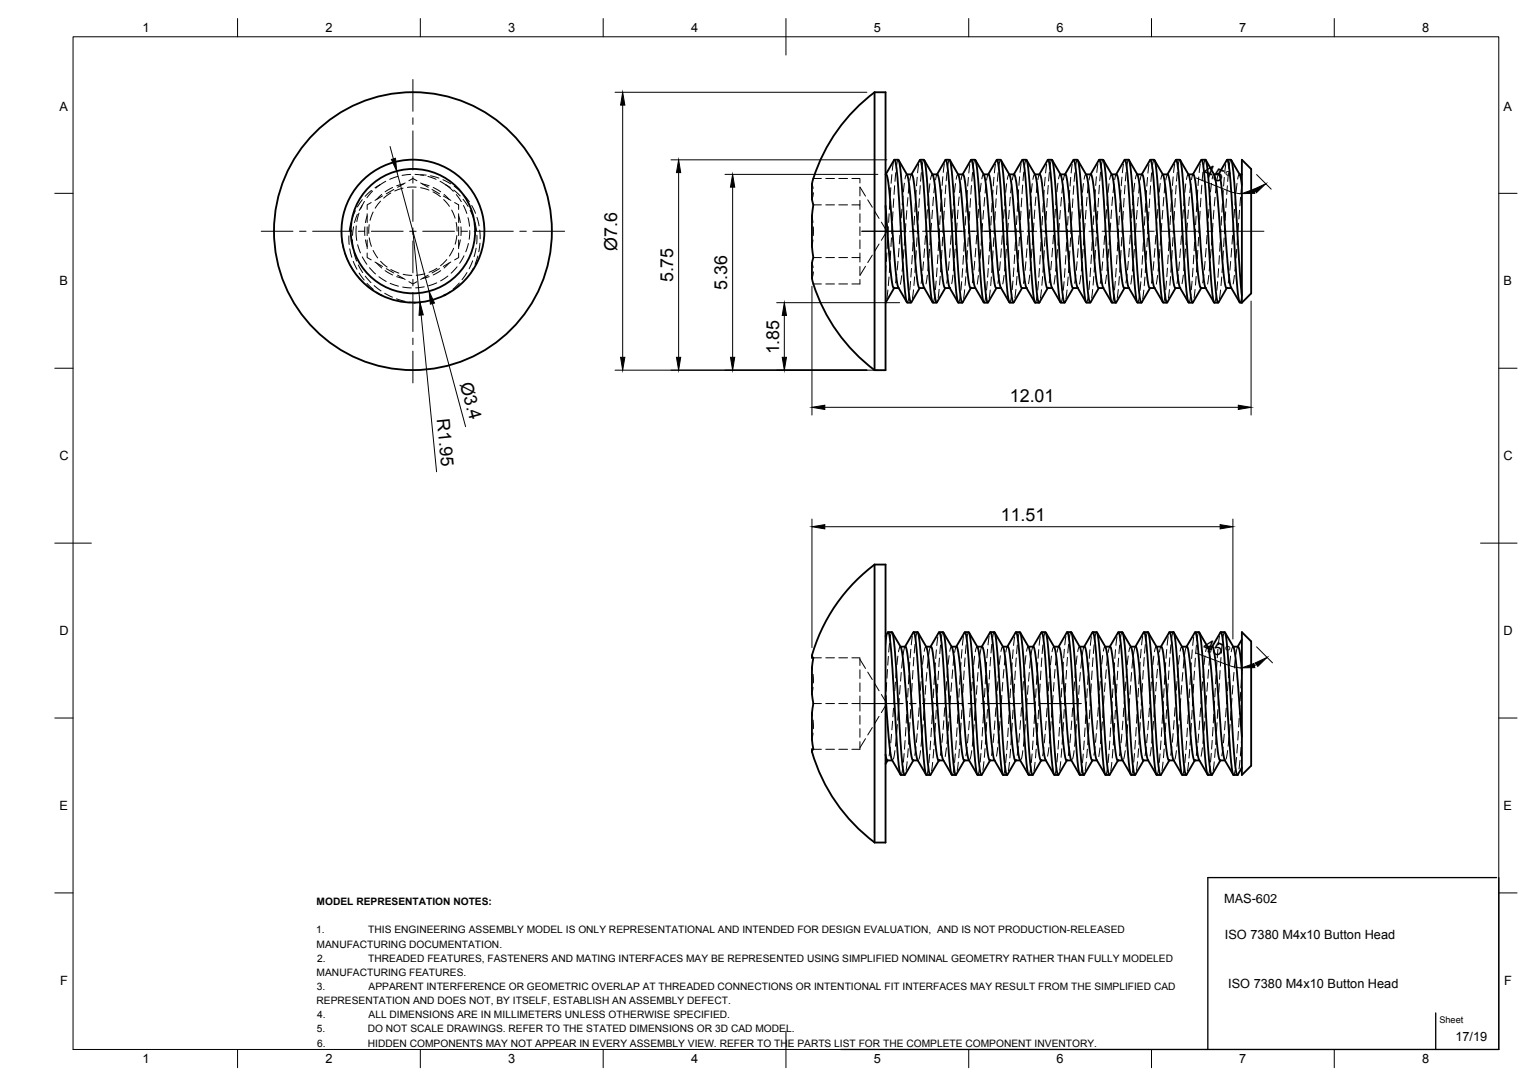
ISO-10303-21;
HEADER;
/* Generated by software containing ST-Developer
 * from STEP Tools, Inc. (www.steptools.com) 
 */

FILE_DESCRIPTION(
/* description */ (''),
/* implementation_level */ '2;1');

FILE_NAME(
/* name */ 'ISO 7380 M4x10 Button Head.step',
/* time_stamp */ '2026-10-15T14:42:47-07:00',
/* author */ (''),
/* organization */ (''),
/* preprocessor_version */ 'ST-DEVELOPER v20.2',
/* originating_system */ 'Autodesk Translation Framework v15.15.0.0',
/* authorisation */ '');

FILE_SCHEMA (('AUTOMOTIVE_DESIGN { 1 0 10303 214 3 1 1 }'));
ENDSEC;

DATA;
#10=MECHANICAL_DESIGN_GEOMETRIC_PRESENTATION_REPRESENTATION('',(#249),#85789);
#147=(
BOUNDED_CURVE()
B_SPLINE_CURVE(2,(#85443,#85444,#85445),.UNSPECIFIED.,.F.,.F.)
B_SPLINE_CURVE_WITH_KNOTS((3,3),(0.00911071066679689,0.0953350369275265),
 .UNSPECIFIED.)
CURVE()
GEOMETRIC_REPRESENTATION_ITEM()
RATIONAL_B_SPLINE_CURVE((1.01317087172823,1.0695397444443,1.01317087172823))
REPRESENTATION_ITEM('')
);
#148=(
BOUNDED_CURVE()
B_SPLINE_CURVE(2,(#85450,#85451,#85452),.UNSPECIFIED.,.F.,.F.)
B_SPLINE_CURVE_WITH_KNOTS((3,3),(0.00911071066679641,0.0953350369275264),
 .UNSPECIFIED.)
CURVE()
GEOMETRIC_REPRESENTATION_ITEM()
RATIONAL_B_SPLINE_CURVE((1.01317087172823,1.06953974444431,1.01317087172823))
REPRESENTATION_ITEM('')
);
#149=(
BOUNDED_CURVE()
B_SPLINE_CURVE(2,(#85457,#85458,#85459),.UNSPECIFIED.,.F.,.F.)
B_SPLINE_CURVE_WITH_KNOTS((3,3),(0.00911071066679675,0.0953350369275265),
 .UNSPECIFIED.)
CURVE()
GEOMETRIC_REPRESENTATION_ITEM()
RATIONAL_B_SPLINE_CURVE((1.01317087172823,1.0695397444443,1.01317087172823))
REPRESENTATION_ITEM('')
);
#150=(
BOUNDED_CURVE()
B_SPLINE_CURVE(2,(#85464,#85465,#85466),.UNSPECIFIED.,.F.,.F.)
B_SPLINE_CURVE_WITH_KNOTS((3,3),(0.00911071066679614,0.0953350369275257),
 .UNSPECIFIED.)
CURVE()
GEOMETRIC_REPRESENTATION_ITEM()
RATIONAL_B_SPLINE_CURVE((1.01317087172823,1.0695397444443,1.01317087172823))
REPRESENTATION_ITEM('')
);
#151=(
BOUNDED_CURVE()
B_SPLINE_CURVE(2,(#85471,#85472,#85473),.UNSPECIFIED.,.F.,.F.)
B_SPLINE_CURVE_WITH_KNOTS((3,3),(0.0091107106667967,0.0953350369275265),
 .UNSPECIFIED.)
CURVE()
GEOMETRIC_REPRESENTATION_ITEM()
RATIONAL_B_SPLINE_CURVE((1.01317087172823,1.0695397444443,1.01317087172823))
REPRESENTATION_ITEM('')
);
#152=(
BOUNDED_CURVE()
B_SPLINE_CURVE(2,(#85480,#85481,#85482),.UNSPECIFIED.,.F.,.F.)
B_SPLINE_CURVE_WITH_KNOTS((3,3),(0.00911071066679617,0.0953350369275259),
 .UNSPECIFIED.)
CURVE()
GEOMETRIC_REPRESENTATION_ITEM()
RATIONAL_B_SPLINE_CURVE((1.01317087172823,1.0695397444443,1.01317087172823))
REPRESENTATION_ITEM('')
);
#190=CONICAL_SURFACE('',#10812,0.185470053837925,1.0471975511966);
#191=CONICAL_SURFACE('',#10814,0.185470053837925,1.0471975511966);
#192=CONICAL_SURFACE('',#10816,0.185470053837925,1.0471975511966);
#193=CONICAL_SURFACE('',#10818,0.185470053837925,1.0471975511966);
#194=CONICAL_SURFACE('',#10820,0.185470053837925,1.0471975511966);
#195=CONICAL_SURFACE('',#10823,0.185470053837925,1.0471975511966);
#196=CONICAL_SURFACE('',#10840,0.06125,1.02376802452586);
#197=CONICAL_SURFACE('',#10851,0.185,0.785398163397448);
#213=SHAPE_REPRESENTATION_RELATIONSHIP('SRR','None',#85878,#231);
#231=ADVANCED_BREP_SHAPE_REPRESENTATION('',(#267),#85786);
#249=STYLED_ITEM('',(#85977),#267);
#267=MANIFOLD_SOLID_BREP('Body1',#9896);
#279=SPHERICAL_SURFACE('',#10825,0.475);
#384=B_SPLINE_SURFACE_WITH_KNOTS('',3,3,((#84473,#84474,#84475,#84476,#84477,
#84478,#84479,#84480,#84481,#84482,#84483,#84484,#84485,#84486,#84487,#84488,
#84489,#84490,#84491,#84492,#84493,#84494,#84495,#84496,#84497,#84498,#84499,
#84500,#84501,#84502,#84503,#84504,#84505,#84506,#84507,#84508,#84509,#84510,
#84511,#84512,#84513,#84514,#84515,#84516,#84517,#84518,#84519,#84520,#84521,
#84522,#84523,#84524,#84525,#84526,#84527,#84528,#84529,#84530,#84531,#84532,
#84533,#84534,#84535,#84536,#84537,#84538,#84539,#84540,#84541,#84542,#84543,
#84544,#84545,#84546,#84547,#84548,#84549,#84550,#84551,#84552,#84553,#84554,
#84555,#84556,#84557,#84558,#84559,#84560,#84561,#84562,#84563,#84564,#84565),
(#84566,#84567,#84568,#84569,#84570,#84571,#84572,#84573,#84574,#84575,
#84576,#84577,#84578,#84579,#84580,#84581,#84582,#84583,#84584,#84585,#84586,
#84587,#84588,#84589,#84590,#84591,#84592,#84593,#84594,#84595,#84596,#84597,
#84598,#84599,#84600,#84601,#84602,#84603,#84604,#84605,#84606,#84607,#84608,
#84609,#84610,#84611,#84612,#84613,#84614,#84615,#84616,#84617,#84618,#84619,
#84620,#84621,#84622,#84623,#84624,#84625,#84626,#84627,#84628,#84629,#84630,
#84631,#84632,#84633,#84634,#84635,#84636,#84637,#84638,#84639,#84640,#84641,
#84642,#84643,#84644,#84645,#84646,#84647,#84648,#84649,#84650,#84651,#84652,
#84653,#84654,#84655,#84656,#84657,#84658),(#84659,#84660,#84661,#84662,
#84663,#84664,#84665,#84666,#84667,#84668,#84669,#84670,#84671,#84672,#84673,
#84674,#84675,#84676,#84677,#84678,#84679,#84680,#84681,#84682,#84683,#84684,
#84685,#84686,#84687,#84688,#84689,#84690,#84691,#84692,#84693,#84694,#84695,
#84696,#84697,#84698,#84699,#84700,#84701,#84702,#84703,#84704,#84705,#84706,
#84707,#84708,#84709,#84710,#84711,#84712,#84713,#84714,#84715,#84716,#84717,
#84718,#84719,#84720,#84721,#84722,#84723,#84724,#84725,#84726,#84727,#84728,
#84729,#84730,#84731,#84732,#84733,#84734,#84735,#84736,#84737,#84738,#84739,
#84740,#84741,#84742,#84743,#84744,#84745,#84746,#84747,#84748,#84749,#84750,
#84751),(#84752,#84753,#84754,#84755,#84756,#84757,#84758,#84759,#84760,
#84761,#84762,#84763,#84764,#84765,#84766,#84767,#84768,#84769,#84770,#84771,
#84772,#84773,#84774,#84775,#84776,#84777,#84778,#84779,#84780,#84781,#84782,
#84783,#84784,#84785,#84786,#84787,#84788,#84789,#84790,#84791,#84792,#84793,
#84794,#84795,#84796,#84797,#84798,#84799,#84800,#84801,#84802,#84803,#84804,
#84805,#84806,#84807,#84808,#84809,#84810,#84811,#84812,#84813,#84814,#84815,
#84816,#84817,#84818,#84819,#84820,#84821,#84822,#84823,#84824,#84825,#84826,
#84827,#84828,#84829,#84830,#84831,#84832,#84833,#84834,#84835,#84836,#84837,
#84838,#84839,#84840,#84841,#84842,#84843,#84844)),.UNSPECIFIED.,.F.,.F.,
 .F.,(4,4),(4,1,1,1,1,1,1,1,1,1,1,1,1,1,1,1,1,1,1,1,1,1,1,1,1,1,1,1,1,1,
1,1,1,1,1,1,1,1,1,1,1,1,1,1,1,1,1,1,1,1,1,1,1,1,1,1,1,1,1,1,1,1,1,1,1,1,
1,1,1,1,1,1,1,1,1,1,1,1,1,1,1,1,1,1,1,1,1,1,1,1,4),(-0.000253204253161567,
0.04630431131317),(8.3105869227397,9.30553171793124,10.3004765131228,11.2954213083143,
12.2903661035059,13.2853108986974,14.2802556938889,15.2752004890805,16.270145284272,
17.2650900794635,18.2600348746551,19.2549796698466,20.2499244650382,21.2448692602297,
22.2398140554212,23.2347588506128,24.2297036458043,25.2246484409959,26.2195932361874,
27.2145380313789,28.2094828265705,29.204427621762,30.1993724169535,31.1943172121451,
32.1892620073366,33.1842068025282,34.1791515977197,35.1740963929112,36.1690411881028,
37.1639859832943,38.1589307784859,39.1538755736774,40.1488203688689,41.1437651640605,
42.138709959252,43.1336547544436,44.1285995496351,45.1235443448266,46.1184891400182,
47.1134339352097,48.1083787304012,49.1033235255928,50.0982683207843,51.0932131159759,
52.0881579111674,53.0831027063589,54.0780475015505,55.072992296742,56.0679370919336,
57.0628818871251,58.0578266823166,59.0527714775082,60.0477162726997,61.0426610678912,
62.0376058630828,63.0325506582743,64.0274954534659,65.0224402486574,66.0173850438489,
67.0123298390405,68.007274634232,69.0022194294236,69.9971642246151,70.9921090198066,
71.9870538149982,72.9819986101897,73.9769434053812,74.9718882005728,75.9668329957643,
76.9617777909559,77.9567225861474,78.951667381339,79.9466121765305,80.941556971722,
81.9365017669136,82.9314465621051,83.9263913572966,84.9213361524882,85.9162809476797,
86.9112257428713,87.9061705380628,88.9011153332543,89.8960601284459,90.8910049236374,
91.885949718829,92.8808945140205,93.875839309212,94.8707841044036,95.8657288995951,
96.8606736947866,97.8556184899782),.UNSPECIFIED.);
#385=B_SPLINE_SURFACE_WITH_KNOTS('',3,3,((#85012,#85013,#85014,#85015,#85016,
#85017,#85018,#85019,#85020,#85021,#85022,#85023,#85024,#85025,#85026,#85027,
#85028,#85029,#85030,#85031,#85032,#85033,#85034,#85035,#85036,#85037,#85038,
#85039,#85040,#85041,#85042,#85043,#85044,#85045,#85046,#85047,#85048,#85049,
#85050,#85051,#85052,#85053,#85054,#85055,#85056,#85057,#85058,#85059,#85060,
#85061,#85062,#85063,#85064,#85065,#85066,#85067,#85068,#85069,#85070,#85071,
#85072,#85073,#85074,#85075,#85076,#85077,#85078,#85079,#85080,#85081,#85082,
#85083,#85084,#85085,#85086,#85087,#85088,#85089,#85090,#85091,#85092,#85093,
#85094,#85095,#85096,#85097,#85098,#85099,#85100,#85101,#85102,#85103,#85104),
(#85105,#85106,#85107,#85108,#85109,#85110,#85111,#85112,#85113,#85114,
#85115,#85116,#85117,#85118,#85119,#85120,#85121,#85122,#85123,#85124,#85125,
#85126,#85127,#85128,#85129,#85130,#85131,#85132,#85133,#85134,#85135,#85136,
#85137,#85138,#85139,#85140,#85141,#85142,#85143,#85144,#85145,#85146,#85147,
#85148,#85149,#85150,#85151,#85152,#85153,#85154,#85155,#85156,#85157,#85158,
#85159,#85160,#85161,#85162,#85163,#85164,#85165,#85166,#85167,#85168,#85169,
#85170,#85171,#85172,#85173,#85174,#85175,#85176,#85177,#85178,#85179,#85180,
#85181,#85182,#85183,#85184,#85185,#85186,#85187,#85188,#85189,#85190,#85191,
#85192,#85193,#85194,#85195,#85196,#85197),(#85198,#85199,#85200,#85201,
#85202,#85203,#85204,#85205,#85206,#85207,#85208,#85209,#85210,#85211,#85212,
#85213,#85214,#85215,#85216,#85217,#85218,#85219,#85220,#85221,#85222,#85223,
#85224,#85225,#85226,#85227,#85228,#85229,#85230,#85231,#85232,#85233,#85234,
#85235,#85236,#85237,#85238,#85239,#85240,#85241,#85242,#85243,#85244,#85245,
#85246,#85247,#85248,#85249,#85250,#85251,#85252,#85253,#85254,#85255,#85256,
#85257,#85258,#85259,#85260,#85261,#85262,#85263,#85264,#85265,#85266,#85267,
#85268,#85269,#85270,#85271,#85272,#85273,#85274,#85275,#85276,#85277,#85278,
#85279,#85280,#85281,#85282,#85283,#85284,#85285,#85286,#85287,#85288,#85289,
#85290),(#85291,#85292,#85293,#85294,#85295,#85296,#85297,#85298,#85299,
#85300,#85301,#85302,#85303,#85304,#85305,#85306,#85307,#85308,#85309,#85310,
#85311,#85312,#85313,#85314,#85315,#85316,#85317,#85318,#85319,#85320,#85321,
#85322,#85323,#85324,#85325,#85326,#85327,#85328,#85329,#85330,#85331,#85332,
#85333,#85334,#85335,#85336,#85337,#85338,#85339,#85340,#85341,#85342,#85343,
#85344,#85345,#85346,#85347,#85348,#85349,#85350,#85351,#85352,#85353,#85354,
#85355,#85356,#85357,#85358,#85359,#85360,#85361,#85362,#85363,#85364,#85365,
#85366,#85367,#85368,#85369,#85370,#85371,#85372,#85373,#85374,#85375,#85376,
#85377,#85378,#85379,#85380,#85381,#85382,#85383)),.UNSPECIFIED.,.F.,.F.,
 .F.,(4,4),(4,1,1,1,1,1,1,1,1,1,1,1,1,1,1,1,1,1,1,1,1,1,1,1,1,1,1,1,1,1,
1,1,1,1,1,1,1,1,1,1,1,1,1,1,1,1,1,1,1,1,1,1,1,1,1,1,1,1,1,1,1,1,1,1,1,1,
1,1,1,1,1,1,1,1,1,1,1,1,1,1,1,1,1,1,1,1,1,1,1,1,4),(-0.000274284936597264,
0.0463311323873803),(11.6151052031776,12.6103663143021,13.6053111094936,
14.6002559046852,15.5952006998767,16.5901454950682,17.5850902902598,18.5800350854513,
19.5749798806429,20.5699246758344,21.5648694710259,22.5598142662175,23.554759061409,
24.5497038566006,25.5446486517921,26.5395934469836,27.5345382421752,28.5294830373667,
29.5244278325583,30.5193726277498,31.5143174229413,32.5092622181329,33.5042070133244,
34.4991518085159,35.4940966037075,36.489041398899,37.4839861940906,38.4789309892821,
39.4738757844736,40.4688205796652,41.4637653748567,42.4587101700483,43.4536549652398,
44.4485997604313,45.4435445556229,46.4384893508144,47.433434146006,48.4283789411975,
49.423323736389,50.4182685315806,51.4132133267721,52.4081581219637,53.4031029171552,
54.3980477123467,55.3929925075383,56.3879373027298,57.3828820979213,58.3778268931129,
59.3727716883044,60.367716483496,61.3626612786875,62.357606073879,63.3525508690706,
64.3474956642621,65.3424404594537,66.3373852546452,67.3323300498367,68.3272748450283,
69.3222196402198,70.3171644354113,71.3121092306029,72.3070540257944,73.301998820986,
74.2969436161775,75.291888411369,76.2868332065606,77.2817780017521,78.2767227969437,
79.2716675921352,80.2666123873267,81.2615571825183,82.2565019777098,83.2514467729014,
84.2463915680929,85.2413363632844,86.236281158476,87.2312259536675,88.226170748859,
89.2211155440506,90.2160603392421,91.2110051344337,92.2059499296252,93.2008947248167,
94.1958395200083,95.1907843151998,96.1857291103914,97.1806739055829,98.1756187007744,
99.170563495966,100.165508291158,101.160453086349),.UNSPECIFIED.);
#473=FACE_BOUND('',#3455,.T.);
#474=FACE_BOUND('',#3459,.T.);
#908=B_SPLINE_CURVE_WITH_KNOTS('',3,(#77896,#77897,#77898,#77899,#77900,
#77901,#77902,#77903,#77904,#77905,#77906,#77907,#77908,#77909,#77910,#77911,
#77912,#77913,#77914,#77915,#77916,#77917,#77918,#77919,#77920,#77921,#77922,
#77923,#77924,#77925,#77926,#77927,#77928,#77929,#77930,#77931,#77932,#77933,
#77934,#77935,#77936,#77937,#77938,#77939,#77940,#77941,#77942,#77943,#77944),
 .UNSPECIFIED.,.F.,.F.,(4,3,3,3,3,3,3,3,3,3,3,3,3,3,3,3,4),(10.3761261730577,
10.5727849197489,10.7692055827359,10.9654664845638,11.1621727918026,11.2954213083143,
11.494377948575,11.6933749873077,11.8919022657422,12.0911341846241,12.2903661035059,
12.4887047013559,12.6878562506913,12.8857302559588,13.0855205773281,13.2853108986974,
13.4195932955372),.UNSPECIFIED.);
#909=B_SPLINE_CURVE_WITH_KNOTS('',3,(#77947,#77948,#77949,#77950,#77951,
#77952,#77953,#77954,#77955,#77956,#77957,#77958,#77959,#77960,#77961,#77962,
#77963,#77964,#77965,#77966,#77967,#77968,#77969,#77970,#77971,#77972,#77973,
#77974),.UNSPECIFIED.,.F.,.F.,(4,3,3,3,3,3,3,3,3,4),(11.6154215191106,11.818758087608,
12.02219938105,12.2256382911152,12.4297226410097,12.6103663143021,12.8124062223988,
13.0085336172549,13.213529781972,13.418525946689),.UNSPECIFIED.);
#910=B_SPLINE_CURVE_WITH_KNOTS('',3,(#77980,#77981,#77982,#77983,#77984,
#77985,#77986,#77987,#77988,#77989,#77990,#77991,#77992,#77993,#77994,#77995,
#77996,#77997,#77998,#77999,#78000,#78001,#78002,#78003,#78004,#78005,#78006,
#78007,#78008,#78009,#78010,#78011,#78012,#78013,#78014,#78015,#78016,#78017,
#78018,#78019,#78020,#78021,#78022,#78023,#78024,#78025,#78026,#78027,#78028,
#78029,#78030,#78031,#78032,#78033,#78034,#78035,#78036,#78037,#78038,#78039,
#78040,#78041,#78042,#78043),.UNSPECIFIED.,.F.,.F.,(4,3,3,3,3,3,3,3,3,3,
3,3,3,3,3,3,3,3,3,3,3,4),(15.7079632679489,15.9107481580219,16.1142494687792,
16.270145284272,16.4687682481423,16.6678487059726,16.8660184761811,17.0655542778223,
17.2650900794635,17.463705654094,17.6627879592342,17.8609505715831,18.0604927231191,
18.2600348746551,18.4586404264755,18.6577252373183,18.8558771547285,19.0554284122876,
19.2549796698466,19.4536004000213,19.6518004795038,19.7024262307223),
 .UNSPECIFIED.);
#911=B_SPLINE_CURVE_WITH_KNOTS('',3,(#78044,#78045,#78046,#78047,#78048,
#78049,#78050,#78051,#78052,#78053,#78054,#78055,#78056,#78057,#78058,#78059,
#78060,#78061,#78062,#78063,#78064,#78065,#78066,#78067,#78068,#78069,#78070,
#78071,#78072,#78073,#78074,#78075,#78076,#78077,#78078,#78079,#78080),
 .UNSPECIFIED.,.F.,.F.,(4,3,3,3,3,3,3,3,3,3,3,3,4),(13.4195932955372,13.6179476079485,
13.816207268142,14.0144158621728,14.2130841295482,14.2802556938889,14.4789073498003,
14.6779806346204,14.8761820439794,15.0756912665299,15.2752004890805,15.4915818782546,
15.7079632674287),.UNSPECIFIED.);
#912=B_SPLINE_CURVE_WITH_KNOTS('',3,(#78082,#78083,#78084,#78085,#78086,
#78087,#78088,#78089,#78090,#78091,#78092,#78093,#78094,#78095,#78096,#78097,
#78098,#78099,#78100,#78101,#78102,#78103,#78104,#78105,#78106,#78107,#78108,
#78109,#78110,#78111,#78112,#78113,#78114,#78115,#78116,#78117,#78118),
 .UNSPECIFIED.,.F.,.F.,(4,3,3,3,3,3,3,3,3,3,3,3,4),(13.418525946689,13.6053111094936,
13.8042318364677,14.003237853522,14.2017004757908,14.400978190238,14.6002559046852,
14.7992124415244,14.9982095061125,15.1967366702124,15.3959686850445,15.5952006998767,
15.7079632679489),.UNSPECIFIED.);
#913=B_SPLINE_CURVE_WITH_KNOTS('',3,(#78119,#78120,#78121,#78122,#78123,
#78124,#78125,#78126,#78127,#78128,#78129,#78130,#78131,#78132,#78133,#78134,
#78135,#78136,#78137,#78138,#78139,#78140,#78141,#78142,#78143,#78144,#78145,
#78146,#78147,#78148,#78149,#78150,#78151,#78152,#78153,#78154,#78155,#78156,
#78157,#78158,#78159,#78160,#78161,#78162,#78163,#78164,#78165,#78166,#78167,
#78168,#78169,#78170,#78171,#78172,#78173,#78174,#78175,#78176,#78177,#78178,
#78179,#78180,#78181,#78182,#78183,#78184,#78185,#78186,#78187,#78188,#78189,
#78190,#78191,#78192,#78193,#78194,#78195,#78196,#78197,#78198,#78199,#78200,
#78201,#78202,#78203,#78204,#78205,#78206,#78207,#78208,#78209,#78210,#78211,
#78212,#78213,#78214,#78215,#78216,#78217,#78218,#78219,#78220,#78221,#78222,
#78223,#78224,#78225,#78226,#78227,#78228,#78229,#78230,#78231,#78232,#78233,
#78234,#78235,#78236,#78237,#78238,#78239,#78240,#78241,#78242),
 .UNSPECIFIED.,.F.,.F.,(4,2,2,2,2,2,2,2,2,2,2,2,2,2,2,2,2,2,2,2,2,2,2,2,
2,2,2,2,2,2,2,2,2,2,2,2,2,2,2,2,2,2,2,2,2,2,2,2,2,2,2,2,2,2,2,2,2,2,2,2,
2,4),(-1.96103056545371,-1.92615510476781,-1.90994104798314,-1.9046916544681,
-1.90116335747262,-1.89772121026667,-1.89353123364095,-1.8830555785659,
-1.84636429336028,-1.83469395897624,-1.82971190344123,-1.82587053879483,
-1.82382632031197,-1.82191411745611,-1.81939311968034,-1.81356733650211,
-1.77965416666506,-1.76360355394232,-1.75280328971649,-1.74820347743362,
-1.74476514754024,-1.74105759432205,-1.73505605688044,-1.70682592759978,
-1.6841639181994,-1.67334525175968,-1.67015445276645,-1.66812211217972,
-1.66633132628009,-1.66333921335296,-1.65504429895045,-1.62400305204443,
-1.60514022362692,-1.59676356512943,-1.59258448468083,-1.58919905483207,
-1.5852684928244,-1.57835914547407,-1.54422662487699,-1.52704989903113,
-1.51777093811399,-1.51474603772319,-1.51275491824691,-1.51094365904601,
-1.50782252160796,-1.49846413471266,-1.47181634411575,-1.44773006870327,
-1.44064466762602,-1.43672150260578,-1.43334093274202,-1.42916612578598,
-1.42263789249716,-1.39594967959925,-1.37360499022705,-1.3663301636072,
-1.3611348244643,-1.35870036542346,-1.35679264787092,-1.35442699301585,
-1.34960688579188,-1.33784917433159),.UNSPECIFIED.);
#914=B_SPLINE_CURVE_WITH_KNOTS('',3,(#78248,#78249,#78250,#78251,#78252,
#78253,#78254,#78255,#78256,#78257,#78258,#78259,#78260,#78261,#78262,#78263,
#78264,#78265,#78266,#78267,#78268,#78269,#78270,#78271,#78272,#78273,#78274,
#78275,#78276,#78277,#78278,#78279,#78280,#78281,#78282,#78283,#78284,#78285,
#78286,#78287,#78288,#78289,#78290,#78291,#78292,#78293,#78294,#78295,#78296,
#78297,#78298,#78299,#78300,#78301,#78302,#78303,#78304,#78305,#78306,#78307,
#78308),.UNSPECIFIED.,.F.,.F.,(4,3,3,3,3,3,3,3,3,3,3,3,3,3,3,3,3,3,3,3,
4),(21.991148575456,22.2398140554212,22.4384256549512,22.6375089538666,
22.8356672026196,23.0352130266162,23.2347588506128,23.4333701243398,23.6324535047059,
23.8306114233726,24.0301575345884,24.2297036458043,24.4283147914976,24.6273982038722,
24.8255559829737,25.0251022119848,25.2246484409959,25.4232904579861,25.6215093722145,
25.8197872076773,25.9848803801132),.UNSPECIFIED.);
#915=B_SPLINE_CURVE_WITH_KNOTS('',3,(#78309,#78310,#78311,#78312,#78313,
#78314,#78315,#78316,#78317,#78318,#78319,#78320,#78321,#78322,#78323,#78324,
#78325,#78326,#78327,#78328,#78329,#78330,#78331,#78332,#78333,#78334,#78335,
#78336,#78337,#78338,#78339,#78340,#78341,#78342,#78343,#78344,#78345),
 .UNSPECIFIED.,.F.,.F.,(4,3,3,3,3,3,3,3,3,3,3,3,4),(19.7024262307223,19.9005709735403,
20.0991973388965,20.2499244650382,20.4485361071857,20.6476193954467,20.845777725713,
21.0453234929714,21.2448692602297,21.4412420479956,21.6371996234507,21.8332504102883,
21.9911485751285),.UNSPECIFIED.);
#916=B_SPLINE_CURVE_WITH_KNOTS('',3,(#78346,#78347,#78348,#78349,#78350,
#78351,#78352,#78353,#78354,#78355,#78356,#78357,#78358,#78359,#78360,#78361,
#78362,#78363,#78364,#78365,#78366,#78367,#78368,#78369,#78370,#78371,#78372,
#78373,#78374,#78375,#78376,#78377,#78378,#78379,#78380,#78381,#78382,#78383,
#78384,#78385,#78386,#78387,#78388,#78389,#78390,#78391,#78392,#78393,#78394,
#78395,#78396,#78397,#78398,#78399,#78400,#78401,#78402,#78403,#78404,#78405,
#78406,#78407,#78408,#78409,#78410,#78411,#78412,#78413,#78414,#78415,#78416,
#78417,#78418,#78419,#78420,#78421,#78422,#78423,#78424,#78425,#78426,#78427,
#78428,#78429,#78430,#78431,#78432,#78433,#78434,#78435,#78436,#78437,#78438,
#78439,#78440,#78441,#78442,#78443,#78444,#78445,#78446,#78447,#78448,#78449,
#78450,#78451,#78452,#78453,#78454,#78455,#78456,#78457,#78458,#78459,#78460,
#78461,#78462,#78463,#78464,#78465,#78466,#78467,#78468,#78469,#78470,#78471,
#78472,#78473,#78474,#78475,#78476,#78477,#78478,#78479,#78480,#78481,#78482,
#78483,#78484,#78485,#78486,#78487,#78488,#78489,#78490,#78491,#78492,#78493,
#78494,#78495,#78496,#78497,#78498,#78499,#78500,#78501,#78502,#78503,#78504,
#78505,#78506,#78507,#78508,#78509,#78510,#78511,#78512,#78513,#78514,#78515,
#78516,#78517,#78518,#78519,#78520,#78521,#78522,#78523,#78524,#78525,#78526,
#78527,#78528,#78529,#78530,#78531,#78532,#78533,#78534,#78535),
 .UNSPECIFIED.,.F.,.F.,(4,2,2,2,2,2,2,2,2,2,2,2,2,2,2,2,2,2,2,2,2,2,2,2,
2,2,2,2,2,2,2,2,2,2,2,2,2,2,2,2,2,2,2,2,2,2,2,2,2,2,2,2,2,2,2,2,2,2,2,2,
2,2,2,2,2,2,2,2,2,2,2,2,2,2,2,2,2,2,2,2,2,2,2,2,2,2,2,2,2,2,2,2,2,2,4),
(-1.33784917433159,-1.32756271885982,-1.30746809628493,-1.28939857659663,
-1.28395387447302,-1.28036685748039,-1.27691930054231,-1.2727846053549,
-1.26276650569296,-1.22575346202038,-1.21407469874287,-1.20681188390887,
-1.20403977707747,-1.20209398347381,-1.19993728032837,-1.19614402680512,
-1.1729430995681,-1.15449759215625,-1.14117856246438,-1.13168731495249,
-1.12730885836149,-1.12390720854947,-1.12011025153647,-1.11365057866505,
-1.07528746513936,-1.0553370235293,-1.05052825197158,-1.04816492281006,
-1.04644637863359,-1.04410710587933,-1.03942200525473,-1.01275043165541,
-0.980829421102169,-0.974447844548088,-0.970667458066885,-0.9672627866578,
-0.962855203362212,-0.953192246538504,-0.939528089692697,-0.921336843879064,
-0.898406338458633,-0.894624793607861,-0.89247094204319,-0.890525409423738,
-0.887750286363114,-0.880459212620312,-0.868713363789876,-0.831175749903035,
-0.822319674972369,-0.817511683875312,-0.814081167966399,-0.810469415682009,
-0.804899683798356,-0.78523918108987,-0.766557014422738,-0.744919619905274,
-0.740103169427347,-0.737738155416985,-0.735829107829343,-0.733390517868837,
-0.728181935370119,-0.720884753609942,-0.69840605593486,-0.671982171455758,
-0.665440679358723,-0.661259612770394,-0.657875180711825,-0.653948729818894,
-0.646860388854981,-0.622776219453138,-0.596138296662889,-0.586737876282968,
-0.58360986965392,-0.581796092624829,-0.579804634036784,-0.576781103437763,
-0.567518514649867,-0.5503895920759,-0.516283668413562,-0.509384121107263,
-0.505456557571469,-0.502072217283729,-0.497892614783625,-0.489508899082389,
-0.470574667497139,-0.439334079795521,-0.431182458349704,-0.428211654249095,
-0.426426865138206,-0.424400132297633,-0.421208225679968,-0.410292686384152,
-0.387244928865465,-0.359349102730245,-0.35767490124526),.UNSPECIFIED.);
#917=B_SPLINE_CURVE_WITH_KNOTS('',3,(#78541,#78542,#78543,#78544,#78545,
#78546,#78547,#78548,#78549,#78550,#78551,#78552,#78553,#78554,#78555,#78556,
#78557,#78558,#78559,#78560,#78561,#78562,#78563,#78564,#78565,#78566,#78567,
#78568,#78569,#78570,#78571,#78572,#78573,#78574,#78575,#78576,#78577,#78578,
#78579,#78580,#78581,#78582,#78583,#78584,#78585,#78586,#78587,#78588,#78589,
#78590,#78591,#78592,#78593,#78594,#78595,#78596,#78597,#78598,#78599,#78600,
#78601,#78602,#78603,#78604),.UNSPECIFIED.,.F.,.F.,(4,3,3,3,3,3,3,3,3,3,
3,3,3,3,3,3,3,3,3,3,3,4),(28.2743338827622,28.471046494824,28.667522646786,
28.8638355561955,29.0606093893357,29.204427621762,29.4030388737554,29.602122259555,
29.8002801509351,29.9998262839443,30.1993724169535,30.3979836682494,30.5970670542233,
30.7952249447415,30.9947710784433,31.1943172121451,31.3929284665306,31.5920118517321,
31.7901697455092,31.9897158764229,32.1892620073366,32.2690227615599),
 .UNSPECIFIED.);
#918=B_SPLINE_CURVE_WITH_KNOTS('',3,(#78605,#78606,#78607,#78608,#78609,
#78610,#78611,#78612,#78613,#78614,#78615,#78616,#78617,#78618,#78619,#78620,
#78621,#78622,#78623,#78624,#78625,#78626,#78627,#78628,#78629,#78630,#78631,
#78632,#78633,#78634,#78635,#78636,#78637,#78638,#78639,#78640,#78641,#78642,
#78643,#78644),.UNSPECIFIED.,.F.,.F.,(4,3,3,3,3,3,3,3,3,3,3,3,3,4),(25.9848803801132,
26.1834953229633,26.2195932361874,26.4182044870052,26.6172878730986,26.8154457638341,
27.0149918976065,27.2145380313789,27.4131492703702,27.6122326594203,27.8103905369092,
28.0099366817399,28.2094828265705,28.2743338823081),.UNSPECIFIED.);
#919=B_SPLINE_CURVE_WITH_KNOTS('',3,(#78646,#78647,#78648,#78649,#78650,
#78651,#78652,#78653,#78654,#78655,#78656,#78657,#78658,#78659,#78660,#78661,
#78662,#78663,#78664,#78665,#78666,#78667,#78668,#78669,#78670,#78671,#78672,
#78673,#78674,#78675,#78676,#78677,#78678,#78679,#78680,#78681,#78682,#78683,
#78684,#78685,#78686,#78687,#78688,#78689,#78690,#78691,#78692,#78693,#78694,
#78695,#78696,#78697,#78698,#78699,#78700,#78701,#78702,#78703,#78704,#78705,
#78706,#78707,#78708,#78709,#78710,#78711,#78712,#78713,#78714,#78715,#78716,
#78717,#78718,#78719,#78720,#78721,#78722,#78723),.UNSPECIFIED.,.F.,.F.,
(4,2,2,2,2,2,2,2,2,2,2,2,2,2,2,2,2,2,2,2,2,2,2,2,2,2,2,2,2,2,2,2,2,2,2,
2,2,2,4),(-0.35767490124526,-0.353305421574032,-0.349595255689124,-0.346170349734198,
-0.341613025527349,-0.331039317409103,-0.315467840449632,-0.284630569162204,
-0.276082485707659,-0.273059191968105,-0.271264872944148,-0.26925104854512,
-0.266119814035009,-0.255837730626168,-0.235260851599245,-0.206256226033263,
-0.199755621329898,-0.195586231881908,-0.192202201704497,-0.188266060712361,
-0.181130922108284,-0.156680755239567,-0.129309790545012,-0.12084135672295,
-0.117828378943232,-0.116035930774091,-0.114019618232537,-0.111292342370151,
-0.10519671203938,-0.102721920333533,-0.0876272756893066,-0.058692799791427,
-0.0465427107185492,-0.0416200658294285,-0.0381695350916806,-0.0345894279611084,
-0.0309667648357375,-0.0258029228333309,-0.000454559668527777),
 .UNSPECIFIED.);
#920=B_SPLINE_CURVE_WITH_KNOTS('',3,(#78724,#78725,#78726,#78727,#78728,
#78729,#78730,#78731,#78732,#78733,#78734,#78735,#78736,#78737,#78738,#78739,
#78740,#78741,#78742,#78743,#78744,#78745,#78746,#78747,#78748,#78749,#78750,
#78751,#78752,#78753,#78754,#78755,#78756,#78757,#78758,#78759,#78760,#78761,
#78762,#78763,#78764,#78765,#78766,#78767,#78768,#78769,#78770,#78771,#78772,
#78773,#78774,#78775,#78776,#78777,#78778,#78779,#78780,#78781,#78782,#78783,
#78784,#78785,#78786,#78787,#78788,#78789,#78790,#78791,#78792,#78793,#78794,
#78795,#78796,#78797,#78798,#78799,#78800,#78801,#78802,#78803,#78804,#78805,
#78806,#78807,#78808,#78809,#78810,#78811,#78812,#78813,#78814,#78815,#78816,
#78817,#78818,#78819,#78820,#78821,#78822,#78823,#78824,#78825,#78826,#78827,
#78828,#78829,#78830,#78831,#78832,#78833,#78834,#78835,#78836,#78837,#78838,
#78839,#78840,#78841,#78842,#78843,#78844,#78845,#78846,#78847,#78848,#78849,
#78850,#78851,#78852,#78853,#78854,#78855,#78856,#78857),.UNSPECIFIED.,
 .F.,.F.,(4,2,2,2,2,2,2,2,2,2,2,2,2,2,2,2,2,2,2,2,2,2,2,2,2,2,2,2,2,2,2,
2,2,2,2,2,2,2,2,2,2,2,2,2,2,2,2,2,2,2,2,2,2,2,2,2,2,2,2,2,2,2,2,2,2,2,4),
(-1.96074742950682,-1.92903103891679,-1.92565394037489,-1.92276149113017,
-1.92079576416029,-1.91868782038145,-1.91511919124233,-1.9004272637792,
-1.87491209959576,-1.85410453753753,-1.84813467188929,-1.8479163875349,
-1.84770085619269,-1.84748534465099,-1.84726696921916,-1.8470425292415,
-1.84680828683192,-1.84655965391311,-1.8462907190531,-1.84285619153888,
-1.83917562130058,-1.83327062379081,-1.80958144579062,-1.78819556450568,
-1.77185176006219,-1.76828771149167,-1.76618076264445,-1.76423727298914,
-1.76136039858266,-1.75390897523033,-1.72574504428177,-1.70091214406183,
-1.69373013799826,-1.68978518091811,-1.68640266589147,-1.68224669189248,
-1.67579014886227,-1.64469048785606,-1.62559436177049,-1.61890027333474,
-1.61401473550339,-1.61163686591323,-1.60991777261583,-1.60759235705981,
-1.60311921587875,-1.56755879210728,-1.54516146622278,-1.53829655404521,
-1.53441625718776,-1.53102828603607,-1.52678609995889,-1.52003079834842,
-1.4794373383665,-1.46156592197152,-1.45793400775734,-1.45581228428364,
-1.45387566523685,-1.45103839222197,-1.44383935846247,-1.41163093054835,
-1.39220114476349,-1.38398165704351,-1.37983323323713,-1.3764507990235,
-1.37249905929152,-1.36548575233231,-1.33781741101813),.UNSPECIFIED.);
#921=B_SPLINE_CURVE_WITH_KNOTS('',3,(#78863,#78864,#78865,#78866,#78867,
#78868,#78869,#78870,#78871,#78872,#78873,#78874,#78875,#78876,#78877,#78878,
#78879,#78880,#78881,#78882,#78883,#78884,#78885,#78886,#78887,#78888,#78889,
#78890,#78891,#78892,#78893,#78894,#78895,#78896,#78897,#78898,#78899,#78900,
#78901,#78902,#78903,#78904,#78905,#78906,#78907,#78908,#78909,#78910,#78911,
#78912,#78913,#78914,#78915,#78916,#78917,#78918,#78919,#78920,#78921,#78922,
#78923),.UNSPECIFIED.,.F.,.F.,(4,3,3,3,3,3,3,3,3,3,3,3,3,3,3,3,3,3,3,3,
4),(34.5575191894876,34.7574162785789,34.9657563357451,35.1740963929112,
35.3727076459311,35.571791031474,35.7699489238318,35.9694950559673,36.1690411881028,
36.3676524411512,36.566735826687,36.7648937190718,36.9644398511831,37.1639859832943,
37.3625972363943,37.5616806219172,37.7598385143569,37.9593846464214,38.1589307784859,
38.3575822166857,38.5521360709588),.UNSPECIFIED.);
#922=B_SPLINE_CURVE_WITH_KNOTS('',3,(#78924,#78925,#78926,#78927,#78928,
#78929,#78930,#78931,#78932,#78933,#78934,#78935,#78936,#78937,#78938,#78939,
#78940,#78941,#78942,#78943,#78944,#78945,#78946,#78947,#78948,#78949,#78950,
#78951,#78952,#78953,#78954,#78955,#78956,#78957,#78958,#78959,#78960),
 .UNSPECIFIED.,.F.,.F.,(4,3,3,3,3,3,3,3,3,3,3,3,4),(32.2690227615599,32.4674315365707,
32.6656817064457,32.8638217074933,33.0624351927568,33.1842068025282,33.3828180553875,
33.5819014409705,33.7800593331526,33.9796054654362,34.1791515977197,34.4020312303527,
34.5575191891138),.UNSPECIFIED.);
#923=B_SPLINE_CURVE_WITH_KNOTS('',3,(#78961,#78962,#78963,#78964,#78965,
#78966,#78967,#78968,#78969,#78970,#78971,#78972,#78973,#78974,#78975,#78976,
#78977,#78978,#78979,#78980,#78981,#78982,#78983,#78984,#78985,#78986,#78987,
#78988,#78989,#78990,#78991,#78992,#78993,#78994,#78995,#78996,#78997,#78998,
#78999,#79000,#79001,#79002,#79003,#79004,#79005,#79006,#79007,#79008,#79009,
#79010,#79011,#79012,#79013,#79014,#79015,#79016,#79017,#79018,#79019,#79020,
#79021,#79022,#79023,#79024,#79025,#79026,#79027,#79028,#79029,#79030,#79031,
#79032,#79033,#79034,#79035,#79036,#79037,#79038,#79039,#79040,#79041,#79042,
#79043,#79044,#79045,#79046,#79047,#79048,#79049,#79050,#79051,#79052,#79053,
#79054,#79055,#79056,#79057,#79058,#79059,#79060,#79061,#79062,#79063,#79064,
#79065,#79066,#79067,#79068,#79069,#79070,#79071,#79072,#79073,#79074,#79075,
#79076,#79077,#79078,#79079,#79080,#79081,#79082,#79083,#79084,#79085,#79086,
#79087,#79088,#79089,#79090,#79091,#79092,#79093,#79094,#79095,#79096,#79097,
#79098,#79099,#79100,#79101,#79102,#79103,#79104,#79105,#79106,#79107,#79108,
#79109,#79110,#79111,#79112,#79113,#79114,#79115,#79116,#79117,#79118,#79119,
#79120,#79121,#79122,#79123,#79124,#79125,#79126,#79127,#79128,#79129,#79130,
#79131,#79132,#79133,#79134,#79135,#79136,#79137,#79138,#79139,#79140,#79141,
#79142,#79143,#79144,#79145,#79146,#79147,#79148,#79149,#79150,#79151,#79152,
#79153,#79154),.UNSPECIFIED.,.F.,.F.,(4,2,2,2,2,2,2,2,2,2,2,2,2,2,2,2,2,
2,2,2,2,2,2,2,2,2,2,2,2,2,2,2,2,2,2,2,2,2,2,2,2,2,2,2,2,2,2,2,2,2,2,2,2,
2,2,2,2,2,2,2,2,2,2,2,2,2,2,2,2,2,2,2,2,2,2,2,2,2,2,2,2,2,2,2,2,2,2,2,2,
2,2,2,2,2,2,2,4),(-1.33781741101813,-1.32557054748569,-1.30642325762965,
-1.30274443726903,-1.3006124784046,-1.29868008249966,-1.29586834752457,
-1.28882936678198,-1.25644145308868,-1.24063435784198,-1.22995239379204,
-1.22537824600346,-1.22195104437654,-1.21824825123111,-1.21223927049898,
-1.18597264853726,-1.16660703127076,-1.15094181272081,-1.1474117560645,
-1.14531188838297,-1.14336405551559,-1.14093291874721,-1.13473541317179,
-1.10549895970416,-1.08015610547455,-1.07291039461136,-1.06895207515003,
-1.06556957871674,-1.0614280936387,-1.05502288041877,-1.01515152809839,
-0.997476336090281,-0.992916540144445,-0.990601665430235,-0.988689696233156,
-0.986232812579258,-0.980778604028425,-0.953630680690489,-0.924854703890282,
-0.918350583704046,-0.914180129903392,-0.910795981752568,-0.906860541147936,
-0.899729092546172,-0.875308682999262,-0.847998749724382,-0.839453654853804,
-0.836430689067862,-0.834636393737101,-0.832622393064683,-0.82949058378624,
-0.819203594884595,-0.798609412213889,-0.769625876465328,-0.763124628596293,
-0.75895495005321,-0.755570762541077,-0.751634525082281,-0.744499459965995,
-0.720051244764577,-0.692685845095345,-0.684209210936487,-0.681195075399877,
-0.679402357538995,-0.677386193267486,-0.674244322217734,-0.663856014568973,
-0.642886016807153,-0.61441246624213,-0.60790414398511,-0.603732352207339,
-0.600347967854745,-0.596413206435946,-0.589285745128215,-0.564898521241319,
-0.537656523833296,-0.529023735626237,-0.52598939754516,-0.524192955143136,
-0.522181455130139,-0.519061844668738,-0.508897862206567,-0.488752430631048,
-0.459147264159303,-0.452656356672005,-0.448489564172418,-0.445105368015876,
-0.441166475658373,-0.434018934636533,-0.409473381633096,-0.381912546958663,
-0.37367728374367,-0.370694922915517,-0.368907871851527,-0.366883711054085,
-0.363704659428616,-0.357528053359181),.UNSPECIFIED.);
#924=B_SPLINE_CURVE_WITH_KNOTS('',3,(#79160,#79161,#79162,#79163,#79164,
#79165,#79166,#79167,#79168,#79169,#79170,#79171,#79172,#79173,#79174,#79175,
#79176,#79177,#79178,#79179,#79180,#79181,#79182,#79183,#79184,#79185,#79186,
#79187,#79188,#79189,#79190,#79191,#79192,#79193,#79194,#79195,#79196,#79197,
#79198,#79199,#79200,#79201,#79202,#79203,#79204,#79205,#79206,#79207,#79208,
#79209,#79210,#79211,#79212,#79213,#79214,#79215,#79216,#79217,#79218,#79219,
#79220,#79221,#79222,#79223),.UNSPECIFIED.,.F.,.F.,(4,3,3,3,3,3,3,3,3,3,
3,3,3,3,3,3,3,3,3,3,3,4),(40.8407044972538,41.0794323899344,41.1437651640605,
41.3423764171309,41.5414598026612,41.7396176950701,41.939163827161,42.138709959252,
42.3373212123239,42.5364045978538,42.7345624902641,42.9341086223539,43.1336547544436,
43.3322660075162,43.5313493930459,43.729507285457,43.929053417546,44.1285995496351,
44.3272255543724,44.5254262229014,44.7236012490529,44.8344902319945),
 .UNSPECIFIED.);
#925=B_SPLINE_CURVE_WITH_KNOTS('',3,(#79224,#79225,#79226,#79227,#79228,
#79229,#79230,#79231,#79232,#79233,#79234,#79235,#79236,#79237,#79238,#79239,
#79240,#79241,#79242,#79243,#79244,#79245,#79246,#79247,#79248,#79249,#79250,
#79251,#79252,#79253,#79254,#79255,#79256,#79257,#79258,#79259,#79260),
 .UNSPECIFIED.,.F.,.F.,(4,3,3,3,3,3,3,3,3,3,3,3,4),(38.5521360709588,38.7502960103253,
38.9520857920013,39.1538755736774,39.3524868267472,39.5515702122776,39.7497281046856,
39.9492742367772,40.1488203688689,40.3464146547053,40.5435759929651,40.740698017163,
40.8407044966673),.UNSPECIFIED.);
#926=B_SPLINE_CURVE_WITH_KNOTS('',3,(#79262,#79263,#79264,#79265,#79266,
#79267,#79268,#79269,#79270,#79271,#79272,#79273,#79274,#79275,#79276,#79277,
#79278,#79279,#79280,#79281,#79282,#79283,#79284,#79285,#79286,#79287,#79288,
#79289,#79290,#79291,#79292,#79293,#79294,#79295,#79296,#79297,#79298,#79299,
#79300,#79301,#79302,#79303,#79304,#79305,#79306,#79307,#79308,#79309,#79310,
#79311,#79312,#79313,#79314,#79315,#79316,#79317,#79318,#79319,#79320,#79321,
#79322,#79323,#79324,#79325,#79326,#79327,#79328,#79329,#79330,#79331,#79332,
#79333,#79334,#79335,#79336,#79337,#79338,#79339,#79340,#79341,#79342,#79343,
#79344,#79345,#79346,#79347,#79348,#79349,#79350,#79351),.UNSPECIFIED.,
 .F.,.F.,(4,2,2,2,2,2,2,2,2,2,2,2,2,2,2,2,2,2,2,2,2,2,2,2,2,2,2,2,2,2,2,
2,2,2,2,2,2,2,2,2,2,2,2,2,4),(-0.357528053359181,-0.352930405912873,-0.330462642455156,
-0.304009230386146,-0.297468152475844,-0.293286744040802,-0.289901657857665,
-0.28597402498536,-0.278882326711891,-0.254777871301631,-0.228102710486401,
-0.218743244390323,-0.215619612249958,-0.213806399782365,-0.211813531796777,
-0.208784517756886,-0.199476651462255,-0.182208505324855,-0.14831736500732,
-0.141398888399427,-0.137466728906528,-0.134291370221815,-0.133828565823825,
-0.133649087723284,-0.133563820798045,-0.133266687893385,-0.132993635286933,
-0.13273680585135,-0.132490289554489,-0.13224935607113,-0.132009976436451,
-0.131768500529493,-0.131521419772047,-0.131265174605576,-0.125091814624551,
-0.117449814466257,-0.100593419334615,-0.0755948938769075,-0.063960119168855,
-0.0606101279504411,-0.0585490235715298,-0.0565519714899307,-0.0535023239476616,
-0.044006928678212,-0.000454731073245817),.UNSPECIFIED.);
#927=B_SPLINE_CURVE_WITH_KNOTS('',3,(#79352,#79353,#79354,#79355,#79356,
#79357,#79358,#79359,#79360,#79361,#79362,#79363,#79364,#79365,#79366,#79367,
#79368,#79369,#79370,#79371,#79372,#79373,#79374,#79375,#79376,#79377,#79378,
#79379,#79380,#79381,#79382,#79383,#79384,#79385,#79386,#79387,#79388,#79389,
#79390,#79391,#79392,#79393,#79394,#79395,#79396,#79397,#79398,#79399,#79400,
#79401,#79402,#79403,#79404,#79405,#79406,#79407,#79408,#79409,#79410,#79411,
#79412,#79413,#79414,#79415,#79416,#79417,#79418,#79419,#79420,#79421,#79422,
#79423,#79424,#79425,#79426,#79427,#79428,#79429,#79430,#79431,#79432,#79433,
#79434,#79435,#79436,#79437,#79438,#79439,#79440,#79441,#79442,#79443,#79444,
#79445,#79446,#79447,#79448,#79449,#79450,#79451,#79452,#79453,#79454,#79455,
#79456,#79457,#79458,#79459,#79460,#79461,#79462,#79463,#79464,#79465,#79466,
#79467,#79468,#79469,#79470,#79471,#79472,#79473,#79474,#79475,#79476,#79477),
 .UNSPECIFIED.,.F.,.F.,(4,2,2,2,2,2,2,2,2,2,2,2,2,2,2,2,2,2,2,2,2,2,2,2,
2,2,2,2,2,2,2,2,2,2,2,2,2,2,2,2,2,2,2,2,2,2,2,2,2,2,2,2,2,2,2,2,2,2,2,2,
2,2,4),(-1.96083796406488,-1.95304681045243,-1.94724249161864,-1.94387972686813,
-1.94064315409192,-1.9369955779625,-1.9312507196165,-1.91060233647322,-1.8795195359313,
-1.86874028479968,-1.86556113495289,-1.86353727366749,-1.8617507481269,
-1.85876976042871,-1.85054114363201,-1.82300332314382,-1.79847602423964,
-1.79133165142375,-1.78739393655562,-1.78401041883277,-1.77984403926801,
-1.77335286974085,-1.74374147656501,-1.72358232948348,-1.71341515720326,
-1.71029554206995,-1.70828432844667,-1.70648834936082,-1.70345520650015,
-1.69482822147054,-1.66760920879968,-1.64323986200272,-1.63611542445173,
-1.63218174894907,-1.62879795656762,-1.62462645986952,-1.61811766535295,
-1.58963305853873,-1.56865179009997,-1.55826088380347,-1.55511901872939,
-1.5531031074038,-1.55131078736854,-1.54829766882227,-1.53982580348723,
-1.51248326195216,-1.48805261014567,-1.48092042094419,-1.47698517392718,
-1.47360148933081,-1.46943198782833,-1.46293006829784,-1.43393941257665,
-1.41332999833887,-1.40303920067864,-1.3999072202002,-1.397893400297,-1.39609947380278,
-1.39307754034751,-1.38453773086663,-1.35371901011083,-1.3381574739814,
-1.33767722568999),.UNSPECIFIED.);
#928=B_SPLINE_CURVE_WITH_KNOTS('',3,(#79483,#79484,#79485,#79486,#79487,
#79488,#79489,#79490,#79491,#79492,#79493,#79494,#79495,#79496,#79497,#79498,
#79499,#79500,#79501,#79502,#79503,#79504,#79505,#79506,#79507,#79508,#79509,
#79510,#79511,#79512,#79513,#79514,#79515,#79516,#79517,#79518,#79519,#79520,
#79521,#79522,#79523,#79524,#79525,#79526,#79527,#79528,#79529,#79530,#79531,
#79532,#79533,#79534,#79535,#79536,#79537,#79538,#79539,#79540,#79541,#79542,
#79543,#79544,#79545,#79546),.UNSPECIFIED.,.F.,.F.,(4,3,3,3,3,3,3,3,3,3,
3,3,3,3,3,3,3,3,3,3,3,4),(47.123889804236,47.3221361842061,47.5201262658007,
47.7179229753624,47.9162111610125,48.1083787304012,48.3069899834732,48.5060733690031,
48.7042312614136,48.9037773935032,49.1033235255928,49.3019347786649,49.5010181641948,
49.6991760566053,49.8987221886948,50.0982683207843,50.2968795738564,50.4959629593862,
50.6941208517967,50.8936669838863,51.0932131159759,51.1183439304616),
 .UNSPECIFIED.);
#929=B_SPLINE_CURVE_WITH_KNOTS('',3,(#79547,#79548,#79549,#79550,#79551,
#79552,#79553,#79554,#79555,#79556,#79557,#79558,#79559,#79560,#79561,#79562,
#79563,#79564,#79565,#79566,#79567,#79568,#79569,#79570,#79571,#79572,#79573,
#79574,#79575,#79576,#79577,#79578,#79579,#79580,#79581,#79582,#79583,#79584,
#79585,#79586),.UNSPECIFIED.,.F.,.F.,(4,3,3,3,3,3,3,3,3,3,3,3,3,4),(44.8344902319945,
45.0330984607145,45.1235443448266,45.3221555978987,45.5212389834285,45.719396875839,
45.9189430079286,46.1184891400182,46.3171003930903,46.5161837786202,46.7143416710308,
46.9138878031202,47.1134339352097,47.1238898038468),.UNSPECIFIED.);
#930=B_SPLINE_CURVE_WITH_KNOTS('',3,(#79587,#79588,#79589,#79590,#79591,
#79592,#79593,#79594,#79595,#79596,#79597,#79598,#79599,#79600,#79601,#79602,
#79603,#79604,#79605,#79606,#79607,#79608,#79609,#79610,#79611,#79612,#79613,
#79614,#79615,#79616,#79617,#79618,#79619,#79620,#79621,#79622,#79623,#79624,
#79625,#79626,#79627,#79628,#79629,#79630,#79631,#79632,#79633,#79634,#79635,
#79636,#79637,#79638,#79639,#79640,#79641,#79642,#79643,#79644,#79645,#79646,
#79647,#79648,#79649,#79650,#79651,#79652,#79653,#79654,#79655,#79656,#79657,
#79658,#79659,#79660,#79661,#79662,#79663,#79664,#79665,#79666,#79667,#79668,
#79669,#79670,#79671,#79672,#79673,#79674,#79675,#79676,#79677,#79678,#79679,
#79680,#79681,#79682,#79683,#79684,#79685,#79686,#79687,#79688,#79689,#79690,
#79691,#79692,#79693,#79694,#79695,#79696,#79697,#79698,#79699,#79700,#79701,
#79702,#79703,#79704,#79705,#79706,#79707,#79708,#79709,#79710,#79711,#79712,
#79713,#79714,#79715,#79716,#79717,#79718,#79719,#79720,#79721,#79722,#79723,
#79724,#79725,#79726,#79727,#79728,#79729,#79730,#79731,#79732,#79733,#79734,
#79735,#79736,#79737,#79738,#79739,#79740,#79741,#79742,#79743,#79744,#79745,
#79746,#79747,#79748,#79749,#79750,#79751,#79752,#79753,#79754,#79755,#79756,
#79757,#79758,#79759,#79760,#79761,#79762,#79763,#79764,#79765,#79766,#79767,
#79768,#79769,#79770,#79771,#79772,#79773,#79774,#79775,#79776,#79777,#79778,
#79779,#79780,#79781,#79782),.UNSPECIFIED.,.F.,.F.,(4,2,2,2,2,2,2,2,2,2,
2,2,2,2,2,2,2,2,2,2,2,2,2,2,2,2,2,2,2,2,2,2,2,2,2,2,2,2,2,2,2,2,2,2,2,2,
2,2,2,2,2,2,2,2,2,2,2,2,2,2,2,2,2,2,2,2,2,2,2,2,2,2,2,2,2,2,2,2,2,2,2,2,
2,2,2,2,2,2,2,2,2,2,2,2,2,2,2,4),(-1.33767722568999,-1.32758777835359,-1.32303141189846,
-1.31960689481019,-1.31589682880466,-1.30985261830067,-1.28200486595905,
-1.25889484858637,-1.2479638977264,-1.24477060909482,-1.24274369745994,
-1.24095924370782,-1.23798994641985,-1.22984828668527,-1.19862340166705,
-1.18299694366057,-1.17239746123665,-1.16783636691018,-1.16441114532542,
-1.16070304138677,-1.15466831111083,-1.12822432422046,-1.10839672328695,
-1.09335746220029,-1.089862024917,-1.08776969451602,-1.08581776867339,-1.08337029254853,
-1.07706421998885,-1.04792697751804,-1.02948176853583,-1.01766536794776,
-1.01292130677384,-1.00946746300486,-1.00582766322246,-1.0001210976762,
-0.980514545331224,-0.96197577279904,-0.940414488641052,-0.935599294137241,
-0.93323466224333,-0.931325724820888,-0.928887069720718,-0.923678001038157,
-0.916379871327629,-0.893895414815347,-0.867479001548879,-0.860936771001032,
-0.856755471721608,-0.853371001053217,-0.84944467137143,-0.842357015678196,
-0.818278089212355,-0.791649530879589,-0.78223812635065,-0.779108791531489,
-0.777294729088857,-0.775303450714145,-0.772280983307875,-0.76302829228506,
-0.74593035437169,-0.711772565981,-0.70487778738906,-0.700951198169582,
-0.697566705836158,-0.693385641202473,-0.684994395317839,-0.665838028072912,
-0.633685399221897,-0.626409251452694,-0.623559327457625,-0.621620302616725,
-0.619502848649844,-0.615891682982514,-0.598524199894345,-0.560768142117848,
-0.551129245076641,-0.546772689462995,-0.543364963454298,-0.539595914197941,
-0.533269818437004,-0.525557076908771,-0.508439917774552,-0.482781675156979,
-0.47207557040729,-0.468808028733748,-0.466765084395115,-0.46475404720377,
-0.461635447271984,-0.451477651476305,-0.431351458565568,-0.401730227951145,
-0.395240924444836,-0.391075019245416,-0.387691454355756,-0.383753196137418,
-0.376606514099715,-0.357534662796563),.UNSPECIFIED.);
#931=B_SPLINE_CURVE_WITH_KNOTS('',3,(#79788,#79789,#79790,#79791,#79792,
#79793,#79794,#79795,#79796,#79797,#79798,#79799,#79800,#79801,#79802,#79803,
#79804,#79805,#79806,#79807,#79808,#79809,#79810,#79811,#79812,#79813,#79814,
#79815,#79816,#79817,#79818,#79819,#79820,#79821,#79822,#79823,#79824,#79825,
#79826,#79827,#79828,#79829,#79830,#79831,#79832,#79833,#79834,#79835,#79836,
#79837,#79838,#79839,#79840,#79841,#79842,#79843,#79844,#79845,#79846,#79847,
#79848,#79849,#79850,#79851),.UNSPECIFIED.,.F.,.F.,(4,3,3,3,3,3,3,3,3,3,
3,3,3,3,3,3,3,3,3,3,3,4),(53.4070751110264,53.60487683556,53.8026307996998,
54.000871365885,54.0780475015505,54.2766587546226,54.4757421401524,54.6739000325629,
54.8734461646525,55.072992296742,55.271603549814,55.4706869353439,55.6688448277544,
55.868390959844,56.0679370919336,56.2665483450057,56.4656317305355,56.663789622946,
56.8633357550356,57.0628818871251,57.2615016254264,57.4018228384941),
 .UNSPECIFIED.);
#932=B_SPLINE_CURVE_WITH_KNOTS('',3,(#79852,#79853,#79854,#79855,#79856,
#79857,#79858,#79859,#79860,#79861,#79862,#79863,#79864,#79865,#79866,#79867,
#79868,#79869,#79870,#79871,#79872,#79873,#79874,#79875,#79876,#79877,#79878,
#79879,#79880,#79881,#79882,#79883,#79884,#79885,#79886,#79887,#79888),
 .UNSPECIFIED.,.F.,.F.,(4,3,3,3,3,3,3,3,3,3,3,3,4),(51.1183439304616,51.316887193595,
51.5152054837938,51.7133542196496,51.9119926666512,52.0881579111674,52.2867691642395,
52.4858525497693,52.6840104421798,52.8835565742693,53.0831027063589,53.3166318695731,
53.4070751106813),.UNSPECIFIED.);
#933=B_SPLINE_CURVE_WITH_KNOTS('',3,(#79890,#79891,#79892,#79893,#79894,
#79895,#79896,#79897,#79898,#79899,#79900,#79901,#79902,#79903,#79904,#79905,
#79906,#79907,#79908,#79909,#79910,#79911,#79912,#79913,#79914,#79915,#79916,
#79917,#79918,#79919,#79920,#79921,#79922,#79923,#79924,#79925,#79926,#79927,
#79928,#79929,#79930,#79931,#79932,#79933,#79934,#79935,#79936,#79937,#79938,
#79939,#79940,#79941,#79942,#79943,#79944,#79945,#79946,#79947,#79948,#79949,
#79950,#79951,#79952,#79953,#79954,#79955,#79956,#79957,#79958,#79959,#79960,
#79961,#79962,#79963),.UNSPECIFIED.,.F.,.F.,(4,2,2,2,2,2,2,2,2,2,2,2,2,
2,2,2,2,2,2,2,2,2,2,2,2,2,2,2,2,2,2,2,2,2,2,2,4),(-0.357534662796563,-0.352061828879747,
-0.324498669175415,-0.316274119770007,-0.313293541342923,-0.311507040490122,
-0.3094829386353,-0.306303005978516,-0.295515099266277,-0.272988406159206,
-0.246636203584961,-0.240088643261087,-0.235905779400237,-0.232521189203807,
-0.228596001578112,-0.221514077821605,-0.197480187724382,-0.170941112393686,
-0.161412833877342,-0.158269898576684,-0.156453226423311,-0.154464468402554,
-0.151454605303766,-0.142313863550418,-0.125561751627027,-0.0908133378192396,
-0.083976867451929,-0.0800628176783954,-0.0766773044227989,-0.0724797197577981,
-0.0639999283873764,-0.0425180059851325,-0.0086660516945617,-0.00422403248952863,
-0.00211299992500007,-0.00103772143207282,-0.000454279888563791),
 .UNSPECIFIED.);
#934=B_SPLINE_CURVE_WITH_KNOTS('',3,(#79964,#79965,#79966,#79967,#79968,
#79969,#79970,#79971,#79972,#79973,#79974,#79975,#79976,#79977,#79978,#79979,
#79980,#79981,#79982,#79983,#79984,#79985,#79986,#79987,#79988,#79989,#79990,
#79991,#79992,#79993,#79994,#79995,#79996,#79997,#79998,#79999,#80000,#80001,
#80002,#80003,#80004,#80005,#80006,#80007,#80008,#80009,#80010,#80011,#80012,
#80013,#80014,#80015,#80016,#80017,#80018,#80019,#80020,#80021,#80022,#80023,
#80024,#80025,#80026,#80027,#80028,#80029,#80030,#80031,#80032,#80033,#80034,
#80035,#80036,#80037,#80038,#80039,#80040,#80041,#80042,#80043,#80044,#80045,
#80046,#80047,#80048,#80049,#80050,#80051,#80052,#80053,#80054,#80055,#80056,
#80057,#80058,#80059,#80060,#80061,#80062,#80063,#80064,#80065,#80066,#80067,
#80068,#80069,#80070,#80071,#80072,#80073,#80074,#80075,#80076,#80077,#80078,
#80079,#80080,#80081,#80082,#80083,#80084,#80085,#80086,#80087,#80088,#80089),
 .UNSPECIFIED.,.F.,.F.,(4,2,2,2,2,2,2,2,2,2,2,2,2,2,2,2,2,2,2,2,2,2,2,2,
2,2,2,2,2,2,2,2,2,2,2,2,2,2,2,2,2,2,2,2,2,2,2,2,2,2,2,2,2,2,2,2,2,2,2,2,
2,2,4),(-1.96085464133602,-1.95969799413353,-1.95743610396883,-1.95136541439688,
-1.92040753629392,-1.89819815000253,-1.88995811661379,-1.88580586328573,
-1.88242331915766,-1.87847486509316,-1.87147666912248,-1.83859073280341,
-1.82068973381756,-1.81118460161822,-1.80813445813614,-1.80613776241746,
-1.8043294845226,-1.8012297961438,-1.79206528041586,-1.7618730798397,-1.74321140454887,
-1.73483965017737,-1.73066261100245,-1.72727876573915,-1.72335000353586,
-1.71644366423225,-1.68238854497493,-1.66521092016379,-1.65593327085967,
-1.65290818501971,-1.65091656906165,-1.64910334223822,-1.64597760466422,
-1.63659397407287,-1.60996931413919,-1.58589774378847,-1.57881149071345,
-1.57488574142084,-1.57150163731259,-1.56732062158679,-1.56077843628138,
-1.53431396178902,-1.51184206421005,-1.50454535163472,-1.49933763829812,
-1.49689937938828,-1.49499064763575,-1.49262612752588,-1.48781073918378,
-1.46615109303773,-1.44741320562003,-1.43435348658196,-1.42499341976237,
-1.4206378635691,-1.41723895996088,-1.41342954093794,-1.40690902358106,
-1.36898803671565,-1.34877064913869,-1.34393436047819,-1.34156569697933,
-1.33984681549977,-1.33778719751885),.UNSPECIFIED.);
#935=B_SPLINE_CURVE_WITH_KNOTS('',3,(#80095,#80096,#80097,#80098,#80099,
#80100,#80101,#80102,#80103,#80104,#80105,#80106,#80107,#80108,#80109,#80110,
#80111,#80112,#80113,#80114,#80115,#80116,#80117,#80118,#80119,#80120,#80121,
#80122,#80123,#80124,#80125,#80126,#80127,#80128,#80129,#80130,#80131,#80132,
#80133,#80134,#80135,#80136,#80137,#80138,#80139,#80140,#80141,#80142,#80143,
#80144,#80145,#80146,#80147,#80148,#80149,#80150,#80151,#80152,#80153,#80154,
#80155,#80156,#80157,#80158),.UNSPECIFIED.,.F.,.F.,(4,3,3,3,3,3,3,3,3,3,
3,3,3,3,3,3,3,3,3,3,3,4),(59.6902604185821,59.9168207671643,60.0477162726997,
60.2463275257718,60.4454109113016,60.6435688037121,60.8431149358017,61.0426610678912,
61.241272320963,61.4403557064929,61.6385135989031,61.838059730993,62.0376058630828,
62.2362171161554,62.4353005016851,62.6334583940962,62.8330045261852,63.0325506582743,
63.2311657262726,63.4293532087799,63.6274455226886,63.6841456582349),
 .UNSPECIFIED.);
#936=B_SPLINE_CURVE_WITH_KNOTS('',3,(#80159,#80160,#80161,#80162,#80163,
#80164,#80165,#80166,#80167,#80168,#80169,#80170,#80171,#80172,#80173,#80174,
#80175,#80176,#80177,#80178,#80179,#80180,#80181,#80182,#80183,#80184,#80185,
#80186,#80187,#80188,#80189,#80190,#80191,#80192,#80193,#80194,#80195,#80196,
#80197,#80198),.UNSPECIFIED.,.F.,.F.,(4,3,3,3,3,3,3,3,3,3,3,3,3,4),(57.4018228384941,
57.6000162812558,57.7981657536071,57.9967750996259,58.0578266823166,58.2564379353886,
58.4555213209185,58.653679213329,58.8532253454186,59.0527714775082,59.2522974269614,
59.4513573899721,59.6502389193865,59.690260418206),.UNSPECIFIED.);
#937=B_SPLINE_CURVE_WITH_KNOTS('',3,(#80199,#80200,#80201,#80202,#80203,
#80204,#80205,#80206,#80207,#80208,#80209,#80210,#80211,#80212,#80213,#80214,
#80215,#80216,#80217,#80218,#80219,#80220,#80221,#80222,#80223,#80224,#80225,
#80226,#80227,#80228,#80229,#80230,#80231,#80232,#80233,#80234,#80235,#80236,
#80237,#80238,#80239,#80240,#80241,#80242,#80243,#80244,#80245,#80246,#80247,
#80248,#80249,#80250,#80251,#80252,#80253,#80254,#80255,#80256,#80257,#80258,
#80259,#80260,#80261,#80262,#80263,#80264,#80265,#80266,#80267,#80268,#80269,
#80270,#80271,#80272,#80273,#80274,#80275,#80276,#80277,#80278,#80279,#80280,
#80281,#80282,#80283,#80284,#80285,#80286,#80287,#80288,#80289,#80290,#80291,
#80292,#80293,#80294,#80295,#80296,#80297,#80298,#80299,#80300,#80301,#80302,
#80303,#80304,#80305,#80306,#80307,#80308,#80309,#80310,#80311,#80312,#80313,
#80314,#80315,#80316,#80317,#80318,#80319,#80320,#80321,#80322,#80323,#80324,
#80325,#80326,#80327,#80328,#80329,#80330,#80331,#80332,#80333,#80334,#80335,
#80336,#80337,#80338,#80339,#80340,#80341,#80342,#80343,#80344,#80345,#80346,
#80347,#80348,#80349,#80350,#80351,#80352,#80353,#80354,#80355,#80356,#80357,
#80358,#80359,#80360,#80361,#80362,#80363,#80364,#80365,#80366,#80367,#80368,
#80369,#80370,#80371,#80372,#80373,#80374,#80375,#80376,#80377,#80378,#80379,
#80380,#80381,#80382,#80383,#80384,#80385,#80386,#80387,#80388,#80389,#80390),
 .UNSPECIFIED.,.F.,.F.,(4,2,2,2,2,2,2,2,2,2,2,2,2,2,2,2,2,2,2,2,2,2,2,2,
2,2,2,2,2,2,2,2,2,2,2,2,2,2,2,2,2,2,2,2,2,2,2,2,2,2,2,2,2,2,2,2,2,2,2,2,
2,2,2,2,2,2,2,2,2,2,2,2,2,2,2,2,2,2,2,2,2,2,2,2,2,2,2,2,2,2,2,2,2,2,2,4),
(-1.33778719751885,-1.33751221745128,-1.33299621567242,-1.30464861401804,
-1.27749033601146,-1.26919469364743,-1.26503172412641,-1.26164837235187,
-1.25770791599161,-1.25074805823796,-1.21731603656382,-1.19975554880528,
-1.19035618530923,-1.187317437687,-1.1853229416187,-1.18351223618444,-1.18040029179032,
-1.17113481752426,-1.14441608402247,-1.12029635960102,-1.11320362196044,
-1.10927635227059,-1.10589206099999,-1.10171225452133,-1.09517488784827,
-1.06863332557585,-1.04620953932327,-1.03892047779849,-1.03371667406926,
-1.03127901133978,-1.02937014559124,-1.0270047120971,-1.02218518799183,
-1.0001975563674,-0.980868736069392,-0.962327044704108,-0.956718033819915,
-0.953098403216103,-0.949633816287525,-0.9448261467839,-0.932557469639629,
-0.912970084656786,-0.882492446579291,-0.878124913519015,-0.875821504477149,
-0.873908638244104,-0.871395435592714,-0.865769678650637,-0.857661050152863,
-0.829582926953075,-0.80760515716153,-0.80175517977091,-0.798085498906799,
-0.794645301848536,-0.789986232540218,-0.778751472055754,-0.761694217390857,
-0.736186915923587,-0.725269080691368,-0.721982143950538,-0.719934925976592,
-0.717927345570818,-0.714825618514982,-0.704834755305202,-0.685301868483314,
-0.654847463860384,-0.648374947689261,-0.644213790441317,-0.64083028904122,
-0.636887828407406,-0.629721089012569,-0.605018364310719,-0.577135759114778,
-0.569301444026419,-0.566374195312102,-0.564421104361875,-0.562330412970304,
-0.558843043965974,-0.543942320337303,-0.524061475833301,-0.497570131108314,
-0.491525515830468,-0.487815162631819,-0.484390336839105,-0.479833502674628,
-0.469262855973516,-0.453698106628933,-0.422903971952484,-0.414312407371696,
-0.41128352262908,-0.409488188760745,-0.407475666834736,-0.404350639104759,
-0.394130897914863,-0.373782171446824,-0.357647925279928),.UNSPECIFIED.);
#938=B_SPLINE_CURVE_WITH_KNOTS('',3,(#80396,#80397,#80398,#80399,#80400,
#80401,#80402,#80403,#80404,#80405,#80406,#80407,#80408,#80409,#80410,#80411,
#80412,#80413,#80414,#80415,#80416,#80417,#80418,#80419,#80420,#80421,#80422,
#80423,#80424,#80425,#80426,#80427,#80428,#80429,#80430,#80431,#80432,#80433,
#80434,#80435,#80436,#80437,#80438,#80439,#80440,#80441,#80442,#80443,#80444,
#80445,#80446,#80447,#80448,#80449,#80450,#80451,#80452,#80453,#80454,#80455,
#80456,#80457,#80458,#80459),.UNSPECIFIED.,.F.,.F.,(4,3,3,3,3,3,3,3,3,3,
3,3,3,3,3,3,3,3,3,3,3,4),(65.9734457253856,66.0173850438489,66.2159962969183,
66.4150796824488,66.6132375748568,66.8127837069487,67.0123298390405,67.210941092103,
67.4100244776353,67.6081823700362,67.8077285021341,68.007274634232,68.2058858873335,
68.404969272856,68.6031271652955,68.8026732973595,69.0022194294236,69.2008324314782,
69.3991652159293,69.5972999332797,69.7958687306036,69.9675922406437),
 .UNSPECIFIED.);
#939=B_SPLINE_CURVE_WITH_KNOTS('',3,(#80460,#80461,#80462,#80463,#80464,
#80465,#80466,#80467,#80468,#80469,#80470,#80471,#80472,#80473,#80474,#80475,
#80476,#80477,#80478,#80479,#80480,#80481,#80482,#80483,#80484,#80485,#80486,
#80487,#80488,#80489,#80490,#80491,#80492,#80493,#80494,#80495,#80496),
 .UNSPECIFIED.,.F.,.F.,(4,3,3,3,3,3,3,3,3,3,3,3,4),(63.6841456582349,63.8827672257363,
64.0274954534659,64.2261067065363,64.4251900920666,64.6233479844754,64.8228941165664,
65.0224402486574,65.2196936990435,65.4166824879541,65.6134849313515,65.8107437883567,
65.973445725034),.UNSPECIFIED.);
#940=B_SPLINE_CURVE_WITH_KNOTS('',3,(#80498,#80499,#80500,#80501,#80502,
#80503,#80504,#80505,#80506,#80507,#80508,#80509,#80510,#80511,#80512,#80513,
#80514,#80515,#80516,#80517,#80518,#80519,#80520,#80521,#80522,#80523,#80524,
#80525,#80526,#80527,#80528,#80529,#80530,#80531,#80532,#80533,#80534,#80535,
#80536,#80537,#80538,#80539,#80540,#80541,#80542,#80543,#80544,#80545,#80546,
#80547,#80548,#80549,#80550,#80551,#80552,#80553,#80554,#80555,#80556,#80557,
#80558,#80559,#80560,#80561,#80562,#80563,#80564,#80565,#80566,#80567,#80568,
#80569,#80570,#80571,#80572,#80573),.UNSPECIFIED.,.F.,.F.,(4,2,2,2,2,2,
2,2,2,2,2,2,2,2,2,2,2,2,2,2,2,2,2,2,2,2,2,2,2,2,2,2,2,2,2,2,2,4),(-0.357647925279928,
-0.34446326816879,-0.33796778868358,-0.333799866922246,-0.330415886590131,
-0.326478519861799,-0.319337440272169,-0.294840394575903,-0.267375679006825,
-0.259024642703012,-0.256027048405568,-0.254237370812583,-0.252217280794945,
-0.24905671709191,-0.238475133453672,-0.21676731689736,-0.189279745222121,
-0.18276485676467,-0.178591240326989,-0.175206867602713,-0.171273793452703,
-0.164154219425701,-0.139828126827636,-0.112708213190028,-0.10392262960473,
-0.100868987359338,-0.0990690282240539,-0.0970619704908127,-0.093963339168338,
-0.0840043631129348,-0.0531050154374437,-0.0314392653121238,-0.0256302262713167,
-0.0219688461200183,-0.0187254011670891,-0.0153699123580542,-0.00916901388829356,
-0.000453918773602445),.UNSPECIFIED.);
#941=B_SPLINE_CURVE_WITH_KNOTS('',3,(#80574,#80575,#80576,#80577,#80578,
#80579,#80580,#80581,#80582,#80583,#80584,#80585,#80586,#80587,#80588,#80589,
#80590,#80591,#80592,#80593,#80594,#80595,#80596,#80597,#80598,#80599,#80600,
#80601,#80602,#80603,#80604,#80605,#80606,#80607,#80608,#80609,#80610,#80611,
#80612,#80613,#80614,#80615,#80616,#80617,#80618,#80619,#80620,#80621,#80622,
#80623,#80624,#80625,#80626,#80627,#80628,#80629,#80630,#80631,#80632,#80633,
#80634,#80635,#80636,#80637,#80638,#80639,#80640,#80641,#80642,#80643,#80644,
#80645,#80646,#80647,#80648,#80649,#80650,#80651,#80652,#80653,#80654,#80655,
#80656,#80657,#80658,#80659,#80660,#80661,#80662,#80663,#80664,#80665,#80666,
#80667,#80668,#80669,#80670,#80671,#80672,#80673,#80674,#80675,#80676,#80677,
#80678,#80679,#80680,#80681,#80682,#80683,#80684,#80685,#80686,#80687,#80688,
#80689,#80690,#80691,#80692,#80693,#80694,#80695,#80696,#80697,#80698,#80699,
#80700,#80701,#80702,#80703,#80704,#80705,#80706,#80707,#80708,#80709,#80710,
#80711,#80712,#80713,#80714,#80715,#80716,#80717),.UNSPECIFIED.,.F.,.F.,
(4,2,2,2,2,2,2,2,2,2,2,2,2,2,2,2,2,2,2,2,2,2,2,2,2,2,2,2,2,2,2,2,2,2,2,
2,2,2,2,2,2,2,2,2,2,2,2,2,2,2,2,2,2,2,2,2,2,2,2,2,2,2,2,2,2,2,2,2,2,2,2,
4),(-1.96070394248481,-1.92933497661198,-1.91166965002557,-1.90711115802255,
-1.90479663559414,-1.90288477673997,-1.90042780996585,-1.89497254781089,
-1.86064015508601,-1.84455014458124,-1.83712307143501,-1.83108918642525,
-1.830844570577,-1.83060683710871,-1.83037264552342,-1.83013861566442,-1.82990113197663,
-1.82965609209598,-1.82939855324977,-1.82912219347787,-1.82881842813478,
-1.82864790734816,-1.82820317743472,-1.82502933496934,-1.82110692176938,
-1.81423173783217,-1.77988936358417,-1.76286992464413,-1.75364254252336,
-1.75062279968158,-1.74863206018267,-1.74681739760326,-1.74368505697505,
-1.73424749517593,-1.70765945710643,-1.68360477817426,-1.67652010598994,
-1.67259431692131,-1.66920968157123,-1.66502737182054,-1.6584818650549,
-1.63204390313268,-1.60954879192493,-1.60224773093705,-1.59703753317579,
-1.59459860323716,-1.59268958544777,-1.59032500857371,-1.58551040970868,
-1.56394268442181,-1.54538465953001,-1.53216356351257,-1.52272129385147,
-1.51835109220562,-1.5149501691811,-1.51114817892382,-1.50466508386144,
-1.46647073413673,-1.44641973752589,-1.44160023140202,-1.43923458101903,
-1.43751559759742,-1.43517749651291,-1.4304999968888,-1.39570889877599,
-1.37916181007943,-1.36814838523904,-1.36352266638425,-1.36008745121614,
-1.35640476373227,-1.35049328168514,-1.33764393648806),.UNSPECIFIED.);
#942=B_SPLINE_CURVE_WITH_KNOTS('',3,(#80723,#80724,#80725,#80726,#80727,
#80728,#80729,#80730,#80731,#80732,#80733,#80734,#80735,#80736,#80737,#80738,
#80739,#80740,#80741,#80742,#80743,#80744,#80745,#80746,#80747,#80748,#80749,
#80750,#80751,#80752,#80753,#80754,#80755,#80756,#80757,#80758,#80759,#80760,
#80761,#80762,#80763,#80764,#80765,#80766,#80767,#80768,#80769,#80770,#80771,
#80772,#80773,#80774,#80775,#80776,#80777,#80778,#80779,#80780,#80781,#80782,
#80783,#80784,#80785,#80786),.UNSPECIFIED.,.F.,.F.,(4,3,3,3,3,3,3,3,3,3,
3,3,3,3,3,3,3,3,3,3,3,4),(72.2566310325652,72.453061509527,72.6493422534457,
72.8460888556948,72.9819986101897,73.1806098630103,73.379693248603,73.5778511407525,
73.7773972730668,73.9769434053812,74.1755546598248,74.3746380450118,74.5727959387811,
74.772342069677,74.9718882005728,75.1704994517123,75.3695828377253,75.5677407282643,
75.7672868620143,75.9668329957643,76.1654410178161,76.2514750095923),
 .UNSPECIFIED.);
#943=B_SPLINE_CURVE_WITH_KNOTS('',3,(#80787,#80788,#80789,#80790,#80791,
#80792,#80793,#80794,#80795,#80796,#80797,#80798,#80799,#80800,#80801,#80802,
#80803,#80804,#80805,#80806,#80807,#80808,#80809,#80810,#80811,#80812,#80813,
#80814,#80815,#80816,#80817,#80818,#80819,#80820,#80821,#80822,#80823,#80824,
#80825,#80826),.UNSPECIFIED.,.F.,.F.,(4,3,3,3,3,3,3,3,3,3,3,3,3,4),(69.9675922406437,
69.9971642246151,70.1957754776355,70.3948588631782,70.593016755536,70.7925628876713,
70.9921090198066,71.1907202730821,71.3898036585611,71.5879615511726,71.7875076830854,
71.9870538149982,72.2359502938216,72.2566310322155),.UNSPECIFIED.);
#944=B_SPLINE_CURVE_WITH_KNOTS('',3,(#80827,#80828,#80829,#80830,#80831,
#80832,#80833,#80834,#80835,#80836,#80837,#80838,#80839,#80840,#80841,#80842,
#80843,#80844,#80845,#80846,#80847,#80848,#80849,#80850,#80851,#80852,#80853,
#80854,#80855,#80856,#80857,#80858,#80859,#80860,#80861,#80862,#80863,#80864,
#80865,#80866,#80867,#80868,#80869,#80870,#80871,#80872,#80873,#80874,#80875,
#80876,#80877,#80878,#80879,#80880,#80881,#80882,#80883,#80884,#80885,#80886,
#80887,#80888,#80889,#80890,#80891,#80892,#80893,#80894,#80895,#80896,#80897,
#80898,#80899,#80900,#80901,#80902,#80903,#80904,#80905,#80906,#80907,#80908,
#80909,#80910,#80911,#80912,#80913,#80914,#80915,#80916,#80917,#80918,#80919,
#80920,#80921,#80922,#80923,#80924,#80925,#80926,#80927,#80928,#80929,#80930,
#80931,#80932,#80933,#80934,#80935,#80936,#80937,#80938,#80939,#80940,#80941,
#80942,#80943,#80944,#80945,#80946,#80947,#80948,#80949,#80950,#80951,#80952,
#80953,#80954,#80955,#80956,#80957,#80958,#80959,#80960,#80961,#80962,#80963,
#80964,#80965,#80966,#80967,#80968,#80969,#80970,#80971,#80972,#80973,#80974,
#80975,#80976,#80977,#80978,#80979,#80980,#80981,#80982,#80983,#80984,#80985,
#80986,#80987,#80988,#80989,#80990,#80991,#80992,#80993,#80994,#80995,#80996,
#80997,#80998,#80999,#81000,#81001,#81002,#81003,#81004,#81005,#81006,#81007,
#81008,#81009,#81010,#81011,#81012),.UNSPECIFIED.,.F.,.F.,(4,2,2,2,2,2,
2,2,2,2,2,2,2,2,2,2,2,2,2,2,2,2,2,2,2,2,2,2,2,2,2,2,2,2,2,2,2,2,2,2,2,2,
2,2,2,2,2,2,2,2,2,2,2,2,2,2,2,2,2,2,2,2,2,2,2,2,2,2,2,2,2,2,2,2,2,2,2,2,
2,2,2,2,2,2,2,2,2,2,2,2,2,2,4),(-1.33764393648806,-1.32659078915027,-1.30533210274314,
-1.28905713672738,-1.28549559930562,-1.2833887772993,-1.28144427872074,
-1.27902714312095,-1.27291844346281,-1.24359623341503,-1.21958569955851,
-1.21150514551954,-1.2073825602272,-1.204328930668,-1.20047835292542,-1.19393580256984,
-1.15671053439527,-1.13603744734816,-1.13115414686181,-1.12877618766843,
-1.12705652003219,-1.12472958073054,-1.12010936254975,-1.0922176721032,
-1.06093976508601,-1.05480389243963,-1.05107419399002,-1.04765506714192,
-1.04321785182638,-1.03309270536602,-0.999032385775235,-0.980434221343209,
-0.975770041141681,-0.973434445539726,-0.97171519949576,-0.969346528418303,
-0.964511847067524,-0.944315365601489,-0.906384348460499,-0.899866903221876,
-0.896057567158741,-0.892657694546348,-0.888299452911519,-0.878927844766484,
-0.865844975839041,-0.847103500686982,-0.825432853771757,-0.820615263050581,
-0.818249962230202,-0.816340759208371,-0.81390211377172,-0.808694265744745,
-0.801398835773369,-0.778933909603497,-0.752479200204457,-0.745938637483802,
-0.741757491251353,-0.738372575491306,-0.734445093587934,-0.727353533703111,
-0.703248611653748,-0.676571474066634,-0.667216739693597,-0.664093764547102,
-0.66228073727372,-0.660287871163014,-0.657258529329938,-0.647946832937712,
-0.6306660697191,-0.596804025816962,-0.589881042019555,-0.585948034885406,
-0.582563473020931,-0.578389310060931,-0.570036953811306,-0.552118977504699,
-0.546085025841321,-0.516057029883534,-0.510522080404953,-0.508050958350324,
-0.506137845802918,-0.503833910757756,-0.499329667921236,-0.482133399455728,
-0.441382183921242,-0.434548845941095,-0.430635280611452,-0.42724943539701,
-0.423050467938173,-0.414564336920297,-0.392952636386033,-0.366603901696779,
-0.35724220641513),.UNSPECIFIED.);
#945=B_SPLINE_CURVE_WITH_KNOTS('',3,(#81018,#81019,#81020,#81021,#81022,
#81023,#81024,#81025,#81026,#81027,#81028,#81029,#81030,#81031,#81032,#81033,
#81034,#81035,#81036,#81037,#81038,#81039,#81040,#81041,#81042,#81043,#81044,
#81045,#81046,#81047,#81048,#81049,#81050,#81051,#81052,#81053,#81054,#81055,
#81056,#81057,#81058,#81059,#81060,#81061,#81062,#81063,#81064,#81065,#81066,
#81067,#81068,#81069,#81070,#81071,#81072,#81073,#81074,#81075,#81076,#81077,
#81078),.UNSPECIFIED.,.F.,.F.,(4,3,3,3,3,3,3,3,3,3,3,3,3,3,3,3,3,3,3,3,
4),(78.5398163403645,78.7576486565568,78.951667381339,79.1502786332354,
79.3493620190592,79.5475199096511,79.7470660430908,79.9466121765305,80.1452234870737,
80.3443068582357,80.5424648079831,80.7420108898526,80.941556971722,81.1401681098791,
81.3392515241377,81.5374093042427,81.7369555355781,81.9365017669136,82.1351109303009,
82.334472825171,82.533834720041),.UNSPECIFIED.);
#946=B_SPLINE_CURVE_WITH_KNOTS('',3,(#81079,#81080,#81081,#81082,#81083,
#81084,#81085,#81086,#81087,#81088,#81089,#81090,#81091,#81092,#81093,#81094,
#81095,#81096,#81097,#81098,#81099,#81100,#81101,#81102,#81103,#81104,#81105,
#81106,#81107,#81108,#81109,#81110,#81111,#81112,#81113,#81114,#81115),
 .UNSPECIFIED.,.F.,.F.,(4,3,3,3,3,3,3,3,3,3,3,3,4),(76.2514750095923,76.4497181715849,
76.647858216347,76.8464700708751,76.9617777909559,77.160389053035,77.3594724363131,
77.5576303376766,77.757176461912,77.9567225861474,78.1589910006078,78.360779972492,
78.5398163397448),.UNSPECIFIED.);
#947=B_SPLINE_CURVE_WITH_KNOTS('',3,(#81117,#81118,#81119,#81120,#81121,
#81122,#81123,#81124,#81125,#81126,#81127,#81128,#81129,#81130,#81131,#81132,
#81133,#81134,#81135,#81136,#81137,#81138,#81139,#81140,#81141,#81142,#81143,
#81144,#81145,#81146,#81147,#81148,#81149,#81150,#81151,#81152,#81153,#81154,
#81155,#81156,#81157,#81158,#81159,#81160,#81161,#81162,#81163,#81164,#81165,
#81166,#81167,#81168,#81169,#81170,#81171,#81172,#81173,#81174,#81175,#81176,
#81177,#81178,#81179,#81180,#81181,#81182,#81183,#81184,#81185,#81186,#81187,
#81188,#81189,#81190,#81191,#81192,#81193,#81194,#81195,#81196,#81197,#81198,
#81199,#81200,#81201,#81202,#81203,#81204),.UNSPECIFIED.,.F.,.F.,(4,2,2,
2,2,2,2,2,2,2,2,2,2,2,2,2,2,2,2,2,2,2,2,2,2,2,2,2,2,2,2,2,2,2,2,2,2,2,2,
2,2,2,2,4),(-0.35724220641513,-0.356822408920814,-0.353650496406972,-0.3518281511151,
-0.349844379338791,-0.346860167994689,-0.337943880317512,-0.321868961818697,
-0.285909469762527,-0.279209178812092,-0.275324385738072,-0.271968054207344,
-0.267745605652009,-0.259132422140335,-0.235607204093075,-0.205624844051143,
-0.200044979049397,-0.197566145235043,-0.195652521087392,-0.193354747262324,
-0.188880964176308,-0.157624336541427,-0.129180683138258,-0.123199353091418,
-0.119502124419729,-0.116072497057409,-0.115798552356404,-0.115546404610803,
-0.1153097713868,-0.115083828284873,-0.114864686845464,-0.114649053761756,
-0.114433994481021,-0.114216757482325,-0.108301119632023,-0.0877394866270328,
-0.0619269363182737,-0.0471301183757394,-0.0435555235041537,-0.0414458869549523,
-0.0394800878424068,-0.0365897386922399,-0.0332164226697334,-0.000252836880366436),
 .UNSPECIFIED.);
#948=B_SPLINE_CURVE_WITH_KNOTS('',3,(#81205,#81206,#81207,#81208,#81209,
#81210,#81211,#81212,#81213,#81214,#81215,#81216,#81217,#81218,#81219,#81220,
#81221,#81222,#81223,#81224,#81225,#81226,#81227,#81228,#81229,#81230,#81231,
#81232,#81233,#81234,#81235,#81236,#81237,#81238,#81239,#81240,#81241,#81242,
#81243,#81244,#81245,#81246,#81247,#81248,#81249,#81250,#81251,#81252,#81253,
#81254,#81255,#81256,#81257,#81258,#81259,#81260,#81261,#81262,#81263,#81264,
#81265,#81266,#81267,#81268,#81269,#81270,#81271,#81272,#81273,#81274,#81275,
#81276,#81277,#81278,#81279,#81280,#81281,#81282,#81283,#81284,#81285,#81286,
#81287,#81288,#81289,#81290,#81291,#81292,#81293,#81294,#81295,#81296,#81297,
#81298,#81299,#81300,#81301,#81302,#81303,#81304,#81305,#81306,#81307,#81308,
#81309,#81310,#81311,#81312,#81313,#81314,#81315,#81316,#81317,#81318,#81319,
#81320,#81321,#81322,#81323,#81324,#81325,#81326,#81327,#81328),
 .UNSPECIFIED.,.F.,.F.,(4,2,2,2,2,2,2,2,2,2,2,2,2,2,2,2,2,2,2,2,2,2,2,2,
2,2,2,2,2,2,2,2,2,2,2,2,2,2,2,2,2,2,2,2,2,2,2,2,2,2,2,2,2,2,2,2,2,2,2,2,
2,4),(-1.96097123673854,-1.93544878824503,-1.9307836078925,-1.92734818430412,
-1.92388135748319,-1.92069499585623,-1.91548164960046,-1.90109442939945,
-1.865759950493,-1.85552578794693,-1.85022311985131,-1.84774122912439,-1.8458479462265,
-1.84352848164422,-1.8389454120148,-1.80368554852454,-1.78733620019686,
-1.77641042110183,-1.77179826467768,-1.7683652435406,-1.76467751706006,
-1.75874133784427,-1.73365165564656,-1.70819814799854,-1.70044158786916,
-1.69499498755983,-1.69251328204544,-1.69062004338693,-1.68830051147821,
-1.68371696872555,-1.64843377421369,-1.63210007874355,-1.62118132453413,
-1.61657030320878,-1.61313750516251,-1.60944943405163,-1.60351138407857,
-1.5783449692973,-1.55295665930332,-1.54520954754212,-1.53976781837696,
-1.53728700949584,-1.53539386058388,-1.53307369614114,-1.52848681416989,
-1.49322206834498,-1.4768811387022,-1.46595924005697,-1.46134779237403,
-1.457914983222,-1.45422718802596,-1.44829023075563,-1.42316176599186,-1.39774250440246,
-1.38999101924419,-1.38454707648446,-1.38206590265396,-1.38017276496632,
-1.37785297666854,-1.37326785735491,-1.33799504523619,-1.33764837993426),
 .UNSPECIFIED.);
#949=B_SPLINE_CURVE_WITH_KNOTS('',3,(#81334,#81335,#81336,#81337,#81338,
#81339,#81340,#81341,#81342,#81343,#81344,#81345,#81346,#81347,#81348,#81349,
#81350,#81351,#81352,#81353,#81354,#81355,#81356,#81357,#81358,#81359,#81360,
#81361,#81362,#81363,#81364,#81365,#81366,#81367,#81368,#81369,#81370,#81371,
#81372,#81373,#81374,#81375,#81376,#81377,#81378,#81379,#81380,#81381,#81382,
#81383,#81384,#81385,#81386,#81387,#81388,#81389,#81390,#81391,#81392,#81393,
#81394,#81395,#81396,#81397),.UNSPECIFIED.,.F.,.F.,(4,3,3,3,3,3,3,3,3,3,
3,3,3,3,3,3,3,3,3,3,3,4),(84.8230016469244,84.9213361524882,85.1199478699099,
85.3190311393523,85.5171894595963,85.716735203638,85.9162809476797,86.1148942966719,
86.3139771582217,86.5121371632032,86.7116814530373,86.9112257428713,87.1098309667632,
87.3089158595881,87.5070678206575,87.7066191793601,87.9061705380628,88.1047926557453,
88.303092888702,88.5011927562955,88.699619191771,88.8169224278005),
 .UNSPECIFIED.);
#950=B_SPLINE_CURVE_WITH_KNOTS('',3,(#81398,#81399,#81400,#81401,#81402,
#81403,#81404,#81405,#81406,#81407,#81408,#81409,#81410,#81411,#81412,#81413,
#81414,#81415,#81416,#81417,#81418,#81419,#81420,#81421,#81422,#81423,#81424,
#81425,#81426,#81427,#81428,#81429,#81430,#81431,#81432,#81433,#81434),
 .UNSPECIFIED.,.F.,.F.,(4,3,3,3,3,3,3,3,3,3,3,3,4),(82.533834720041,82.732640641073,
82.9314465621051,83.1300581696947,83.3291414665952,83.5272997142751,83.7268455357858,
83.9263913572966,84.1225530095749,84.3184285456288,84.5141253382016,84.7102046185275,
84.8230016464018),.UNSPECIFIED.);
#951=B_SPLINE_CURVE_WITH_KNOTS('',3,(#81435,#81436,#81437,#81438,#81439,
#81440,#81441,#81442,#81443,#81444,#81445,#81446,#81447,#81448,#81449,#81450,
#81451,#81452,#81453,#81454,#81455,#81456,#81457,#81458,#81459,#81460,#81461,
#81462,#81463,#81464,#81465,#81466,#81467,#81468,#81469,#81470,#81471,#81472,
#81473,#81474,#81475,#81476,#81477,#81478,#81479,#81480,#81481,#81482,#81483,
#81484,#81485,#81486,#81487,#81488,#81489,#81490,#81491,#81492,#81493,#81494,
#81495,#81496,#81497,#81498,#81499,#81500,#81501,#81502,#81503,#81504,#81505,
#81506,#81507,#81508,#81509,#81510,#81511,#81512,#81513,#81514,#81515,#81516,
#81517,#81518,#81519,#81520,#81521,#81522,#81523,#81524,#81525,#81526,#81527,
#81528,#81529,#81530,#81531,#81532,#81533,#81534,#81535,#81536,#81537,#81538,
#81539,#81540,#81541,#81542,#81543,#81544,#81545,#81546,#81547,#81548,#81549,
#81550,#81551,#81552,#81553,#81554,#81555,#81556,#81557,#81558,#81559,#81560,
#81561,#81562,#81563,#81564,#81565,#81566,#81567,#81568,#81569,#81570,#81571,
#81572,#81573,#81574,#81575,#81576,#81577,#81578,#81579,#81580,#81581,#81582,
#81583,#81584,#81585,#81586,#81587,#81588,#81589,#81590,#81591,#81592,#81593,
#81594,#81595,#81596,#81597,#81598,#81599,#81600,#81601,#81602,#81603,#81604,
#81605,#81606,#81607,#81608,#81609,#81610,#81611,#81612,#81613,#81614,#81615,
#81616,#81617,#81618,#81619,#81620,#81621,#81622,#81623,#81624,#81625,#81626,
#81627,#81628,#81629,#81630),.UNSPECIFIED.,.F.,.F.,(4,2,2,2,2,2,2,2,2,2,
2,2,2,2,2,2,2,2,2,2,2,2,2,2,2,2,2,2,2,2,2,2,2,2,2,2,2,2,2,2,2,2,2,2,2,2,
2,2,2,2,2,2,2,2,2,2,2,2,2,2,2,2,2,2,2,2,2,2,2,2,2,2,2,2,2,2,2,2,2,2,2,2,
2,2,2,2,2,2,2,2,2,2,2,2,2,2,2,4),(-1.33764837993426,-1.32165810253604,-1.31073804337826,
-1.30612693446348,-1.30269422892397,-1.2990064054951,-1.29306908852945,
-1.26792279772655,-1.24627596486119,-1.23153357172201,-1.22805536621762,
-1.22596672666616,-1.22401255626506,-1.22155650316898,-1.21518196032515,
-1.18610221571187,-1.16083126561247,-1.15359433587048,-1.1496377758412,
-1.14625517243094,-1.14211152867885,-1.13569894365946,-1.10336918517922,
-1.08510125263788,-1.07548312239255,-1.07242048652656,-1.07042103974912,
-1.06836389702773,-1.06503111073197,-1.05358746507316,-1.02847935360512,
-1.00726130090864,-0.999027706381584,-0.994876273035988,-0.991493280153546,
-0.987543036962968,-0.980538232961267,-0.956451018629418,-0.929806678131979,
-0.92041441546276,-0.917287266944642,-0.915473588273764,-0.913481828396923,
-0.910457150452979,-0.90118517021443,-0.88402744118857,-0.849967606465764,
-0.843063428827941,-0.839134747891653,-0.835750304186665,-0.83157167268334,
-0.823193836926178,-0.804446510178452,-0.773948860844069,-0.765061632318366,
-0.761995393534293,-0.760193158739031,-0.75818895983127,-0.755103802600909,
-0.745273606516182,-0.726295947047053,-0.695049120900939,-0.688596761355418,
-0.684441364973233,-0.681058003851479,-0.677110567447394,-0.66991977471846,
-0.645025481726327,-0.616751452980132,-0.609394446240116,-0.606531407471489,
-0.604589995903919,-0.602477227718807,-0.598887961390896,-0.582018916142274,
-0.546915379310128,-0.535219056371545,-0.530376653344707,-0.526940370528925,
-0.523338876336458,-0.517818758274082,-0.498812804566657,-0.479636234585103,
-0.457731627679638,-0.452911554985154,-0.450545945761603,-0.448636991192947,
-0.446199306962801,-0.440995736158348,-0.43370816828533,-0.411288894065386,
-0.384769545814982,-0.378234104175473,-0.374054671587356,-0.37067017430508,
-0.366742096133908,-0.359646354434851,-0.357466815432906),.UNSPECIFIED.);
#952=B_SPLINE_CURVE_WITH_KNOTS('',3,(#81636,#81637,#81638,#81639,#81640,
#81641,#81642,#81643,#81644,#81645,#81646,#81647,#81648,#81649,#81650,#81651,
#81652,#81653,#81654,#81655,#81656,#81657,#81658,#81659,#81660,#81661,#81662,
#81663,#81664,#81665,#81666,#81667,#81668,#81669,#81670,#81671,#81672,#81673,
#81674,#81675,#81676,#81677,#81678,#81679,#81680,#81681,#81682,#81683,#81684,
#81685,#81686,#81687,#81688,#81689,#81690,#81691,#81692,#81693,#81694,#81695,
#81696,#81697,#81698,#81699),.UNSPECIFIED.,.F.,.F.,(4,3,3,3,3,3,3,3,3,3,
3,3,3,3,3,3,3,3,3,3,3,4),(91.1061869544955,91.3019231704377,91.4974252818407,
91.6933906075753,91.885949718829,92.0846205836694,92.2836890662572,92.4819083883214,
92.681401451171,92.8808945140205,93.0792205808948,93.2783752629741,93.4762509314101,
93.676045120311,93.875839309212,94.0748286238527,94.2738174939904,94.4723404042387,
94.6715622543211,94.8707841044036,95.0696932795969,95.1011120778127),
 .UNSPECIFIED.);
#953=B_SPLINE_CURVE_WITH_KNOTS('',3,(#81700,#81701,#81702,#81703,#81704,
#81705,#81706,#81707,#81708,#81709,#81710,#81711,#81712,#81713,#81714,#81715,
#81716,#81717,#81718,#81719,#81720,#81721,#81722,#81723,#81724,#81725,#81726,
#81727,#81728,#81729,#81730,#81731,#81732,#81733,#81734,#81735,#81736),
 .UNSPECIFIED.,.F.,.F.,(4,3,3,3,3,3,3,3,3,3,3,3,4),(88.8169224278005,88.9011153332543,
89.0997382756417,89.2988187388427,89.4969885119119,89.6965243201789,89.8960601284459,
90.0946293819821,90.2937232673959,90.4918397176078,90.6914223206226,90.8910049236374,
91.106186954104),.UNSPECIFIED.);
#954=B_SPLINE_CURVE_WITH_KNOTS('',3,(#81738,#81739,#81740,#81741,#81742,
#81743,#81744,#81745,#81746,#81747,#81748,#81749,#81750,#81751,#81752,#81753,
#81754,#81755,#81756,#81757,#81758,#81759,#81760,#81761,#81762,#81763,#81764,
#81765,#81766,#81767,#81768,#81769,#81770,#81771,#81772,#81773,#81774,#81775,
#81776,#81777,#81778,#81779,#81780,#81781,#81782,#81783,#81784,#81785,#81786,
#81787,#81788,#81789,#81790,#81791,#81792,#81793,#81794,#81795,#81796,#81797,
#81798,#81799,#81800,#81801,#81802,#81803,#81804,#81805,#81806,#81807,#81808,
#81809,#81810,#81811,#81812,#81813,#81814,#81815,#81816,#81817,#81818,#81819,
#81820,#81821,#81822,#81823,#81824,#81825,#81826,#81827,#81828,#81829,#81830,
#81831,#81832,#81833,#81834,#81835,#81836,#81837,#81838,#81839,#81840,#81841,
#81842,#81843,#81844,#81845,#81846,#81847,#81848,#81849,#81850,#81851),
 .UNSPECIFIED.,.F.,.F.,(4,2,2,2,2,2,2,2,2,2,2,2,2,2,2,2,2,2,2,2,2,2,2,2,
2,2,2,2,2,2,2,2,2,2,2,2,2,2,2,2,2,2,2,2,2,2,2,2,2,2,2,2,2,2,2,2,4),(-0.357466815432906,
-0.335505369566104,-0.308753656232884,-0.299500133901965,-0.296389308718004,
-0.294578676695416,-0.292583469853657,-0.289542586091397,-0.280126391837006,
-0.262513679674971,-0.229204091676723,-0.222237301328509,-0.21829495824427,
-0.214911098029315,-0.210748904360708,-0.202459882276656,-0.175758644558994,
-0.14683741003079,-0.142356826979249,-0.140029425723709,-0.138310021477257,
-0.138266268667842,-0.138228291607211,-0.138195152653209,-0.138166103444295,
-0.138140538750668,-0.138117963388781,-0.138073152228888,-0.138029311126522,
-0.137986357293708,-0.137944214086576,-0.137902810316141,-0.137862079643245,
-0.137821960045959,-0.137782393344716,-0.137743324782,-0.137704702646856,
-0.137666477938929,-0.137628604064892,-0.137591036565843,-0.137553732869206,
-0.137516652063368,-0.137479754690233,-0.137443002555816,-0.137406358554429,
-0.134792103433566,-0.131519171259025,-0.125370551601353,-0.108938515655659,
-0.0736210289563799,-0.066845749561155,-0.0629450966540203,-0.059558690499896,
-0.0553437885576436,-0.0467694157111863,-0.0235830156413483,-0.00025810012616317),
 .UNSPECIFIED.);
#955=B_SPLINE_CURVE_WITH_KNOTS('',3,(#81852,#81853,#81854,#81855,#81856,
#81857,#81858,#81859),.UNSPECIFIED.,.F.,.F.,(4,1,1,1,1,4),(91.106186954104,
91.2110051344337,92.2059499296252,93.2008947248167,94.1958395200083,95.0999839528908),
 .UNSPECIFIED.);
#956=B_SPLINE_CURVE_WITH_KNOTS('',3,(#81863,#81864,#81865,#81866,#81867,
#81868),.UNSPECIFIED.,.F.,.F.,(4,1,1,4),(-4.09254174883834,-3.97977918076615,
-2.98483438557462,-2.06533154845012),.UNSPECIFIED.);
#957=B_SPLINE_CURVE_WITH_KNOTS('',3,(#81872,#81873,#81874,#81875,#81876),
 .UNSPECIFIED.,.F.,.F.,(4,1,4),(0.,0.994944795191534,1.11419103802954),
 .UNSPECIFIED.);
#958=B_SPLINE_CURVE_WITH_KNOTS('',3,(#81878,#81879,#81880,#81881,#81882,
#81883,#81884,#81885,#81886,#81887,#81888,#81889,#81890,#81891,#81892,#81893,
#81894,#81895,#81896,#81897,#81898,#81899,#81900,#81901,#81902,#81903,#81904,
#81905,#81906,#81907,#81908,#81909,#81910,#81911,#81912,#81913,#81914,#81915,
#81916,#81917,#81918,#81919,#81920,#81921,#81922,#81923,#81924,#81925,#81926,
#81927,#81928,#81929,#81930,#81931,#81932,#81933,#81934,#81935,#81936,#81937,
#81938,#81939,#81940,#81941,#81942,#81943,#81944,#81945,#81946,#81947,#81948,
#81949,#81950,#81951,#81952,#81953,#81954,#81955,#81956,#81957,#81958,#81959,
#81960,#81961,#81962,#81963,#81964,#81965,#81966,#81967,#81968,#81969,#81970,
#81971,#81972,#81973,#81974,#81975,#81976,#81977,#81978,#81979,#81980,#81981,
#81982,#81983,#81984,#81985,#81986,#81987,#81988,#81989,#81990,#81991,#81992),
 .UNSPECIFIED.,.F.,.F.,(4,3,3,3,3,3,3,3,3,3,3,3,3,3,3,3,3,3,3,3,3,3,3,3,
3,3,3,3,3,3,3,3,3,3,3,3,3,3,4),(1.11419103802954,1.29735287581724,1.48032203138593,
1.66315115312043,1.84640621249915,1.98988959038307,2.17778566050261,2.36529042623222,
2.55276479925355,2.7402270554159,2.92810799385181,2.98483438557461,3.17276381816055,
3.36031274498174,3.54784651507135,3.73537708606522,3.92333837693577,3.97977918076615,
4.16712482605355,4.35407332305044,4.54099162516431,4.72789741546226,4.91523160890231,
4.97472397595769,5.16238494385731,5.34965485800517,5.53689856155208,5.7241324002202,
5.91179256293985,5.96966877114923,6.15731012319844,6.34456142792096,6.53178829851298,
6.71900632200928,6.90665247879335,6.96461356634077,7.1682696460741,7.3706362873007,
7.39737602502259),.UNSPECIFIED.);
#959=B_SPLINE_CURVE_WITH_KNOTS('',3,(#81994,#81995,#81996,#81997,#81998,
#81999,#82000,#82001,#82002,#82003),.UNSPECIFIED.,.F.,.F.,(4,1,1,1,1,1,
1,4),(7.39737634520912,7.95955836153231,8.95450315672385,9.94944795191539,
10.9443927471069,11.9393375422985,12.93428233749,13.6805616523887),
 .UNSPECIFIED.);
#960=B_SPLINE_CURVE_WITH_KNOTS('',3,(#82005,#82006,#82007,#82008,#82009,
#82010,#82011,#82012,#82013,#82014,#82015),.UNSPECIFIED.,.F.,.F.,(4,1,1,
1,1,1,1,1,4),(13.6805616523887,13.9292271326815,14.9241719278731,15.9191167230646,
16.9140615182562,17.9090063134477,18.9039511086392,19.8988959038308,19.9637469595683),
 .UNSPECIFIED.);
#961=B_SPLINE_CURVE_WITH_KNOTS('',3,(#82017,#82018,#82019,#82020,#82021,
#82022,#82023,#82024,#82025,#82026),.UNSPECIFIED.,.F.,.F.,(4,1,1,1,1,1,
1,4),(19.9637469595683,20.8938406990223,21.8887854942138,22.8837302894054,
23.8786750845969,24.8736198797885,25.86856467498,26.2469322667479),
 .UNSPECIFIED.);
#962=B_SPLINE_CURVE_WITH_KNOTS('',3,(#82028,#82029,#82030,#82031,#82032,
#82033,#82034,#82035,#82036,#82037),.UNSPECIFIED.,.F.,.F.,(4,1,1,1,1,1,
1,4),(26.2469322667479,26.8635094701715,27.8584542653631,28.8533990605546,
29.8483438557462,30.8432886509377,31.8382334461292,32.5301175739275),
 .UNSPECIFIED.);
#963=B_SPLINE_CURVE_WITH_KNOTS('',3,(#82039,#82040,#82041,#82042,#82043,
#82044,#82045,#82046,#82047,#82048,#82049,#82050,#82051,#82052,#82053,#82054,
#82055,#82056,#82057,#82058,#82059,#82060,#82061,#82062,#82063,#82064,#82065,
#82066,#82067,#82068,#82069,#82070,#82071,#82072,#82073,#82074,#82075,#82076,
#82077,#82078,#82079,#82080,#82081,#82082,#82083,#82084,#82085,#82086,#82087,
#82088,#82089,#82090,#82091,#82092,#82093,#82094,#82095,#82096,#82097,#82098,
#82099,#82100,#82101,#82102,#82103,#82104,#82105,#82106,#82107,#82108,#82109,
#82110,#82111,#82112,#82113,#82114,#82115,#82116,#82117,#82118,#82119,#82120,
#82121,#82122,#82123,#82124,#82125,#82126,#82127,#82128,#82129,#82130,#82131,
#82132,#82133,#82134,#82135,#82136,#82137,#82138,#82139,#82140,#82141,#82142,
#82143,#82144,#82145,#82146,#82147,#82148,#82149,#82150,#82151,#82152,#82153,
#82154,#82155,#82156),.UNSPECIFIED.,.F.,.F.,(4,3,3,3,3,3,3,3,3,3,3,3,3,
3,3,3,3,3,3,3,3,3,3,3,3,3,3,3,3,3,3,3,3,3,3,3,3,3,3,4),(32.530117758059,
32.7556141163704,32.8331782413208,33.0207814298638,33.2079931850932,33.3951790868026,
33.5823552778384,33.7699590877266,33.8281230365123,34.0157262250567,34.2029379802876,
34.3901238819984,34.5773000730357,34.7649038829253,34.8230678317039,35.010671020249,
35.1978827754804,35.3850686771919,35.5722448682299,35.7598486781202,35.8180126268954,
36.0056158154396,36.1928275706703,36.3800134723809,36.5671896634181,36.7547934733075,
36.8129574220869,37.0005606106315,37.1877723658625,37.3749582675735,37.562134458611,
37.7497382685008,37.8079022172785,37.9955054058231,38.1827171610541,38.3699030627651,
38.5570792538025,38.7446830636923,38.80284701247,38.8133028811071),
 .UNSPECIFIED.);
#964=B_SPLINE_CURVE_WITH_KNOTS('',3,(#82158,#82159,#82160,#82161,#82162,
#82163,#82164,#82165,#82166,#82167,#82168,#82169,#82170,#82171,#82172,#82173,
#82174,#82175,#82176,#82177,#82178,#82179,#82180,#82181,#82182,#82183,#82184,
#82185,#82186,#82187,#82188,#82189,#82190,#82191,#82192,#82193,#82194,#82195,
#82196,#82197,#82198,#82199,#82200,#82201,#82202,#82203,#82204,#82205,#82206,
#82207,#82208,#82209,#82210,#82211,#82212,#82213,#82214,#82215,#82216,#82217,
#82218,#82219,#82220,#82221,#82222,#82223,#82224,#82225,#82226,#82227,#82228,
#82229,#82230,#82231,#82232,#82233,#82234,#82235,#82236,#82237,#82238,#82239,
#82240,#82241,#82242,#82243,#82244,#82245,#82246,#82247,#82248,#82249,#82250,
#82251,#82252,#82253,#82254,#82255,#82256,#82257,#82258,#82259,#82260,#82261,
#82262,#82263,#82264,#82265,#82266,#82267,#82268,#82269,#82270,#82271,#82272),
 .UNSPECIFIED.,.F.,.F.,(4,3,3,3,3,3,3,3,3,3,3,3,3,3,3,3,3,3,3,3,3,3,3,3,
3,3,3,3,3,3,3,3,3,3,3,3,3,3,4),(38.8133028814085,39.0005614200088,39.1874299894609,
39.3742739703344,39.5611126744816,39.7483747801438,39.7977918076615,39.9853949962061,
40.1726067514371,40.3597926531481,40.5469688441856,40.7345726540754,40.7927366028531,
40.9803397913976,41.1675515466286,41.3547374483395,41.5419136393771,41.7295174492668,
41.7876813980446,41.9752845865891,42.1624963418201,42.3496822435311,42.5368584345686,
42.7244622444584,42.7826261932362,42.9702293817808,43.1574411370118,43.3446270387228,
43.5318032297602,43.7194070396501,43.7775709884277,43.9651741769722,44.1523859322031,
44.3395718339139,44.5267480249514,44.714351834841,44.7725157836192,44.9931015508383,
45.0964881878767),.UNSPECIFIED.);
#965=B_SPLINE_CURVE_WITH_KNOTS('',3,(#82274,#82275,#82276,#82277,#82278,
#82279,#82280,#82281,#82282,#82283,#82284,#82285,#82286,#82287,#82288,#82289,
#82290,#82291,#82292,#82293,#82294,#82295,#82296,#82297,#82298,#82299,#82300,
#82301,#82302,#82303,#82304,#82305,#82306,#82307,#82308,#82309,#82310,#82311,
#82312,#82313,#82314,#82315,#82316,#82317,#82318,#82319,#82320,#82321,#82322,
#82323,#82324,#82325,#82326,#82327,#82328,#82329,#82330,#82331,#82332,#82333,
#82334,#82335,#82336,#82337,#82338,#82339,#82340,#82341,#82342,#82343,#82344,
#82345,#82346,#82347,#82348,#82349,#82350,#82351,#82352,#82353,#82354,#82355,
#82356,#82357,#82358,#82359,#82360,#82361,#82362,#82363,#82364,#82365,#82366,
#82367,#82368,#82369,#82370,#82371,#82372,#82373,#82374,#82375,#82376,#82377,
#82378,#82379,#82380,#82381,#82382,#82383,#82384,#82385,#82386,#82387,#82388),
 .UNSPECIFIED.,.F.,.F.,(4,3,3,3,3,3,3,3,3,3,3,3,3,3,3,3,3,3,3,3,3,3,3,3,
3,3,3,3,3,3,3,3,3,3,3,3,3,3,4),(45.0964881882867,45.2833267165581,45.4701172611129,
45.6573702632114,45.7674605788108,45.9550637673553,46.1422755225862,46.3294614242972,
46.5166376153346,46.7042414252244,46.7624053740023,46.9500085625469,47.1372203177779,
47.3244062194889,47.5115824105264,47.6991862204162,47.7573501691939,47.9449533577385,
48.1321651129695,48.3193510146805,48.506527205718,48.6941310156078,48.7522949643854,
48.9398981529299,49.1271099081609,49.3142958098718,49.5014720009093,49.689075810799,
49.7472397595769,49.9348429481215,50.1220547033524,50.3092406050634,50.4964167961009,
50.6840206059907,50.7421845547685,50.9306517424822,51.1186979603826,51.3065834404951,
51.3796734954662),.UNSPECIFIED.);
#966=B_SPLINE_CURVE_WITH_KNOTS('',3,(#82390,#82391,#82392,#82393,#82394,
#82395,#82396,#82397,#82398,#82399,#82400,#82401,#82402,#82403,#82404,#82405,
#82406,#82407,#82408,#82409,#82410,#82411,#82412,#82413,#82414,#82415,#82416,
#82417,#82418,#82419,#82420,#82421,#82422,#82423,#82424,#82425,#82426,#82427,
#82428,#82429,#82430,#82431,#82432,#82433,#82434,#82435,#82436,#82437,#82438,
#82439,#82440,#82441,#82442,#82443,#82444,#82445,#82446,#82447,#82448,#82449,
#82450,#82451,#82452,#82453,#82454,#82455,#82456,#82457,#82458,#82459,#82460,
#82461,#82462,#82463,#82464,#82465,#82466,#82467,#82468,#82469,#82470,#82471,
#82472,#82473,#82474,#82475,#82476,#82477,#82478,#82479,#82480,#82481,#82482,
#82483,#82484,#82485,#82486,#82487,#82488,#82489,#82490,#82491,#82492,#82493,
#82494,#82495,#82496,#82497,#82498,#82499,#82500,#82501),.UNSPECIFIED.,
 .F.,.F.,(4,3,3,3,3,3,3,3,3,3,3,3,3,3,3,3,3,3,3,3,3,3,3,3,3,3,3,3,3,3,3,
3,3,3,3,3,3,4),(51.3796734959224,51.5936766963176,51.73712934996,51.9247325385046,
52.1119442937356,52.2991301954466,52.4863063864841,52.6739101963739,52.7320741451516,
52.9196773336959,53.1068890889265,53.2940749906372,53.4812511816744,53.6688549915638,
53.7270189403431,53.9146221288881,54.1018338841196,54.289019785831,54.476195976869,
54.6637997867592,54.7219637355346,54.909566924079,55.0967786793098,55.2839645810207,
55.471140772058,55.6587445819477,55.7169085307262,55.9045117192692,56.0917234744985,
56.2789093762079,56.4660855672438,56.653689377132,56.7118533259177,56.8981739682351,
57.0893451767646,57.2752466163079,57.4690527093306,57.6628588023532),
 .UNSPECIFIED.);
#967=B_SPLINE_CURVE_WITH_KNOTS('',3,(#82503,#82504,#82505,#82506,#82507,
#82508,#82509,#82510,#82511,#82512,#82513,#82514,#82515,#82516,#82517,#82518,
#82519,#82520,#82521,#82522,#82523,#82524,#82525,#82526,#82527,#82528,#82529,
#82530,#82531,#82532,#82533,#82534,#82535,#82536,#82537,#82538,#82539,#82540,
#82541,#82542,#82543,#82544,#82545,#82546,#82547,#82548,#82549,#82550,#82551,
#82552,#82553,#82554,#82555,#82556,#82557,#82558,#82559,#82560,#82561,#82562,
#82563,#82564,#82565,#82566,#82567,#82568,#82569,#82570,#82571,#82572,#82573,
#82574,#82575,#82576,#82577,#82578,#82579,#82580,#82581,#82582,#82583,#82584,
#82585,#82586,#82587,#82588,#82589,#82590,#82591,#82592,#82593,#82594,#82595,
#82596,#82597,#82598,#82599,#82600,#82601,#82602,#82603,#82604,#82605,#82606,
#82607,#82608,#82609,#82610,#82611,#82612,#82613,#82614,#82615,#82616,#82617,
#82618,#82619,#82620),.UNSPECIFIED.,.F.,.F.,(4,3,3,3,3,3,3,3,3,3,3,3,3,
3,3,3,3,3,3,3,3,3,3,3,3,3,3,3,3,3,3,3,3,3,3,3,3,3,3,4),(57.6628588026459,
57.7067981211093,57.8944013096513,58.0816130648797,58.2687989665883,58.4559751576235,
58.643578967511,58.7017429163008,58.8893461048363,59.0765578600581,59.2637437617599,
59.4509199527882,59.638523762669,59.6966877114923,59.8842909000647,60.0715026553235,
60.258688557062,60.4458647481267,60.6334685580429,60.6916325066839,60.8792356952034,
61.0664474504096,61.2536333520967,61.4408095431107,61.6284133529781,61.6865773018754,
61.8741804903711,62.0613922455524,62.2485781472136,62.435754338201,62.6233581480414,
62.6815220970669,62.8691252858037,63.0563370412272,63.243522943128,63.4306991343541,
63.6183029444271,63.6764668922585,63.9115682388477,63.9460441094081),
 .UNSPECIFIED.);
#968=B_SPLINE_CURVE_WITH_KNOTS('',3,(#82622,#82623,#82624,#82625,#82626,
#82627,#82628,#82629,#82630,#82631,#82632,#82633,#82634,#82635,#82636,#82637,
#82638,#82639,#82640,#82641,#82642,#82643,#82644,#82645,#82646,#82647,#82648,
#82649,#82650,#82651,#82652,#82653,#82654,#82655,#82656,#82657,#82658,#82659,
#82660,#82661,#82662,#82663,#82664,#82665,#82666,#82667,#82668,#82669,#82670,
#82671,#82672,#82673,#82674,#82675,#82676,#82677,#82678,#82679,#82680,#82681,
#82682,#82683,#82684,#82685,#82686,#82687,#82688,#82689,#82690,#82691,#82692,
#82693,#82694,#82695,#82696,#82697,#82698,#82699,#82700,#82701,#82702,#82703,
#82704,#82705,#82706,#82707,#82708,#82709,#82710,#82711,#82712,#82713,#82714,
#82715,#82716,#82717,#82718,#82719,#82720,#82721,#82722,#82723,#82724,#82725,
#82726,#82727,#82728,#82729,#82730,#82731,#82732,#82733),.UNSPECIFIED.,
 .F.,.F.,(4,3,3,3,3,3,3,3,3,3,3,3,3,3,3,3,3,3,3,3,3,3,3,3,3,3,3,3,3,3,3,
3,3,3,3,3,3,4),(63.9460441098254,64.131587392169,64.3169915432042,64.5028443208997,
64.67141168745,64.8590148757571,65.0462266307455,65.2334125322104,65.4205887229996,
65.6081925326422,65.6663564826416,65.8539596724817,66.0411714290113,66.2283573320057,
66.4155335243191,66.6031373354505,66.6613012778331,66.8489044645521,67.0361162179695,
67.223302117911,67.4104783072031,67.5980821154138,67.6562460730246,67.8438492606578,
68.0310610149416,68.2182469156685,68.4054231056998,68.5930269145697,68.6511908682162,
68.8387940652687,69.0260058290388,69.2131917392048,69.4003679386567,69.5879717567479,
69.6461356634077,69.8371933145111,70.033211365758,70.229229417005),
 .UNSPECIFIED.);
#969=B_SPLINE_CURVE_WITH_KNOTS('',3,(#82735,#82736,#82737,#82738,#82739,
#82740,#82741,#82742,#82743,#82744,#82745,#82746,#82747,#82748,#82749,#82750,
#82751,#82752,#82753,#82754,#82755,#82756,#82757,#82758,#82759,#82760,#82761,
#82762,#82763,#82764,#82765,#82766,#82767,#82768,#82769,#82770,#82771,#82772,
#82773,#82774,#82775,#82776,#82777,#82778,#82779,#82780,#82781,#82782,#82783,
#82784,#82785,#82786,#82787,#82788,#82789,#82790,#82791,#82792,#82793,#82794,
#82795,#82796,#82797,#82798,#82799,#82800,#82801,#82802,#82803,#82804,#82805,
#82806,#82807,#82808,#82809,#82810,#82811,#82812,#82813,#82814,#82815,#82816,
#82817,#82818,#82819,#82820,#82821,#82822,#82823,#82824,#82825,#82826,#82827,
#82828,#82829,#82830,#82831,#82832,#82833,#82834,#82835,#82836,#82837,#82838,
#82839,#82840,#82841,#82842,#82843,#82844,#82845,#82846),.UNSPECIFIED.,
 .F.,.F.,(4,3,3,3,3,3,3,3,3,3,3,3,3,3,3,3,3,3,3,3,3,3,3,3,3,3,3,3,3,3,3,
3,3,3,3,3,3,4),(70.2292294173832,70.4351549379912,70.6410804585992,70.8286836460334,
71.0158953999048,71.203081299923,71.3902574890733,71.5778612968305,71.6360252537908,
71.8236284966211,72.0108403064174,72.1980262622685,72.3852025072517,72.5728063698176,
72.6309700489823,72.8185731289811,73.0057847759896,73.192970571568,73.3801466575811,
73.5677503659684,73.6259148441739,73.8135180610028,74.000729842834,74.1879157683528,
74.375091981605,74.5626958110086,74.6208596393654,74.8084631627783,74.9956752551974,
75.1828614923107,75.3700380180363,75.5576421554465,75.6158044345569,75.8010937918736,
75.9861285115055,76.1709869704709,76.3562168039986,76.5124147237435),
 .UNSPECIFIED.);
#970=B_SPLINE_CURVE_WITH_KNOTS('',3,(#82848,#82849,#82850,#82851,#82852,
#82853,#82854,#82855,#82856,#82857,#82858,#82859,#82860,#82861,#82862,#82863,
#82864,#82865,#82866,#82867,#82868,#82869,#82870,#82871,#82872,#82873,#82874,
#82875,#82876,#82877,#82878,#82879,#82880,#82881,#82882,#82883,#82884,#82885,
#82886,#82887,#82888,#82889,#82890,#82891,#82892,#82893,#82894,#82895,#82896,
#82897,#82898,#82899,#82900,#82901,#82902,#82903,#82904,#82905,#82906,#82907,
#82908,#82909,#82910,#82911,#82912,#82913,#82914,#82915,#82916,#82917,#82918,
#82919,#82920,#82921,#82922,#82923,#82924,#82925,#82926,#82927,#82928,#82929,
#82930,#82931,#82932,#82933,#82934,#82935,#82936,#82937,#82938,#82939,#82940,
#82941,#82942,#82943,#82944,#82945,#82946,#82947,#82948,#82949,#82950,#82951,
#82952,#82953,#82954,#82955,#82956,#82957,#82958,#82959,#82960,#82961,#82962),
 .UNSPECIFIED.,.F.,.F.,(4,3,3,3,3,3,3,3,3,3,3,3,3,3,3,3,3,3,3,3,3,3,3,3,
3,3,3,3,3,3,3,3,3,3,3,3,3,3,4),(76.5124147241846,76.6107492297485,76.7983528569055,
76.9855650396531,77.1727513466827,77.3599279305794,77.5475321081861,77.60569402494,
77.7932991932381,77.9805129465394,78.1677008422247,78.3548790267638,78.5424847929033,
78.6006388201316,78.7882363136644,78.9754423761354,79.162622674032,79.3497933073766,
79.5373917279101,79.5955836153231,79.7831914375022,79.9704077552958,80.1575980498889,
80.3447785397938,80.5323864343542,80.5905284105146,80.7781426404921,80.9653655764656,
81.152562688196,81.339750116825,81.5273649977987,81.5854732057062,81.7730367225467,
81.960208775334,82.1473555280425,82.334492852466,82.5220589147969,82.5804180008977,
82.7956000313642),.UNSPECIFIED.);
#971=B_SPLINE_CURVE_WITH_KNOTS('',3,(#82964,#82965,#82966,#82967,#82968,
#82969,#82970,#82971),.UNSPECIFIED.,.F.,.F.,(4,1,1,1,1,4),(82.7956015954281,
83.5753627960893,84.5703075912808,85.5652523864723,86.5601971816639,87.4798914339604),
 .UNSPECIFIED.);
#972=B_SPLINE_CURVE_WITH_KNOTS('',3,(#82975,#82976,#82977,#82978,#82979,
#82980,#82981),.UNSPECIFIED.,.F.,.F.,(4,1,1,1,4),(-89.5450315672385,-88.550086772047,
-87.5551419768554,-86.5601971816639,-85.773952932868),.UNSPECIFIED.);
#973=B_SPLINE_CURVE_WITH_KNOTS('',3,(#82983,#82984,#82985,#82986,#82987,
#82988,#82989,#82990,#82991,#82992,#82993,#82994,#82995,#82996,#82997,#82998,
#82999,#83000,#83001,#83002,#83003,#83004,#83005,#83006,#83007,#83008,#83009,
#83010,#83011,#83012,#83013,#83014,#83015,#83016,#83017,#83018,#83019,#83020,
#83021,#83022,#83023,#83024,#83025,#83026,#83027,#83028,#83029,#83030,#83031,
#83032,#83033,#83034,#83035,#83036,#83037,#83038,#83039,#83040,#83041,#83042,
#83043,#83044,#83045,#83046,#83047,#83048,#83049,#83050,#83051,#83052,#83053,
#83054,#83055,#83056,#83057,#83058,#83059,#83060,#83061,#83062,#83063,#83064,
#83065,#83066,#83067,#83068,#83069,#83070,#83071,#83072,#83073,#83074,#83075,
#83076,#83077,#83078,#83079,#83080,#83081,#83082,#83083,#83084,#83085,#83086,
#83087,#83088,#83089,#83090,#83091,#83092,#83093,#83094,#83095,#83096,#83097),
 .UNSPECIFIED.,.F.,.F.,(4,3,3,3,3,3,3,3,3,3,3,3,3,3,3,3,3,3,3,3,3,3,3,3,
3,3,3,3,3,3,3,3,3,3,3,3,3,3,4),(-85.773950742173,-85.5652523864724,-85.3779064829695,
-85.1909577220866,-85.0040391516937,-84.8171330902571,-84.6297986263033,
-84.5703075912808,-84.3826467392874,-84.1953769427502,-84.0081333574826,
-83.8208996375907,-83.6332395922033,-83.5753627960893,-83.3877214692297,
-83.2004701908784,-83.013243347994,-82.8260253530088,-82.6383792254152,
-82.5804180008977,-82.392852474649,-82.2056792726101,-82.0185326323522,
-81.8313961522527,-81.6438319912061,-81.5854732057062,-81.397858980688,
-81.2106360590108,-81.0234389748642,-80.8362515815531,-80.6486367465815,
-80.5905284105147,-80.4029211436349,-80.2157051380387,-80.0285147992829,
-79.8413340584639,-79.6537256147139,-79.5955836153231,-79.4907654349934),
 .UNSPECIFIED.);
#974=B_SPLINE_CURVE_WITH_KNOTS('',3,(#83099,#83100,#83101,#83102,#83103,
#83104,#83105,#83106,#83107,#83108,#83109,#83110,#83111,#83112,#83113,#83114,
#83115,#83116,#83117,#83118,#83119,#83120,#83121,#83122,#83123,#83124,#83125,
#83126,#83127,#83128,#83129,#83130,#83131,#83132,#83133,#83134,#83135,#83136,
#83137,#83138,#83139,#83140,#83141,#83142,#83143,#83144,#83145,#83146,#83147,
#83148,#83149,#83150,#83151,#83152,#83153,#83154,#83155,#83156,#83157,#83158,
#83159,#83160,#83161,#83162,#83163,#83164,#83165,#83166,#83167,#83168,#83169,
#83170,#83171,#83172,#83173,#83174,#83175,#83176,#83177,#83178,#83179,#83180,
#83181,#83182,#83183,#83184,#83185,#83186,#83187,#83188,#83189,#83190,#83191,
#83192,#83193,#83194,#83195,#83196,#83197,#83198,#83199,#83200,#83201,#83202,
#83203,#83204,#83205,#83206,#83207,#83208,#83209,#83210),.UNSPECIFIED.,
 .F.,.F.,(4,3,3,3,3,3,3,3,3,3,3,3,3,3,3,3,3,3,3,3,3,3,3,3,3,3,3,3,3,3,3,
3,3,3,3,3,3,4),(-79.4907654345562,-79.3056659286142,-79.1207476836018,-78.9359630581407,
-78.7507490396709,-78.6006388201316,-78.4130336821603,-78.2258199481935,
-78.0386320556497,-77.8514538648623,-77.6638480788338,-77.60569402494,-77.4180904691762,
-77.2308783264915,-77.0436920136003,-76.856515397198,-76.6689111486492,
-76.6107492297485,-76.4231467887123,-76.2359358006407,-76.048750682992,
-75.861575286587,-75.673972272423,-75.6158044345569,-75.4282009197706,-75.2409888326382,
-75.0538025959008,-74.8666260677027,-74.6790219236929,-74.6208596393654,
-74.4332564312801,-74.2460446543263,-74.0588587280189,-73.8716825106907,
-73.6840786724701,-73.6259148441739,-73.4167474861729,-73.2075801281719),
 .UNSPECIFIED.);
#975=B_SPLINE_CURVE_WITH_KNOTS('',3,(#83212,#83213,#83214,#83215,#83216,
#83217,#83218,#83219,#83220,#83221,#83222,#83223,#83224,#83225,#83226,#83227,
#83228,#83229,#83230,#83231,#83232,#83233,#83234,#83235,#83236,#83237,#83238,
#83239,#83240,#83241,#83242,#83243,#83244,#83245,#83246,#83247,#83248,#83249,
#83250,#83251,#83252,#83253,#83254,#83255,#83256,#83257,#83258,#83259,#83260,
#83261,#83262,#83263,#83264,#83265,#83266,#83267,#83268,#83269,#83270,#83271,
#83272,#83273,#83274,#83275,#83276,#83277,#83278,#83279,#83280,#83281,#83282,
#83283,#83284,#83285,#83286,#83287,#83288,#83289,#83290,#83291,#83292,#83293,
#83294,#83295,#83296,#83297,#83298,#83299,#83300,#83301,#83302,#83303,#83304,
#83305,#83306,#83307,#83308,#83309,#83310,#83311,#83312,#83313,#83314,#83315,
#83316,#83317,#83318,#83319,#83320,#83321,#83322,#83323),.UNSPECIFIED.,
 .F.,.F.,(4,3,3,3,3,3,3,3,3,3,3,3,3,3,3,3,3,3,3,3,3,3,3,3,3,3,3,3,3,3,3,
3,3,3,3,3,3,4),(-73.2075801278138,-73.016815520887,-72.8238927849347,-72.6309700489823,
-72.4433668079907,-72.2561549993083,-72.0689690435056,-71.8817927979529,
-71.6941889339227,-71.6360252537908,-71.4484220673553,-71.2612103140335,
-71.074024413907,-70.8868482242669,-70.6992444154695,-70.6410804585993,
-70.4534772833099,-70.2662655417254,-70.0790796540231,-69.8919034772181,
-69.7042996816319,-69.6461356634077,-69.4585324667012,-69.2713207031396,
-69.0841347929803,-68.8969585934182,-68.7093547750472,-68.6511908682162,
-68.4635876806845,-68.276375926455,-68.0891900257129,-67.9020138356261,
-67.7144100266428,-67.6562460730246,-67.4705123135506,-67.2851577710245,
-67.0997342737558,-66.9243948206342),.UNSPECIFIED.);
#976=B_SPLINE_CURVE_WITH_KNOTS('',3,(#83325,#83326,#83327,#83328,#83329,
#83330,#83331,#83332,#83333,#83334,#83335,#83336,#83337,#83338,#83339,#83340,
#83341,#83342,#83343,#83344,#83345,#83346,#83347,#83348,#83349,#83350,#83351,
#83352,#83353,#83354,#83355,#83356,#83357,#83358,#83359,#83360,#83361,#83362,
#83363,#83364,#83365,#83366,#83367,#83368,#83369,#83370,#83371,#83372,#83373,
#83374,#83375,#83376,#83377,#83378,#83379,#83380,#83381,#83382,#83383,#83384,
#83385,#83386,#83387,#83388,#83389,#83390,#83391,#83392,#83393,#83394,#83395,
#83396,#83397,#83398,#83399,#83400,#83401,#83402,#83403,#83404,#83405,#83406,
#83407,#83408,#83409,#83410,#83411,#83412,#83413,#83414,#83415,#83416,#83417,
#83418,#83419,#83420,#83421,#83422,#83423,#83424,#83425,#83426,#83427,#83428,
#83429,#83430,#83431,#83432,#83433,#83434,#83435,#83436,#83437,#83438,#83439,
#83440,#83441,#83442),.UNSPECIFIED.,.F.,.F.,(4,3,3,3,3,3,3,3,3,3,3,3,3,
3,3,3,3,3,3,3,3,3,3,3,3,3,3,3,3,3,3,3,3,3,3,3,3,3,3,4),(-66.9243948202828,
-66.6871196879193,-66.6613012778331,-66.4736980880535,-66.2864863315603,
-66.0993004285668,-65.9121242362338,-65.7245204250532,-65.6663564826416,
-65.4787532943425,-65.2915415393579,-65.1043556378908,-64.9171794470959,
-64.7295756374425,-64.67141168745,-64.4838084991056,-64.2965967440818,-64.109410842585,
-63.9222346517659,-63.734630842097,-63.6764668922585,-63.4888637035318,
-63.3016519481145,-63.1144660462139,-62.9272898549847,-62.7396860449035,
-62.681522097067,-62.4939189085714,-62.3067071533899,-62.1195212517283,
-61.9323450607403,-61.7447412508991,-61.6865773018754,-61.498974113353,
-61.3117623581451,-61.1245764564582,-60.9374002654453,-60.7497964555805,
-60.6916325066839,-60.6412095134547),.UNSPECIFIED.);
#977=B_SPLINE_CURVE_WITH_KNOTS('',3,(#83444,#83445,#83446,#83447,#83448,
#83449,#83450,#83451,#83452,#83453,#83454,#83455,#83456,#83457,#83458,#83459,
#83460,#83461,#83462,#83463,#83464,#83465,#83466,#83467,#83468,#83469,#83470,
#83471,#83472,#83473,#83474,#83475,#83476,#83477,#83478,#83479,#83480,#83481,
#83482,#83483,#83484,#83485,#83486,#83487,#83488,#83489,#83490,#83491,#83492,
#83493,#83494,#83495,#83496,#83497,#83498,#83499,#83500,#83501,#83502,#83503,
#83504,#83505,#83506,#83507,#83508,#83509,#83510,#83511,#83512,#83513,#83514,
#83515,#83516,#83517,#83518,#83519,#83520,#83521,#83522,#83523,#83524,#83525,
#83526,#83527,#83528,#83529,#83530,#83531,#83532,#83533,#83534,#83535,#83536,
#83537,#83538,#83539,#83540,#83541,#83542,#83543,#83544,#83545,#83546,#83547,
#83548,#83549,#83550,#83551,#83552,#83553,#83554,#83555),.UNSPECIFIED.,
 .F.,.F.,(4,3,3,3,3,3,3,3,3,3,3,3,3,3,3,3,3,3,3,3,3,3,3,3,3,3,3,3,3,3,3,
3,3,3,3,3,3,4),(-60.6412095131385,-60.4550710274,-60.2654751984231,-60.0797248474358,
-59.888206279464,-59.6966877114923,-59.5090845229566,-59.3218727677347,
-59.1346868660328,-58.9475106750045,-58.7599068651237,-58.7017429163008,
-58.5141397277585,-58.3269279725298,-58.1397420708213,-57.9525658797863,
-57.7649620698991,-57.7067981211093,-57.519194932561,-57.3319831773264,
-57.1447972756115,-56.9576210845701,-56.7700172746764,-56.7118533259177,
-56.5242501373747,-56.3370383821452,-56.1498524804358,-55.9626762894,-55.7750724795118,
-55.7169085307262,-55.5293053421818,-55.342093586951,-55.1549076852402,
-54.9677314942029,-54.7801276843134,-54.7219637355346,-54.5090848399423,
-54.3580242067312),.UNSPECIFIED.);
#978=B_SPLINE_CURVE_WITH_KNOTS('',3,(#83557,#83558,#83559,#83560,#83561,
#83562,#83563,#83564,#83565,#83566,#83567,#83568,#83569,#83570,#83571,#83572,
#83573,#83574,#83575,#83576,#83577,#83578,#83579,#83580,#83581,#83582,#83583,
#83584,#83585,#83586,#83587,#83588,#83589,#83590,#83591,#83592,#83593,#83594,
#83595,#83596,#83597,#83598,#83599,#83600,#83601,#83602,#83603,#83604,#83605,
#83606,#83607,#83608,#83609,#83610,#83611,#83612,#83613,#83614,#83615,#83616,
#83617,#83618,#83619,#83620,#83621,#83622,#83623,#83624,#83625,#83626,#83627,
#83628,#83629,#83630,#83631,#83632,#83633,#83634,#83635,#83636,#83637,#83638,
#83639,#83640,#83641,#83642,#83643,#83644,#83645,#83646,#83647,#83648,#83649,
#83650,#83651,#83652,#83653,#83654,#83655,#83656,#83657,#83658,#83659,#83660,
#83661,#83662,#83663,#83664,#83665,#83666,#83667,#83668,#83669,#83670,#83671),
 .UNSPECIFIED.,.F.,.F.,(4,3,3,3,3,3,3,3,3,3,3,3,3,3,3,3,3,3,3,3,3,3,3,3,
3,3,3,3,3,3,3,3,3,3,3,3,3,3,4),(-54.3580242062751,-54.1698030157393,-53.9815482560258,
-53.7928058472959,-53.7270189403431,-53.5394157517988,-53.3522039965681,
-53.1650180948574,-52.9778419038202,-52.7902380939308,-52.7320741451516,
-52.544470956607,-52.357259201376,-52.170073299665,-51.9828971086275,-51.7952932987378,
-51.73712934996,-51.5495261614154,-51.3623144061844,-51.1751285044734,-50.9879523134359,
-50.8003485035461,-50.7421845547685,-50.554581366224,-50.367369610993,-50.1801837092821,
-49.9930075182446,-49.8054037083549,-49.7472397595769,-49.5596365710323,
-49.3724248158012,-49.1852389140902,-48.9980627230527,-48.810458913163,
-48.7522949643854,-48.5652370035731,-48.3785769311802,-48.1919778865844,
-48.0748388990955),.UNSPECIFIED.);
#979=B_SPLINE_CURVE_WITH_KNOTS('',3,(#83673,#83674,#83675,#83676,#83677,
#83678,#83679,#83680,#83681,#83682,#83683,#83684,#83685,#83686,#83687,#83688,
#83689,#83690,#83691,#83692,#83693,#83694,#83695,#83696,#83697,#83698,#83699,
#83700,#83701,#83702,#83703,#83704,#83705,#83706,#83707,#83708,#83709,#83710,
#83711,#83712,#83713,#83714,#83715,#83716,#83717,#83718,#83719,#83720,#83721,
#83722,#83723,#83724,#83725,#83726,#83727,#83728,#83729,#83730,#83731,#83732,
#83733,#83734,#83735,#83736,#83737,#83738,#83739,#83740,#83741,#83742,#83743,
#83744,#83745,#83746,#83747,#83748,#83749,#83750,#83751,#83752,#83753,#83754,
#83755,#83756,#83757,#83758,#83759,#83760,#83761,#83762,#83763,#83764,#83765,
#83766,#83767,#83768,#83769,#83770,#83771,#83772,#83773,#83774,#83775,#83776,
#83777,#83778,#83779,#83780,#83781,#83782,#83783,#83784,#83785,#83786,#83787),
 .UNSPECIFIED.,.F.,.F.,(4,3,3,3,3,3,3,3,3,3,3,3,3,3,3,3,3,3,3,3,3,3,3,3,
3,3,3,3,3,3,3,3,3,3,3,3,3,3,4),(-48.0748388987013,-47.8528052031575,-47.7573501691939,
-47.5697469806493,-47.3825352254183,-47.1953493237073,-47.0081731326697,
-46.82056932278,-46.7624053740023,-46.5748021854578,-46.3875904302269,-46.200404528516,
-46.0132283374785,-45.8256245275888,-45.7674605788108,-45.5798573902662,
-45.3926456350353,-45.2054597333243,-45.0182835422868,-44.830679732397,
-44.7725157836192,-44.5849125950746,-44.3977008398437,-44.2105149381327,
-44.0233387470952,-43.8357349372054,-43.7775709884277,-43.5899677998832,
-43.4027560446523,-43.2155701429414,-43.0283939519039,-42.8407901420143,
-42.7826261932362,-42.5951562904176,-42.4080774892545,-42.221024314044,
-42.0339793110198,-41.8465084281791,-41.791653592194),.UNSPECIFIED.);
#980=B_SPLINE_CURVE_WITH_KNOTS('',3,(#83789,#83790,#83791,#83792,#83793,
#83794,#83795,#83796,#83797,#83798,#83799,#83800,#83801,#83802,#83803,#83804,
#83805,#83806,#83807,#83808,#83809,#83810,#83811,#83812,#83813,#83814,#83815,
#83816,#83817,#83818,#83819,#83820,#83821,#83822,#83823,#83824,#83825,#83826,
#83827,#83828,#83829,#83830,#83831,#83832,#83833,#83834,#83835,#83836,#83837,
#83838,#83839,#83840,#83841,#83842,#83843,#83844,#83845,#83846,#83847,#83848,
#83849,#83850,#83851,#83852,#83853,#83854,#83855,#83856,#83857,#83858,#83859,
#83860,#83861,#83862,#83863,#83864,#83865,#83866,#83867,#83868,#83869,#83870,
#83871,#83872,#83873,#83874,#83875,#83876,#83877,#83878,#83879,#83880,#83881,
#83882,#83883,#83884,#83885,#83886,#83887,#83888,#83889,#83890,#83891,#83892,
#83893,#83894,#83895,#83896,#83897,#83898,#83899,#83900,#83901,#83902,#83903),
 .UNSPECIFIED.,.F.,.F.,(4,3,3,3,3,3,3,3,3,3,3,3,3,3,3,3,3,3,3,3,3,3,3,3,
3,3,3,3,3,3,3,3,3,3,3,3,3,3,4),(-41.7916535919159,-41.6039138088844,-41.4165657069799,
-41.2292436594185,-41.0419328482664,-40.854192754235,-40.7927366028531,
-40.6051334143086,-40.4179216590777,-40.2307357573668,-40.0435595663293,
-39.8559557564396,-39.7977918076616,-39.610188619117,-39.4229768638861,
-39.2357909621751,-39.0486147711376,-38.8610109612479,-38.80284701247,-38.6152438239254,
-38.4280320686944,-38.2408461669834,-38.0536699759458,-37.8660661660561,
-37.8079022172785,-37.620299028734,-37.433087273503,-37.245901371792,-37.0587251807545,
-36.8711213708648,-36.8129574220869,-36.6253542335426,-36.4381424783119,
-36.2509565766011,-36.0637803855639,-35.8761765756744,-35.8180126268954,
-35.5941154784001,-35.5084682851079),.UNSPECIFIED.);
#981=B_SPLINE_CURVE_WITH_KNOTS('',3,(#83905,#83906,#83907,#83908,#83909,
#83910,#83911,#83912,#83913,#83914,#83915,#83916,#83917,#83918,#83919,#83920,
#83921,#83922,#83923,#83924,#83925,#83926,#83927,#83928,#83929,#83930,#83931,
#83932,#83933,#83934,#83935,#83936,#83937,#83938,#83939,#83940,#83941,#83942,
#83943,#83944,#83945,#83946,#83947,#83948,#83949,#83950,#83951,#83952,#83953,
#83954,#83955,#83956,#83957,#83958,#83959,#83960,#83961,#83962,#83963,#83964,
#83965,#83966,#83967,#83968,#83969,#83970,#83971,#83972,#83973,#83974,#83975,
#83976,#83977,#83978,#83979,#83980,#83981,#83982,#83983,#83984,#83985,#83986,
#83987,#83988,#83989,#83990,#83991,#83992,#83993,#83994,#83995,#83996,#83997,
#83998,#83999,#84000,#84001,#84002,#84003,#84004,#84005,#84006,#84007,#84008,
#84009,#84010,#84011,#84012,#84013,#84014,#84015,#84016,#84017,#84018,#84019),
 .UNSPECIFIED.,.F.,.F.,(4,3,3,3,3,3,3,3,3,3,3,3,3,3,3,3,3,3,3,3,3,3,3,3,
3,3,3,3,3,3,3,3,3,3,3,3,3,3,4),(-35.5084682847363,-35.3220367280429,-35.1356792786183,
-34.9488651523034,-34.8230678317039,-34.6354646431595,-34.4482528879287,
-34.2610669862178,-34.0738907951805,-33.8862869852908,-33.8281230365123,
-33.6405198479693,-33.45330809274,-33.2661221910306,-33.0789459999947,-32.8913421901065,
-32.8331782413208,-32.6455750527723,-32.4583632975375,-32.2711773958227,
-32.0840012047815,-31.896397394888,-31.8382334461292,-31.6506302575872,
-31.4634185023586,-31.27623260065,-31.0890564096147,-30.9014525997272,-30.8432886509377,
-30.6556854624021,-30.4684737071803,-30.2812878054784,-30.09411161445,-29.9065078045693,
-29.8483438557462,-29.6592690772485,-29.4706263248811,-29.2821819130397,
-29.2252829775567),.UNSPECIFIED.);
#982=B_SPLINE_CURVE_WITH_KNOTS('',3,(#84021,#84022,#84023,#84024,#84025,
#84026,#84027,#84028,#84029,#84030,#84031,#84032,#84033,#84034,#84035,#84036,
#84037,#84038,#84039,#84040,#84041,#84042,#84043,#84044,#84045,#84046,#84047,
#84048,#84049,#84050,#84051,#84052,#84053,#84054,#84055,#84056,#84057,#84058,
#84059,#84060,#84061,#84062,#84063,#84064,#84065,#84066,#84067,#84068,#84069,
#84070,#84071,#84072,#84073,#84074,#84075,#84076,#84077,#84078,#84079,#84080,
#84081,#84082,#84083,#84084,#84085,#84086,#84087,#84088,#84089,#84090,#84091,
#84092,#84093,#84094,#84095,#84096,#84097,#84098,#84099,#84100,#84101,#84102,
#84103,#84104,#84105,#84106,#84107,#84108,#84109,#84110,#84111,#84112,#84113,
#84114,#84115,#84116,#84117,#84118,#84119,#84120,#84121,#84122,#84123,#84124,
#84125,#84126,#84127,#84128,#84129,#84130,#84131,#84132),.UNSPECIFIED.,
 .F.,.F.,(4,3,3,3,3,3,3,3,3,3,3,3,3,3,3,3,3,3,3,3,3,3,3,3,3,3,3,3,3,3,3,
3,3,3,3,3,3,4),(-29.2252829771043,-29.0137239014305,-28.8533990605546,-28.6657958720351,
-28.4785841168289,-28.2913982151417,-28.1042220241277,-27.9166182142602,
-27.8584542653631,-27.6708510768672,-27.4836393216855,-27.2964534200241,
-27.1092772290363,-26.9216734191956,-26.8635094701716,-26.6759062814358,
-26.4886945260133,-26.3015086241134,-26.1143324328882,-25.9267286228161,
-25.86856467498,-25.680961486656,-25.4937497316436,-25.306563830145,-25.1193876393166,
-24.9317838296272,-24.8736198797885,-24.6860166914801,-24.4988049364903,
-24.311619035024,-24.1244428442335,-23.9368390345895,-23.8786750845969,
-23.6926863022266,-23.5050391443534,-23.3194703520081,-23.1307840113709,
-22.9420976707337),.UNSPECIFIED.);
#983=B_SPLINE_CURVE_WITH_KNOTS('',3,(#84134,#84135,#84136,#84137,#84138,
#84139,#84140,#84141,#84142,#84143,#84144,#84145,#84146,#84147,#84148,#84149,
#84150,#84151,#84152,#84153,#84154,#84155,#84156,#84157,#84158,#84159,#84160,
#84161,#84162,#84163,#84164,#84165,#84166,#84167,#84168,#84169,#84170,#84171,
#84172,#84173,#84174,#84175,#84176,#84177,#84178,#84179,#84180,#84181,#84182,
#84183,#84184,#84185,#84186,#84187,#84188,#84189,#84190,#84191,#84192,#84193,
#84194,#84195,#84196,#84197,#84198,#84199,#84200,#84201,#84202,#84203,#84204,
#84205,#84206,#84207,#84208,#84209,#84210,#84211,#84212,#84213,#84214,#84215,
#84216,#84217,#84218,#84219,#84220,#84221,#84222,#84223,#84224,#84225,#84226,
#84227,#84228,#84229,#84230,#84231,#84232,#84233,#84234,#84235,#84236,#84237,
#84238,#84239,#84240,#84241,#84242,#84243,#84244,#84245,#84246,#84247,#84248,
#84249,#84250,#84251),.UNSPECIFIED.,.F.,.F.,(4,3,3,3,3,3,3,3,3,3,3,3,3,
3,3,3,3,3,3,3,3,3,3,3,3,3,3,3,3,3,3,3,3,3,3,3,3,3,3,4),(-22.9420976703771,
-22.8837302894054,-22.6961271026793,-22.508915349255,-22.3217294493065,
-22.1345532600077,-21.9469494517905,-21.8887854942139,-21.7011823065751,
-21.5139705522857,-21.3267846515529,-21.1396084615158,-20.9520046526399,
-20.8938406990223,-20.7062375020042,-20.5190257382684,-20.3318398281365,
-20.1446636287185,-19.9570598106604,-19.8988959038308,-19.7112927295762,
-19.52408098857,-19.336895100777,-19.1497189234932,-18.9621151268684,-18.9039511086392,
-18.7163479211876,-18.5291361672979,-18.3419502672604,-18.1547740780903,
-17.9671702703128,-17.9090063134477,-17.7214030708108,-17.5341912612088,
-17.3470053055504,-17.1598290607591,-16.9722251983805,-16.9140615182562,
-16.6739534983264,-16.6589123634645),.UNSPECIFIED.);
#984=B_SPLINE_CURVE_WITH_KNOTS('',3,(#84253,#84254,#84255,#84256,#84257,
#84258,#84259,#84260,#84261,#84262,#84263,#84264,#84265,#84266,#84267,#84268,
#84269,#84270,#84271,#84272,#84273,#84274,#84275,#84276,#84277,#84278,#84279,
#84280,#84281,#84282,#84283,#84284,#84285,#84286,#84287,#84288,#84289,#84290,
#84291,#84292,#84293,#84294,#84295,#84296,#84297,#84298,#84299,#84300,#84301,
#84302,#84303,#84304,#84305,#84306,#84307,#84308,#84309,#84310,#84311,#84312,
#84313,#84314,#84315,#84316,#84317,#84318,#84319,#84320,#84321,#84322,#84323,
#84324,#84325,#84326,#84327,#84328,#84329,#84330,#84331,#84332,#84333,#84334,
#84335,#84336,#84337,#84338,#84339,#84340,#84341,#84342,#84343,#84344,#84345,
#84346,#84347,#84348,#84349,#84350,#84351,#84352,#84353,#84354,#84355,#84356,
#84357,#84358,#84359,#84360,#84361,#84362,#84363,#84364),.UNSPECIFIED.,
 .F.,.F.,(4,3,3,3,3,3,3,3,3,3,3,3,3,3,3,3,3,3,3,3,3,3,3,3,3,3,3,3,3,3,3,
3,3,3,3,3,3,4),(-16.6589123631975,-16.4736069552956,-16.2884618531051,-16.1028684349565,
-15.9191167230646,-15.7315135062259,-15.54430172438,-15.3571157988396,-15.169939585562,
-14.9823357561277,-14.9241719278731,-14.7365684055012,-14.5493563141293,
-14.3621700780567,-14.1749935533688,-13.9873894169731,-13.9292271326815,
-13.7416247391222,-13.5544137775851,-13.3672286557758,-13.1800532374019,
-12.9924501755822,-12.93428233749,-12.7466787107606,-12.5594665284143,-12.3722802217423,
-12.1851036381787,-11.9974994608632,-11.9393375422985,-11.7517323793176,
-11.5645186313735,-11.3773307410216,-11.1901525618073,-11.0025468008832,
-10.9443927471069,-10.7525085527175,-10.56110757904,-10.3757270560179),
 .UNSPECIFIED.);
#985=B_SPLINE_CURVE_WITH_KNOTS('',3,(#84365,#84366,#84367,#84368,#84369,
#84370,#84371,#84372,#84373,#84374),.UNSPECIFIED.,.F.,.F.,(4,1,1,1,1,1,
1,4),(-10.3757218525839,-9.94944795191539,-8.95450315672385,-7.95955836153231,
-6.96461356634077,-5.96966877114923,-4.97472397595769,-4.09254174883834),
 .UNSPECIFIED.);
#986=B_SPLINE_CURVE_WITH_KNOTS('',3,(#84377,#84378,#84379,#84380,#84381,
#84382,#84383),.UNSPECIFIED.,.F.,.F.,(4,1,1,1,4),(95.0999839528908,95.1907843151998,
96.1857291103914,97.1806739055829,97.3893722612836),.UNSPECIFIED.);
#987=B_SPLINE_CURVE_WITH_KNOTS('',3,(#84385,#84386,#84387,#84388,#84389,
#84390,#84391,#84392,#84393,#84394,#84395,#84396,#84397,#84398,#84399,#84400,
#84401,#84402,#84403,#84404,#84405,#84406,#84407,#84408,#84409,#84410,#84411,
#84412),.UNSPECIFIED.,.F.,.F.,(4,3,3,3,3,3,3,3,3,4),(97.3893724044164,97.5859339785059,
97.7815995754182,97.9786091380963,98.1756187007744,98.3723125568378,98.5687414387062,
98.7649953873722,98.9616717847817,99.0952857495152),.UNSPECIFIED.);
#988=B_SPLINE_CURVE_WITH_KNOTS('',3,(#84416,#84417,#84418,#84419,#84420,
#84421,#84422,#84423,#84424,#84425,#84426,#84427,#84428,#84429,#84430,#84431,
#84432,#84433,#84434,#84435),.UNSPECIFIED.,.F.,.F.,(4,2,2,2,2,2,2,2,2,4),
(0.000182933856833843,0.00211949330641253,0.00426999235183267,0.00836840074118015,
0.0151774046226676,0.0366484253322754,0.0654492646296514,0.0700723566601802,
0.0716586735729506,0.0730520430944184),.UNSPECIFIED.);
#989=B_SPLINE_CURVE_WITH_KNOTS('',3,(#84436,#84437,#84438,#84439,#84440,
#84441,#84442,#84443,#84444,#84445,#84446,#84447,#84448,#84449,#84450,#84451,
#84452,#84453,#84454,#84455,#84456,#84457,#84458,#84459,#84460,#84461,#84462,
#84463,#84464,#84465,#84466,#84467,#84468,#84469,#84470,#84471,#84472),
 .UNSPECIFIED.,.F.,.F.,(4,3,3,3,3,3,3,3,3,3,3,3,4),(95.1011120778127,95.2997246445013,
95.4981796586158,95.6971224053591,95.8657288995951,96.062179531293,96.2618030721664,
96.4578350224103,96.6592543585984,96.8606736947866,97.075180245871,97.2884928513503,
97.3893722612836),.UNSPECIFIED.);
#990=B_SPLINE_CURVE_WITH_KNOTS('',3,(#84845,#84846,#84847,#84848,#84849,
#84850,#84851,#84852,#84853,#84854,#84855,#84856,#84857,#84858,#84859,#84860,
#84861,#84862,#84863,#84864,#84865,#84866,#84867,#84868,#84869,#84870,#84871,
#84872,#84873,#84874,#84875,#84876,#84877,#84878,#84879,#84880,#84881,#84882,
#84883,#84884,#84885,#84886,#84887,#84888,#84889,#84890,#84891,#84892,#84893,
#84894,#84895,#84896,#84897,#84898,#84899),.UNSPECIFIED.,.F.,.F.,(4,3,3,
3,3,3,3,3,3,3,3,3,3,3,3,3,3,3,4),(-0.364609086663937,-0.349955759834691,
-0.322148792467856,-0.301818556032635,-0.269021332414628,-0.255281697682016,
-0.220959067372234,-0.202353981127163,-0.188377705920309,-0.186636437062452,
-0.165752269796004,-0.142062715941464,-0.129304435383701,-0.117755883775514,
-0.0883169128316359,-0.069851718219777,-0.0532071563521246,-0.020916945320546,
0.),.UNSPECIFIED.);
#991=B_SPLINE_CURVE_WITH_KNOTS('',3,(#84900,#84901,#84902,#84903,#84904,
#84905,#84906,#84907,#84908,#84909,#84910,#84911,#84912,#84913,#84914,#84915,
#84916,#84917,#84918,#84919,#84920,#84921,#84922,#84923,#84924,#84925,#84926,
#84927,#84928,#84929,#84930,#84931,#84932,#84933,#84934,#84935,#84936,#84937,
#84938,#84939,#84940,#84941,#84942,#84943,#84944,#84945,#84946,#84947,#84948,
#84949,#84950,#84951),.UNSPECIFIED.,.F.,.F.,(4,3,3,3,3,3,3,3,3,3,3,3,3,
3,3,3,3,4),(-0.366397579005849,-0.354487143711378,-0.327235825426289,-0.312257563612696,
-0.287192971194593,-0.271636001607225,-0.236484251747428,-0.218731998635388,
-0.204568081622605,-0.186662998246843,-0.163330123465988,-0.147055277061879,
-0.13340270893607,-0.100052031702053,-0.080940924208064,-0.0644514768169998,
-0.0259839405418483,-2.77882917038371E-15),.UNSPECIFIED.);
#992=B_SPLINE_CURVE_WITH_KNOTS('',3,(#84957,#84958,#84959,#84960,#84961,
#84962,#84963,#84964,#84965,#84966,#84967,#84968,#84969,#84970,#84971,#84972,
#84973,#84974,#84975,#84976,#84977,#84978,#84979,#84980,#84981,#84982,#84983,
#84984,#84985,#84986,#84987,#84988,#84989,#84990,#84991,#84992,#84993,#84994,
#84995,#84996,#84997,#84998,#84999,#85000,#85001,#85002,#85003,#85004,#85005,
#85006,#85007,#85008,#85009,#85010,#85011),.UNSPECIFIED.,.F.,.F.,(4,3,3,
3,3,3,3,3,3,3,3,3,3,3,3,3,3,3,4),(-0.361287482968457,-0.349955759834647,
-0.323048888644992,-0.302534193252467,-0.279099431199845,-0.265528167404287,
-0.252514851361878,-0.222201740894643,-0.202919079809183,-0.184570412842509,
-0.165752269795994,-0.142063101534203,-0.129304205568179,-0.117754438538821,
-0.0883158289041158,-0.0698511326658658,-0.0532073016903481,-0.0209171118703778,
0.),.UNSPECIFIED.);
#993=B_SPLINE_CURVE_WITH_KNOTS('',3,(#85384,#85385,#85386,#85387,#85388,
#85389,#85390,#85391,#85392,#85393,#85394,#85395,#85396,#85397,#85398,#85399,
#85400,#85401,#85402,#85403,#85404,#85405,#85406,#85407,#85408,#85409,#85410,
#85411,#85412,#85413,#85414,#85415,#85416,#85417,#85418,#85419,#85420,#85421,
#85422,#85423,#85424,#85425,#85426,#85427,#85428,#85429,#85430,#85431,#85432,
#85433,#85434,#85435),.UNSPECIFIED.,.F.,.F.,(4,3,3,3,3,3,3,3,3,3,3,3,3,
3,3,3,3,4),(-0.366397579005855,-0.354487143711385,-0.327235824669574,-0.312257556235388,
-0.287192226768709,-0.271635974620829,-0.23648422270589,-0.218732050894258,
-0.204568071899735,-0.186662998246842,-0.163330123465987,-0.147055270097115,
-0.133402728476446,-0.100052046357334,-0.0809409309648167,-0.0644514752458169,
-0.0259839471903043,0.),.UNSPECIFIED.);
#994=B_SPLINE_CURVE_WITH_KNOTS('',3,(#85436,#85437,#85438,#85439),
 .UNSPECIFIED.,.F.,.F.,(4,4),(0.,0.00337788989814126),.UNSPECIFIED.);
#1177=PLANE('',#10809);
#1178=PLANE('',#10842);
#1179=PLANE('',#10843);
#1180=PLANE('',#10844);
#1181=PLANE('',#10845);
#1182=PLANE('',#10846);
#1183=PLANE('',#10847);
#1184=PLANE('',#10848);
#1185=PLANE('',#10849);
#1186=PLANE('',#10852);
#1662=LINE('',#77894,#2198);
#1663=LINE('',#77978,#2199);
#1664=LINE('',#78246,#2200);
#1665=LINE('',#78539,#2201);
#1666=LINE('',#78861,#2202);
#1667=LINE('',#79158,#2203);
#1668=LINE('',#79481,#2204);
#1669=LINE('',#79786,#2205);
#1670=LINE('',#80093,#2206);
#1671=LINE('',#80394,#2207);
#1672=LINE('',#80721,#2208);
#1673=LINE('',#81016,#2209);
#1674=LINE('',#81332,#2210);
#1675=LINE('',#81634,#2211);
#1676=LINE('',#85509,#2212);
#1677=LINE('',#85513,#2213);
#1678=LINE('',#85515,#2214);
#1679=LINE('',#85516,#2215);
#1680=LINE('',#85519,#2216);
#1681=LINE('',#85520,#2217);
#1682=LINE('',#85523,#2218);
#1683=LINE('',#85524,#2219);
#1684=LINE('',#85527,#2220);
#1685=LINE('',#85528,#2221);
#1686=LINE('',#85531,#2222);
#1687=LINE('',#85532,#2223);
#1688=LINE('',#85534,#2224);
#1689=LINE('',#85540,#2225);
#1690=LINE('',#85545,#2226);
#2198=VECTOR('',#12806,0.15555);
#2199=VECTOR('',#12811,0.15555);
#2200=VECTOR('',#12814,0.15555);
#2201=VECTOR('',#12817,0.15555);
#2202=VECTOR('',#12820,0.15555);
#2203=VECTOR('',#12823,0.15555);
#2204=VECTOR('',#12826,0.15555);
#2205=VECTOR('',#12829,0.15555);
#2206=VECTOR('',#12832,0.15555);
#2207=VECTOR('',#12835,0.15555);
#2208=VECTOR('',#12838,0.15555);
#2209=VECTOR('',#12841,0.15555);
#2210=VECTOR('',#12844,0.15555);
#2211=VECTOR('',#12847,0.15555);
#2212=VECTOR('',#12922,0.06125);
#2213=VECTOR('',#12927,1.);
#2214=VECTOR('',#12928,1.);
#2215=VECTOR('',#12929,1.);
#2216=VECTOR('',#12932,1.);
#2217=VECTOR('',#12933,1.);
#2218=VECTOR('',#12936,1.);
#2219=VECTOR('',#12937,1.);
#2220=VECTOR('',#12940,1.);
#2221=VECTOR('',#12941,1.);
#2222=VECTOR('',#12944,1.);
#2223=VECTOR('',#12945,1.);
#2224=VECTOR('',#12948,1.);
#2225=VECTOR('',#12957,0.185);
#2226=VECTOR('',#12964,0.38);
#2365=CYLINDRICAL_SURFACE('',#10789,0.15555);
#2366=CYLINDRICAL_SURFACE('',#10791,0.15555);
#2367=CYLINDRICAL_SURFACE('',#10792,0.15555);
#2368=CYLINDRICAL_SURFACE('',#10793,0.15555);
#2369=CYLINDRICAL_SURFACE('',#10794,0.15555);
#2370=CYLINDRICAL_SURFACE('',#10795,0.15555);
#2371=CYLINDRICAL_SURFACE('',#10796,0.15555);
#2372=CYLINDRICAL_SURFACE('',#10797,0.15555);
#2373=CYLINDRICAL_SURFACE('',#10798,0.15555);
#2374=CYLINDRICAL_SURFACE('',#10799,0.15555);
#2375=CYLINDRICAL_SURFACE('',#10800,0.15555);
#2376=CYLINDRICAL_SURFACE('',#10801,0.15555);
#2377=CYLINDRICAL_SURFACE('',#10802,0.15555);
#2378=CYLINDRICAL_SURFACE('',#10803,0.15555);
#2379=CYLINDRICAL_SURFACE('',#10804,0.1954);
#2380=CYLINDRICAL_SURFACE('',#10807,0.15555);
#2381=CYLINDRICAL_SURFACE('',#10854,0.38);
#2833=FACE_OUTER_BOUND('',#3421,.T.);
#2834=FACE_OUTER_BOUND('',#3422,.T.);
#2835=FACE_OUTER_BOUND('',#3423,.T.);
#2836=FACE_OUTER_BOUND('',#3424,.T.);
#2837=FACE_OUTER_BOUND('',#3425,.T.);
#2838=FACE_OUTER_BOUND('',#3426,.T.);
#2839=FACE_OUTER_BOUND('',#3427,.T.);
#2840=FACE_OUTER_BOUND('',#3428,.T.);
#2841=FACE_OUTER_BOUND('',#3429,.T.);
#2842=FACE_OUTER_BOUND('',#3430,.T.);
#2843=FACE_OUTER_BOUND('',#3431,.T.);
#2844=FACE_OUTER_BOUND('',#3432,.T.);
#2845=FACE_OUTER_BOUND('',#3433,.T.);
#2846=FACE_OUTER_BOUND('',#3434,.T.);
#2847=FACE_OUTER_BOUND('',#3435,.T.);
#2848=FACE_OUTER_BOUND('',#3436,.T.);
#2849=FACE_OUTER_BOUND('',#3437,.T.);
#2850=FACE_OUTER_BOUND('',#3438,.T.);
#2851=FACE_OUTER_BOUND('',#3439,.T.);
#2852=FACE_OUTER_BOUND('',#3440,.T.);
#2853=FACE_OUTER_BOUND('',#3441,.T.);
#2854=FACE_OUTER_BOUND('',#3442,.T.);
#2855=FACE_OUTER_BOUND('',#3443,.T.);
#2856=FACE_OUTER_BOUND('',#3444,.T.);
#2857=FACE_OUTER_BOUND('',#3445,.T.);
#2858=FACE_OUTER_BOUND('',#3446,.T.);
#2859=FACE_OUTER_BOUND('',#3447,.T.);
#2860=FACE_OUTER_BOUND('',#3448,.T.);
#2861=FACE_OUTER_BOUND('',#3449,.T.);
#2862=FACE_OUTER_BOUND('',#3450,.T.);
#2863=FACE_OUTER_BOUND('',#3451,.T.);
#2864=FACE_OUTER_BOUND('',#3452,.T.);
#2865=FACE_OUTER_BOUND('',#3453,.T.);
#2866=FACE_OUTER_BOUND('',#3454,.T.);
#2867=FACE_OUTER_BOUND('',#3456,.T.);
#2868=FACE_OUTER_BOUND('',#3457,.T.);
#2869=FACE_OUTER_BOUND('',#3458,.T.);
#2870=FACE_OUTER_BOUND('',#3460,.T.);
#3421=EDGE_LOOP('',(#8903,#8904,#8905,#8906));
#3422=EDGE_LOOP('',(#8907,#8908,#8909,#8910,#8911,#8912));
#3423=EDGE_LOOP('',(#8913,#8914,#8915,#8916,#8917));
#3424=EDGE_LOOP('',(#8918,#8919,#8920,#8921,#8922,#8923));
#3425=EDGE_LOOP('',(#8924,#8925,#8926,#8927,#8928));
#3426=EDGE_LOOP('',(#8929,#8930,#8931,#8932,#8933,#8934));
#3427=EDGE_LOOP('',(#8935,#8936,#8937,#8938,#8939));
#3428=EDGE_LOOP('',(#8940,#8941,#8942,#8943,#8944,#8945));
#3429=EDGE_LOOP('',(#8946,#8947,#8948,#8949,#8950));
#3430=EDGE_LOOP('',(#8951,#8952,#8953,#8954,#8955,#8956));
#3431=EDGE_LOOP('',(#8957,#8958,#8959,#8960,#8961));
#3432=EDGE_LOOP('',(#8962,#8963,#8964,#8965,#8966,#8967));
#3433=EDGE_LOOP('',(#8968,#8969,#8970,#8971,#8972));
#3434=EDGE_LOOP('',(#8973,#8974,#8975,#8976,#8977,#8978));
#3435=EDGE_LOOP('',(#8979,#8980,#8981,#8982,#8983,#8984,#8985,#8986,#8987,
#8988,#8989,#8990,#8991,#8992,#8993,#8994,#8995,#8996,#8997,#8998,#8999,
#9000,#9001,#9002,#9003,#9004,#9005,#9006,#9007,#9008,#9009,#9010));
#3436=EDGE_LOOP('',(#9011,#9012,#9013,#9014,#9015,#9016));
#3437=EDGE_LOOP('',(#9017,#9018,#9019,#9020,#9021,#9022,#9023,#9024,#9025,
#9026,#9027,#9028,#9029,#9030,#9031,#9032,#9033,#9034,#9035,#9036,#9037,
#9038,#9039,#9040,#9041,#9042,#9043,#9044,#9045,#9046,#9047,#9048,#9049,
#9050,#9051,#9052,#9053,#9054,#9055,#9056,#9057,#9058,#9059,#9060,#9061,
#9062));
#3438=EDGE_LOOP('',(#9063,#9064,#9065,#9066,#9067));
#3439=EDGE_LOOP('',(#9068,#9069,#9070,#9071,#9072,#9073,#9074,#9075,#9076,
#9077,#9078,#9079,#9080,#9081,#9082,#9083,#9084,#9085,#9086,#9087,#9088,
#9089,#9090,#9091,#9092,#9093,#9094,#9095,#9096,#9097,#9098,#9099,#9100,
#9101,#9102,#9103,#9104,#9105,#9106,#9107,#9108));
#3440=EDGE_LOOP('',(#9109,#9110));
#3441=EDGE_LOOP('',(#9111,#9112));
#3442=EDGE_LOOP('',(#9113,#9114));
#3443=EDGE_LOOP('',(#9115,#9116));
#3444=EDGE_LOOP('',(#9117,#9118,#9119));
#3445=EDGE_LOOP('',(#9120,#9121));
#3446=EDGE_LOOP('',(#9122,#9123,#9124,#9125,#9126,#9127,#9128,#9129,#9130,
#9131,#9132,#9133,#9134,#9135,#9136,#9137,#9138,#9139,#9140,#9141,#9142,
#9143));
#3447=EDGE_LOOP('',(#9144,#9145,#9146));
#3448=EDGE_LOOP('',(#9147,#9148,#9149,#9150,#9151,#9152));
#3449=EDGE_LOOP('',(#9153,#9154,#9155,#9156,#9157,#9158));
#3450=EDGE_LOOP('',(#9159,#9160,#9161,#9162,#9163,#9164));
#3451=EDGE_LOOP('',(#9165,#9166,#9167,#9168,#9169,#9170));
#3452=EDGE_LOOP('',(#9171,#9172,#9173,#9174,#9175,#9176));
#3453=EDGE_LOOP('',(#9177,#9178,#9179,#9180,#9181,#9182));
#3454=EDGE_LOOP('',(#9183,#9184,#9185,#9186,#9187,#9188));
#3455=EDGE_LOOP('',(#9189));
#3456=EDGE_LOOP('',(#9190));
#3457=EDGE_LOOP('',(#9191,#9192,#9193,#9194,#9195,#9196,#9197));
#3458=EDGE_LOOP('',(#9198));
#3459=EDGE_LOOP('',(#9199,#9200,#9201,#9202));
#3460=EDGE_LOOP('',(#9203,#9204,#9205,#9206));
#3825=CIRCLE('',#10790,0.15555);
#3826=CIRCLE('',#10805,0.1954);
#3827=CIRCLE('',#10806,0.1954);
#3828=CIRCLE('',#10808,0.15555);
#3829=CIRCLE('',#10810,0.1954);
#3830=CIRCLE('',#10811,0.1954);
#3831=CIRCLE('',#10813,0.131954512102672);
#3832=CIRCLE('',#10815,0.131954512102672);
#3833=CIRCLE('',#10817,0.131954512102672);
#3834=CIRCLE('',#10819,0.131954512102672);
#3835=CIRCLE('',#10821,0.131954512102672);
#3836=CIRCLE('',#10822,0.131954512102672);
#3837=CIRCLE('',#10824,0.131954512102672);
#3838=CIRCLE('',#10826,0.475);
#3839=CIRCLE('',#10827,0.38);
#3840=CIRCLE('',#10828,0.458257569495584);
#3841=CIRCLE('',#10829,0.458257569495584);
#3842=CIRCLE('',#10830,0.458257569495584);
#3843=CIRCLE('',#10831,0.458257569495584);
#3844=CIRCLE('',#10832,0.458257569495584);
#3845=CIRCLE('',#10833,0.458257569495584);
#3846=CIRCLE('',#10834,0.458257569495584);
#3847=CIRCLE('',#10835,0.458257569495584);
#3848=CIRCLE('',#10836,0.458257569495584);
#3849=CIRCLE('',#10837,0.458257569495584);
#3850=CIRCLE('',#10838,0.458257569495584);
#3851=CIRCLE('',#10839,0.458257569495584);
#3852=CIRCLE('',#10841,0.120858028271594);
#3853=CIRCLE('',#10850,0.17);
#3854=CIRCLE('',#10853,0.38);
#4761=VERTEX_POINT('',#77892);
#4762=VERTEX_POINT('',#77893);
#4763=VERTEX_POINT('',#77895);
#4764=VERTEX_POINT('',#77945);
#4765=VERTEX_POINT('',#77976);
#4766=VERTEX_POINT('',#77977);
#4767=VERTEX_POINT('',#77979);
#4768=VERTEX_POINT('',#78081);
#4769=VERTEX_POINT('',#78244);
#4770=VERTEX_POINT('',#78245);
#4771=VERTEX_POINT('',#78247);
#4772=VERTEX_POINT('',#78537);
#4773=VERTEX_POINT('',#78538);
#4774=VERTEX_POINT('',#78540);
#4775=VERTEX_POINT('',#78645);
#4776=VERTEX_POINT('',#78859);
#4777=VERTEX_POINT('',#78860);
#4778=VERTEX_POINT('',#78862);
#4779=VERTEX_POINT('',#79156);
#4780=VERTEX_POINT('',#79157);
#4781=VERTEX_POINT('',#79159);
#4782=VERTEX_POINT('',#79261);
#4783=VERTEX_POINT('',#79479);
#4784=VERTEX_POINT('',#79480);
#4785=VERTEX_POINT('',#79482);
#4786=VERTEX_POINT('',#79784);
#4787=VERTEX_POINT('',#79785);
#4788=VERTEX_POINT('',#79787);
#4789=VERTEX_POINT('',#79889);
#4790=VERTEX_POINT('',#80091);
#4791=VERTEX_POINT('',#80092);
#4792=VERTEX_POINT('',#80094);
#4793=VERTEX_POINT('',#80392);
#4794=VERTEX_POINT('',#80393);
#4795=VERTEX_POINT('',#80395);
#4796=VERTEX_POINT('',#80497);
#4797=VERTEX_POINT('',#80719);
#4798=VERTEX_POINT('',#80720);
#4799=VERTEX_POINT('',#80722);
#4800=VERTEX_POINT('',#81014);
#4801=VERTEX_POINT('',#81015);
#4802=VERTEX_POINT('',#81017);
#4803=VERTEX_POINT('',#81116);
#4804=VERTEX_POINT('',#81330);
#4805=VERTEX_POINT('',#81331);
#4806=VERTEX_POINT('',#81333);
#4807=VERTEX_POINT('',#81632);
#4808=VERTEX_POINT('',#81633);
#4809=VERTEX_POINT('',#81635);
#4810=VERTEX_POINT('',#81737);
#4811=VERTEX_POINT('',#81861);
#4812=VERTEX_POINT('',#81862);
#4813=VERTEX_POINT('',#81869);
#4814=VERTEX_POINT('',#81871);
#4815=VERTEX_POINT('',#81877);
#4816=VERTEX_POINT('',#81993);
#4817=VERTEX_POINT('',#82004);
#4818=VERTEX_POINT('',#82016);
#4819=VERTEX_POINT('',#82027);
#4820=VERTEX_POINT('',#82038);
#4821=VERTEX_POINT('',#82157);
#4822=VERTEX_POINT('',#82273);
#4823=VERTEX_POINT('',#82389);
#4824=VERTEX_POINT('',#82502);
#4825=VERTEX_POINT('',#82621);
#4826=VERTEX_POINT('',#82734);
#4827=VERTEX_POINT('',#82847);
#4828=VERTEX_POINT('',#82963);
#4829=VERTEX_POINT('',#82972);
#4830=VERTEX_POINT('',#82974);
#4831=VERTEX_POINT('',#82982);
#4832=VERTEX_POINT('',#83098);
#4833=VERTEX_POINT('',#83211);
#4834=VERTEX_POINT('',#83324);
#4835=VERTEX_POINT('',#83443);
#4836=VERTEX_POINT('',#83556);
#4837=VERTEX_POINT('',#83672);
#4838=VERTEX_POINT('',#83788);
#4839=VERTEX_POINT('',#83904);
#4840=VERTEX_POINT('',#84020);
#4841=VERTEX_POINT('',#84133);
#4842=VERTEX_POINT('',#84252);
#4843=VERTEX_POINT('',#84376);
#4844=VERTEX_POINT('',#84384);
#4845=VERTEX_POINT('',#84413);
#4846=VERTEX_POINT('',#84415);
#4847=VERTEX_POINT('',#84953);
#4848=VERTEX_POINT('',#84955);
#4849=VERTEX_POINT('',#85441);
#4850=VERTEX_POINT('',#85442);
#4851=VERTEX_POINT('',#85448);
#4852=VERTEX_POINT('',#85449);
#4853=VERTEX_POINT('',#85455);
#4854=VERTEX_POINT('',#85456);
#4855=VERTEX_POINT('',#85462);
#4856=VERTEX_POINT('',#85463);
#4857=VERTEX_POINT('',#85469);
#4858=VERTEX_POINT('',#85470);
#4859=VERTEX_POINT('',#85474);
#4860=VERTEX_POINT('',#85478);
#4861=VERTEX_POINT('',#85479);
#4862=VERTEX_POINT('',#85485);
#4863=VERTEX_POINT('',#85488);
#4864=VERTEX_POINT('',#85491);
#4865=VERTEX_POINT('',#85494);
#4866=VERTEX_POINT('',#85497);
#4867=VERTEX_POINT('',#85500);
#4868=VERTEX_POINT('',#85503);
#4869=VERTEX_POINT('',#85507);
#4870=VERTEX_POINT('',#85508);
#4871=VERTEX_POINT('',#85512);
#4872=VERTEX_POINT('',#85514);
#4873=VERTEX_POINT('',#85518);
#4874=VERTEX_POINT('',#85522);
#4875=VERTEX_POINT('',#85526);
#4876=VERTEX_POINT('',#85530);
#4877=VERTEX_POINT('',#85537);
#4878=VERTEX_POINT('',#85542);
#6179=EDGE_CURVE('',#4761,#4762,#1662,.T.);
#6180=EDGE_CURVE('',#4763,#4761,#908,.T.);
#6181=EDGE_CURVE('',#4764,#4763,#3825,.T.);
#6182=EDGE_CURVE('',#4764,#4762,#909,.T.);
#6183=EDGE_CURVE('',#4765,#4766,#1663,.T.);
#6184=EDGE_CURVE('',#4767,#4765,#910,.T.);
#6185=EDGE_CURVE('',#4761,#4767,#911,.T.);
#6186=EDGE_CURVE('',#4762,#4768,#912,.T.);
#6187=EDGE_CURVE('',#4768,#4766,#913,.T.);
#6188=EDGE_CURVE('',#4769,#4770,#1664,.T.);
#6189=EDGE_CURVE('',#4771,#4769,#914,.T.);
#6190=EDGE_CURVE('',#4765,#4771,#915,.T.);
#6191=EDGE_CURVE('',#4766,#4770,#916,.T.);
#6192=EDGE_CURVE('',#4772,#4773,#1665,.T.);
#6193=EDGE_CURVE('',#4774,#4772,#917,.T.);
#6194=EDGE_CURVE('',#4769,#4774,#918,.T.);
#6195=EDGE_CURVE('',#4770,#4775,#919,.T.);
#6196=EDGE_CURVE('',#4775,#4773,#920,.T.);
#6197=EDGE_CURVE('',#4776,#4777,#1666,.T.);
#6198=EDGE_CURVE('',#4778,#4776,#921,.T.);
#6199=EDGE_CURVE('',#4772,#4778,#922,.T.);
#6200=EDGE_CURVE('',#4773,#4777,#923,.T.);
#6201=EDGE_CURVE('',#4779,#4780,#1667,.T.);
#6202=EDGE_CURVE('',#4781,#4779,#924,.T.);
#6203=EDGE_CURVE('',#4776,#4781,#925,.T.);
#6204=EDGE_CURVE('',#4777,#4782,#926,.T.);
#6205=EDGE_CURVE('',#4782,#4780,#927,.T.);
#6206=EDGE_CURVE('',#4783,#4784,#1668,.T.);
#6207=EDGE_CURVE('',#4785,#4783,#928,.T.);
#6208=EDGE_CURVE('',#4779,#4785,#929,.T.);
#6209=EDGE_CURVE('',#4780,#4784,#930,.T.);
#6210=EDGE_CURVE('',#4786,#4787,#1669,.T.);
#6211=EDGE_CURVE('',#4788,#4786,#931,.T.);
#6212=EDGE_CURVE('',#4783,#4788,#932,.T.);
#6213=EDGE_CURVE('',#4784,#4789,#933,.T.);
#6214=EDGE_CURVE('',#4789,#4787,#934,.T.);
#6215=EDGE_CURVE('',#4790,#4791,#1670,.T.);
#6216=EDGE_CURVE('',#4792,#4790,#935,.T.);
#6217=EDGE_CURVE('',#4786,#4792,#936,.T.);
#6218=EDGE_CURVE('',#4787,#4791,#937,.T.);
#6219=EDGE_CURVE('',#4793,#4794,#1671,.T.);
#6220=EDGE_CURVE('',#4795,#4793,#938,.T.);
#6221=EDGE_CURVE('',#4790,#4795,#939,.T.);
#6222=EDGE_CURVE('',#4791,#4796,#940,.T.);
#6223=EDGE_CURVE('',#4796,#4794,#941,.T.);
#6224=EDGE_CURVE('',#4797,#4798,#1672,.T.);
#6225=EDGE_CURVE('',#4799,#4797,#942,.T.);
#6226=EDGE_CURVE('',#4793,#4799,#943,.T.);
#6227=EDGE_CURVE('',#4794,#4798,#944,.T.);
#6228=EDGE_CURVE('',#4800,#4801,#1673,.T.);
#6229=EDGE_CURVE('',#4802,#4800,#945,.T.);
#6230=EDGE_CURVE('',#4797,#4802,#946,.T.);
#6231=EDGE_CURVE('',#4798,#4803,#947,.T.);
#6232=EDGE_CURVE('',#4803,#4801,#948,.T.);
#6233=EDGE_CURVE('',#4804,#4805,#1674,.T.);
#6234=EDGE_CURVE('',#4806,#4804,#949,.T.);
#6235=EDGE_CURVE('',#4800,#4806,#950,.T.);
#6236=EDGE_CURVE('',#4801,#4805,#951,.T.);
#6237=EDGE_CURVE('',#4807,#4808,#1675,.T.);
#6238=EDGE_CURVE('',#4809,#4807,#952,.T.);
#6239=EDGE_CURVE('',#4804,#4809,#953,.T.);
#6240=EDGE_CURVE('',#4805,#4810,#954,.T.);
#6241=EDGE_CURVE('',#4810,#4808,#955,.T.);
#6242=EDGE_CURVE('',#4811,#4812,#956,.T.);
#6243=EDGE_CURVE('',#4812,#4813,#3826,.T.);
#6244=EDGE_CURVE('',#4813,#4814,#957,.T.);
#6245=EDGE_CURVE('',#4814,#4815,#958,.T.);
#6246=EDGE_CURVE('',#4815,#4816,#959,.T.);
#6247=EDGE_CURVE('',#4816,#4817,#960,.T.);
#6248=EDGE_CURVE('',#4817,#4818,#961,.T.);
#6249=EDGE_CURVE('',#4818,#4819,#962,.T.);
#6250=EDGE_CURVE('',#4819,#4820,#963,.T.);
#6251=EDGE_CURVE('',#4820,#4821,#964,.T.);
#6252=EDGE_CURVE('',#4821,#4822,#965,.T.);
#6253=EDGE_CURVE('',#4822,#4823,#966,.T.);
#6254=EDGE_CURVE('',#4823,#4824,#967,.T.);
#6255=EDGE_CURVE('',#4824,#4825,#968,.T.);
#6256=EDGE_CURVE('',#4825,#4826,#969,.T.);
#6257=EDGE_CURVE('',#4826,#4827,#970,.T.);
#6258=EDGE_CURVE('',#4827,#4828,#971,.T.);
#6259=EDGE_CURVE('',#4829,#4828,#3827,.T.);
#6260=EDGE_CURVE('',#4829,#4830,#972,.T.);
#6261=EDGE_CURVE('',#4830,#4831,#973,.T.);
#6262=EDGE_CURVE('',#4831,#4832,#974,.T.);
#6263=EDGE_CURVE('',#4832,#4833,#975,.T.);
#6264=EDGE_CURVE('',#4833,#4834,#976,.T.);
#6265=EDGE_CURVE('',#4834,#4835,#977,.T.);
#6266=EDGE_CURVE('',#4835,#4836,#978,.T.);
#6267=EDGE_CURVE('',#4836,#4837,#979,.T.);
#6268=EDGE_CURVE('',#4837,#4838,#980,.T.);
#6269=EDGE_CURVE('',#4838,#4839,#981,.T.);
#6270=EDGE_CURVE('',#4839,#4840,#982,.T.);
#6271=EDGE_CURVE('',#4840,#4841,#983,.T.);
#6272=EDGE_CURVE('',#4841,#4842,#984,.T.);
#6273=EDGE_CURVE('',#4842,#4811,#985,.T.);
#6274=EDGE_CURVE('',#4808,#4843,#986,.T.);
#6275=EDGE_CURVE('',#4843,#4844,#987,.T.);
#6276=EDGE_CURVE('',#4845,#4844,#3828,.T.);
#6277=EDGE_CURVE('',#4846,#4845,#988,.T.);
#6278=EDGE_CURVE('',#4807,#4846,#989,.T.);
#6279=EDGE_CURVE('',#4828,#4845,#990,.T.);
#6280=EDGE_CURVE('',#4763,#4813,#991,.T.);
#6281=EDGE_CURVE('',#4813,#4847,#3829,.T.);
#6282=EDGE_CURVE('',#4847,#4848,#3830,.T.);
#6283=EDGE_CURVE('',#4848,#4764,#992,.T.);
#6284=EDGE_CURVE('',#4844,#4829,#993,.T.);
#6285=EDGE_CURVE('',#4848,#4812,#994,.T.);
#6286=EDGE_CURVE('',#4849,#4850,#147,.T.);
#6287=EDGE_CURVE('',#4850,#4849,#3831,.T.);
#6288=EDGE_CURVE('',#4851,#4852,#148,.T.);
#6289=EDGE_CURVE('',#4852,#4851,#3832,.T.);
#6290=EDGE_CURVE('',#4853,#4854,#149,.T.);
#6291=EDGE_CURVE('',#4854,#4853,#3833,.T.);
#6292=EDGE_CURVE('',#4855,#4856,#150,.T.);
#6293=EDGE_CURVE('',#4856,#4855,#3834,.T.);
#6294=EDGE_CURVE('',#4857,#4858,#151,.T.);
#6295=EDGE_CURVE('',#4859,#4857,#3835,.T.);
#6296=EDGE_CURVE('',#4858,#4859,#3836,.T.);
#6297=EDGE_CURVE('',#4860,#4861,#152,.T.);
#6298=EDGE_CURVE('',#4861,#4860,#3837,.T.);
#6299=EDGE_CURVE('',#4859,#4862,#3838,.T.);
#6300=EDGE_CURVE('',#4862,#4862,#3839,.T.);
#6301=EDGE_CURVE('',#4857,#4863,#3840,.T.);
#6302=EDGE_CURVE('',#4863,#4856,#3841,.T.);
#6303=EDGE_CURVE('',#4855,#4864,#3842,.T.);
#6304=EDGE_CURVE('',#4864,#4854,#3843,.T.);
#6305=EDGE_CURVE('',#4853,#4865,#3844,.T.);
#6306=EDGE_CURVE('',#4865,#4850,#3845,.T.);
#6307=EDGE_CURVE('',#4849,#4866,#3846,.T.);
#6308=EDGE_CURVE('',#4866,#4852,#3847,.T.);
#6309=EDGE_CURVE('',#4851,#4867,#3848,.T.);
#6310=EDGE_CURVE('',#4867,#4861,#3849,.T.);
#6311=EDGE_CURVE('',#4860,#4868,#3850,.T.);
#6312=EDGE_CURVE('',#4868,#4858,#3851,.T.);
#6313=EDGE_CURVE('',#4869,#4870,#1676,.T.);
#6314=EDGE_CURVE('',#4870,#4870,#3852,.T.);
#6315=EDGE_CURVE('',#4867,#4871,#1677,.T.);
#6316=EDGE_CURVE('',#4871,#4872,#1678,.T.);
#6317=EDGE_CURVE('',#4868,#4872,#1679,.T.);
#6318=EDGE_CURVE('',#4872,#4873,#1680,.T.);
#6319=EDGE_CURVE('',#4863,#4873,#1681,.T.);
#6320=EDGE_CURVE('',#4873,#4874,#1682,.T.);
#6321=EDGE_CURVE('',#4864,#4874,#1683,.T.);
#6322=EDGE_CURVE('',#4874,#4875,#1684,.T.);
#6323=EDGE_CURVE('',#4865,#4875,#1685,.T.);
#6324=EDGE_CURVE('',#4866,#4876,#1686,.T.);
#6325=EDGE_CURVE('',#4876,#4871,#1687,.T.);
#6326=EDGE_CURVE('',#4875,#4876,#1688,.T.);
#6327=EDGE_CURVE('',#4877,#4877,#3853,.T.);
#6328=EDGE_CURVE('',#4847,#4877,#1689,.T.);
#6329=EDGE_CURVE('',#4878,#4878,#3854,.T.);
#6330=EDGE_CURVE('',#4862,#4878,#1690,.T.);
#8903=ORIENTED_EDGE('',*,*,#6179,.F.);
#8904=ORIENTED_EDGE('',*,*,#6180,.F.);
#8905=ORIENTED_EDGE('',*,*,#6181,.F.);
#8906=ORIENTED_EDGE('',*,*,#6182,.T.);
#8907=ORIENTED_EDGE('',*,*,#6183,.F.);
#8908=ORIENTED_EDGE('',*,*,#6184,.F.);
#8909=ORIENTED_EDGE('',*,*,#6185,.F.);
#8910=ORIENTED_EDGE('',*,*,#6179,.T.);
#8911=ORIENTED_EDGE('',*,*,#6186,.T.);
#8912=ORIENTED_EDGE('',*,*,#6187,.T.);
#8913=ORIENTED_EDGE('',*,*,#6188,.F.);
#8914=ORIENTED_EDGE('',*,*,#6189,.F.);
#8915=ORIENTED_EDGE('',*,*,#6190,.F.);
#8916=ORIENTED_EDGE('',*,*,#6183,.T.);
#8917=ORIENTED_EDGE('',*,*,#6191,.T.);
#8918=ORIENTED_EDGE('',*,*,#6192,.F.);
#8919=ORIENTED_EDGE('',*,*,#6193,.F.);
#8920=ORIENTED_EDGE('',*,*,#6194,.F.);
#8921=ORIENTED_EDGE('',*,*,#6188,.T.);
#8922=ORIENTED_EDGE('',*,*,#6195,.T.);
#8923=ORIENTED_EDGE('',*,*,#6196,.T.);
#8924=ORIENTED_EDGE('',*,*,#6197,.F.);
#8925=ORIENTED_EDGE('',*,*,#6198,.F.);
#8926=ORIENTED_EDGE('',*,*,#6199,.F.);
#8927=ORIENTED_EDGE('',*,*,#6192,.T.);
#8928=ORIENTED_EDGE('',*,*,#6200,.T.);
#8929=ORIENTED_EDGE('',*,*,#6201,.F.);
#8930=ORIENTED_EDGE('',*,*,#6202,.F.);
#8931=ORIENTED_EDGE('',*,*,#6203,.F.);
#8932=ORIENTED_EDGE('',*,*,#6197,.T.);
#8933=ORIENTED_EDGE('',*,*,#6204,.T.);
#8934=ORIENTED_EDGE('',*,*,#6205,.T.);
#8935=ORIENTED_EDGE('',*,*,#6206,.F.);
#8936=ORIENTED_EDGE('',*,*,#6207,.F.);
#8937=ORIENTED_EDGE('',*,*,#6208,.F.);
#8938=ORIENTED_EDGE('',*,*,#6201,.T.);
#8939=ORIENTED_EDGE('',*,*,#6209,.T.);
#8940=ORIENTED_EDGE('',*,*,#6210,.F.);
#8941=ORIENTED_EDGE('',*,*,#6211,.F.);
#8942=ORIENTED_EDGE('',*,*,#6212,.F.);
#8943=ORIENTED_EDGE('',*,*,#6206,.T.);
#8944=ORIENTED_EDGE('',*,*,#6213,.T.);
#8945=ORIENTED_EDGE('',*,*,#6214,.T.);
#8946=ORIENTED_EDGE('',*,*,#6215,.F.);
#8947=ORIENTED_EDGE('',*,*,#6216,.F.);
#8948=ORIENTED_EDGE('',*,*,#6217,.F.);
#8949=ORIENTED_EDGE('',*,*,#6210,.T.);
#8950=ORIENTED_EDGE('',*,*,#6218,.T.);
#8951=ORIENTED_EDGE('',*,*,#6219,.F.);
#8952=ORIENTED_EDGE('',*,*,#6220,.F.);
#8953=ORIENTED_EDGE('',*,*,#6221,.F.);
#8954=ORIENTED_EDGE('',*,*,#6215,.T.);
#8955=ORIENTED_EDGE('',*,*,#6222,.T.);
#8956=ORIENTED_EDGE('',*,*,#6223,.T.);
#8957=ORIENTED_EDGE('',*,*,#6224,.F.);
#8958=ORIENTED_EDGE('',*,*,#6225,.F.);
#8959=ORIENTED_EDGE('',*,*,#6226,.F.);
#8960=ORIENTED_EDGE('',*,*,#6219,.T.);
#8961=ORIENTED_EDGE('',*,*,#6227,.T.);
#8962=ORIENTED_EDGE('',*,*,#6228,.F.);
#8963=ORIENTED_EDGE('',*,*,#6229,.F.);
#8964=ORIENTED_EDGE('',*,*,#6230,.F.);
#8965=ORIENTED_EDGE('',*,*,#6224,.T.);
#8966=ORIENTED_EDGE('',*,*,#6231,.T.);
#8967=ORIENTED_EDGE('',*,*,#6232,.T.);
#8968=ORIENTED_EDGE('',*,*,#6233,.F.);
#8969=ORIENTED_EDGE('',*,*,#6234,.F.);
#8970=ORIENTED_EDGE('',*,*,#6235,.F.);
#8971=ORIENTED_EDGE('',*,*,#6228,.T.);
#8972=ORIENTED_EDGE('',*,*,#6236,.T.);
#8973=ORIENTED_EDGE('',*,*,#6237,.F.);
#8974=ORIENTED_EDGE('',*,*,#6238,.F.);
#8975=ORIENTED_EDGE('',*,*,#6239,.F.);
#8976=ORIENTED_EDGE('',*,*,#6233,.T.);
#8977=ORIENTED_EDGE('',*,*,#6240,.T.);
#8978=ORIENTED_EDGE('',*,*,#6241,.T.);
#8979=ORIENTED_EDGE('',*,*,#6242,.T.);
#8980=ORIENTED_EDGE('',*,*,#6243,.T.);
#8981=ORIENTED_EDGE('',*,*,#6244,.T.);
#8982=ORIENTED_EDGE('',*,*,#6245,.T.);
#8983=ORIENTED_EDGE('',*,*,#6246,.T.);
#8984=ORIENTED_EDGE('',*,*,#6247,.T.);
#8985=ORIENTED_EDGE('',*,*,#6248,.T.);
#8986=ORIENTED_EDGE('',*,*,#6249,.T.);
#8987=ORIENTED_EDGE('',*,*,#6250,.T.);
#8988=ORIENTED_EDGE('',*,*,#6251,.T.);
#8989=ORIENTED_EDGE('',*,*,#6252,.T.);
#8990=ORIENTED_EDGE('',*,*,#6253,.T.);
#8991=ORIENTED_EDGE('',*,*,#6254,.T.);
#8992=ORIENTED_EDGE('',*,*,#6255,.T.);
#8993=ORIENTED_EDGE('',*,*,#6256,.T.);
#8994=ORIENTED_EDGE('',*,*,#6257,.T.);
#8995=ORIENTED_EDGE('',*,*,#6258,.T.);
#8996=ORIENTED_EDGE('',*,*,#6259,.F.);
#8997=ORIENTED_EDGE('',*,*,#6260,.T.);
#8998=ORIENTED_EDGE('',*,*,#6261,.T.);
#8999=ORIENTED_EDGE('',*,*,#6262,.T.);
#9000=ORIENTED_EDGE('',*,*,#6263,.T.);
#9001=ORIENTED_EDGE('',*,*,#6264,.T.);
#9002=ORIENTED_EDGE('',*,*,#6265,.T.);
#9003=ORIENTED_EDGE('',*,*,#6266,.T.);
#9004=ORIENTED_EDGE('',*,*,#6267,.T.);
#9005=ORIENTED_EDGE('',*,*,#6268,.T.);
#9006=ORIENTED_EDGE('',*,*,#6269,.T.);
#9007=ORIENTED_EDGE('',*,*,#6270,.T.);
#9008=ORIENTED_EDGE('',*,*,#6271,.T.);
#9009=ORIENTED_EDGE('',*,*,#6272,.T.);
#9010=ORIENTED_EDGE('',*,*,#6273,.T.);
#9011=ORIENTED_EDGE('',*,*,#6237,.T.);
#9012=ORIENTED_EDGE('',*,*,#6274,.T.);
#9013=ORIENTED_EDGE('',*,*,#6275,.T.);
#9014=ORIENTED_EDGE('',*,*,#6276,.F.);
#9015=ORIENTED_EDGE('',*,*,#6277,.F.);
#9016=ORIENTED_EDGE('',*,*,#6278,.F.);
#9017=ORIENTED_EDGE('',*,*,#6279,.F.);
#9018=ORIENTED_EDGE('',*,*,#6258,.F.);
#9019=ORIENTED_EDGE('',*,*,#6257,.F.);
#9020=ORIENTED_EDGE('',*,*,#6256,.F.);
#9021=ORIENTED_EDGE('',*,*,#6255,.F.);
#9022=ORIENTED_EDGE('',*,*,#6254,.F.);
#9023=ORIENTED_EDGE('',*,*,#6253,.F.);
#9024=ORIENTED_EDGE('',*,*,#6252,.F.);
#9025=ORIENTED_EDGE('',*,*,#6251,.F.);
#9026=ORIENTED_EDGE('',*,*,#6250,.F.);
#9027=ORIENTED_EDGE('',*,*,#6249,.F.);
#9028=ORIENTED_EDGE('',*,*,#6248,.F.);
#9029=ORIENTED_EDGE('',*,*,#6247,.F.);
#9030=ORIENTED_EDGE('',*,*,#6246,.F.);
#9031=ORIENTED_EDGE('',*,*,#6245,.F.);
#9032=ORIENTED_EDGE('',*,*,#6244,.F.);
#9033=ORIENTED_EDGE('',*,*,#6280,.F.);
#9034=ORIENTED_EDGE('',*,*,#6180,.T.);
#9035=ORIENTED_EDGE('',*,*,#6185,.T.);
#9036=ORIENTED_EDGE('',*,*,#6184,.T.);
#9037=ORIENTED_EDGE('',*,*,#6190,.T.);
#9038=ORIENTED_EDGE('',*,*,#6189,.T.);
#9039=ORIENTED_EDGE('',*,*,#6194,.T.);
#9040=ORIENTED_EDGE('',*,*,#6193,.T.);
#9041=ORIENTED_EDGE('',*,*,#6199,.T.);
#9042=ORIENTED_EDGE('',*,*,#6198,.T.);
#9043=ORIENTED_EDGE('',*,*,#6203,.T.);
#9044=ORIENTED_EDGE('',*,*,#6202,.T.);
#9045=ORIENTED_EDGE('',*,*,#6208,.T.);
#9046=ORIENTED_EDGE('',*,*,#6207,.T.);
#9047=ORIENTED_EDGE('',*,*,#6212,.T.);
#9048=ORIENTED_EDGE('',*,*,#6211,.T.);
#9049=ORIENTED_EDGE('',*,*,#6217,.T.);
#9050=ORIENTED_EDGE('',*,*,#6216,.T.);
#9051=ORIENTED_EDGE('',*,*,#6221,.T.);
#9052=ORIENTED_EDGE('',*,*,#6220,.T.);
#9053=ORIENTED_EDGE('',*,*,#6226,.T.);
#9054=ORIENTED_EDGE('',*,*,#6225,.T.);
#9055=ORIENTED_EDGE('',*,*,#6230,.T.);
#9056=ORIENTED_EDGE('',*,*,#6229,.T.);
#9057=ORIENTED_EDGE('',*,*,#6235,.T.);
#9058=ORIENTED_EDGE('',*,*,#6234,.T.);
#9059=ORIENTED_EDGE('',*,*,#6239,.T.);
#9060=ORIENTED_EDGE('',*,*,#6238,.T.);
#9061=ORIENTED_EDGE('',*,*,#6278,.T.);
#9062=ORIENTED_EDGE('',*,*,#6277,.T.);
#9063=ORIENTED_EDGE('',*,*,#6281,.T.);
#9064=ORIENTED_EDGE('',*,*,#6282,.T.);
#9065=ORIENTED_EDGE('',*,*,#6283,.T.);
#9066=ORIENTED_EDGE('',*,*,#6181,.T.);
#9067=ORIENTED_EDGE('',*,*,#6280,.T.);
#9068=ORIENTED_EDGE('',*,*,#6284,.F.);
#9069=ORIENTED_EDGE('',*,*,#6275,.F.);
#9070=ORIENTED_EDGE('',*,*,#6274,.F.);
#9071=ORIENTED_EDGE('',*,*,#6241,.F.);
#9072=ORIENTED_EDGE('',*,*,#6240,.F.);
#9073=ORIENTED_EDGE('',*,*,#6236,.F.);
#9074=ORIENTED_EDGE('',*,*,#6232,.F.);
#9075=ORIENTED_EDGE('',*,*,#6231,.F.);
#9076=ORIENTED_EDGE('',*,*,#6227,.F.);
#9077=ORIENTED_EDGE('',*,*,#6223,.F.);
#9078=ORIENTED_EDGE('',*,*,#6222,.F.);
#9079=ORIENTED_EDGE('',*,*,#6218,.F.);
#9080=ORIENTED_EDGE('',*,*,#6214,.F.);
#9081=ORIENTED_EDGE('',*,*,#6213,.F.);
#9082=ORIENTED_EDGE('',*,*,#6209,.F.);
#9083=ORIENTED_EDGE('',*,*,#6205,.F.);
#9084=ORIENTED_EDGE('',*,*,#6204,.F.);
#9085=ORIENTED_EDGE('',*,*,#6200,.F.);
#9086=ORIENTED_EDGE('',*,*,#6196,.F.);
#9087=ORIENTED_EDGE('',*,*,#6195,.F.);
#9088=ORIENTED_EDGE('',*,*,#6191,.F.);
#9089=ORIENTED_EDGE('',*,*,#6187,.F.);
#9090=ORIENTED_EDGE('',*,*,#6186,.F.);
#9091=ORIENTED_EDGE('',*,*,#6182,.F.);
#9092=ORIENTED_EDGE('',*,*,#6283,.F.);
#9093=ORIENTED_EDGE('',*,*,#6285,.T.);
#9094=ORIENTED_EDGE('',*,*,#6242,.F.);
#9095=ORIENTED_EDGE('',*,*,#6273,.F.);
#9096=ORIENTED_EDGE('',*,*,#6272,.F.);
#9097=ORIENTED_EDGE('',*,*,#6271,.F.);
#9098=ORIENTED_EDGE('',*,*,#6270,.F.);
#9099=ORIENTED_EDGE('',*,*,#6269,.F.);
#9100=ORIENTED_EDGE('',*,*,#6268,.F.);
#9101=ORIENTED_EDGE('',*,*,#6267,.F.);
#9102=ORIENTED_EDGE('',*,*,#6266,.F.);
#9103=ORIENTED_EDGE('',*,*,#6265,.F.);
#9104=ORIENTED_EDGE('',*,*,#6264,.F.);
#9105=ORIENTED_EDGE('',*,*,#6263,.F.);
#9106=ORIENTED_EDGE('',*,*,#6262,.F.);
#9107=ORIENTED_EDGE('',*,*,#6261,.F.);
#9108=ORIENTED_EDGE('',*,*,#6260,.F.);
#9109=ORIENTED_EDGE('',*,*,#6286,.F.);
#9110=ORIENTED_EDGE('',*,*,#6287,.F.);
#9111=ORIENTED_EDGE('',*,*,#6288,.F.);
#9112=ORIENTED_EDGE('',*,*,#6289,.F.);
#9113=ORIENTED_EDGE('',*,*,#6290,.F.);
#9114=ORIENTED_EDGE('',*,*,#6291,.F.);
#9115=ORIENTED_EDGE('',*,*,#6292,.F.);
#9116=ORIENTED_EDGE('',*,*,#6293,.F.);
#9117=ORIENTED_EDGE('',*,*,#6294,.F.);
#9118=ORIENTED_EDGE('',*,*,#6295,.F.);
#9119=ORIENTED_EDGE('',*,*,#6296,.F.);
#9120=ORIENTED_EDGE('',*,*,#6297,.F.);
#9121=ORIENTED_EDGE('',*,*,#6298,.F.);
#9122=ORIENTED_EDGE('',*,*,#6296,.T.);
#9123=ORIENTED_EDGE('',*,*,#6299,.T.);
#9124=ORIENTED_EDGE('',*,*,#6300,.T.);
#9125=ORIENTED_EDGE('',*,*,#6299,.F.);
#9126=ORIENTED_EDGE('',*,*,#6295,.T.);
#9127=ORIENTED_EDGE('',*,*,#6301,.T.);
#9128=ORIENTED_EDGE('',*,*,#6302,.T.);
#9129=ORIENTED_EDGE('',*,*,#6293,.T.);
#9130=ORIENTED_EDGE('',*,*,#6303,.T.);
#9131=ORIENTED_EDGE('',*,*,#6304,.T.);
#9132=ORIENTED_EDGE('',*,*,#6291,.T.);
#9133=ORIENTED_EDGE('',*,*,#6305,.T.);
#9134=ORIENTED_EDGE('',*,*,#6306,.T.);
#9135=ORIENTED_EDGE('',*,*,#6287,.T.);
#9136=ORIENTED_EDGE('',*,*,#6307,.T.);
#9137=ORIENTED_EDGE('',*,*,#6308,.T.);
#9138=ORIENTED_EDGE('',*,*,#6289,.T.);
#9139=ORIENTED_EDGE('',*,*,#6309,.T.);
#9140=ORIENTED_EDGE('',*,*,#6310,.T.);
#9141=ORIENTED_EDGE('',*,*,#6298,.T.);
#9142=ORIENTED_EDGE('',*,*,#6311,.T.);
#9143=ORIENTED_EDGE('',*,*,#6312,.T.);
#9144=ORIENTED_EDGE('',*,*,#6313,.T.);
#9145=ORIENTED_EDGE('',*,*,#6314,.F.);
#9146=ORIENTED_EDGE('',*,*,#6313,.F.);
#9147=ORIENTED_EDGE('',*,*,#6297,.T.);
#9148=ORIENTED_EDGE('',*,*,#6310,.F.);
#9149=ORIENTED_EDGE('',*,*,#6315,.T.);
#9150=ORIENTED_EDGE('',*,*,#6316,.T.);
#9151=ORIENTED_EDGE('',*,*,#6317,.F.);
#9152=ORIENTED_EDGE('',*,*,#6311,.F.);
#9153=ORIENTED_EDGE('',*,*,#6294,.T.);
#9154=ORIENTED_EDGE('',*,*,#6312,.F.);
#9155=ORIENTED_EDGE('',*,*,#6317,.T.);
#9156=ORIENTED_EDGE('',*,*,#6318,.T.);
#9157=ORIENTED_EDGE('',*,*,#6319,.F.);
#9158=ORIENTED_EDGE('',*,*,#6301,.F.);
#9159=ORIENTED_EDGE('',*,*,#6292,.T.);
#9160=ORIENTED_EDGE('',*,*,#6302,.F.);
#9161=ORIENTED_EDGE('',*,*,#6319,.T.);
#9162=ORIENTED_EDGE('',*,*,#6320,.T.);
#9163=ORIENTED_EDGE('',*,*,#6321,.F.);
#9164=ORIENTED_EDGE('',*,*,#6303,.F.);
#9165=ORIENTED_EDGE('',*,*,#6290,.T.);
#9166=ORIENTED_EDGE('',*,*,#6304,.F.);
#9167=ORIENTED_EDGE('',*,*,#6321,.T.);
#9168=ORIENTED_EDGE('',*,*,#6322,.T.);
#9169=ORIENTED_EDGE('',*,*,#6323,.F.);
#9170=ORIENTED_EDGE('',*,*,#6305,.F.);
#9171=ORIENTED_EDGE('',*,*,#6288,.T.);
#9172=ORIENTED_EDGE('',*,*,#6308,.F.);
#9173=ORIENTED_EDGE('',*,*,#6324,.T.);
#9174=ORIENTED_EDGE('',*,*,#6325,.T.);
#9175=ORIENTED_EDGE('',*,*,#6315,.F.);
#9176=ORIENTED_EDGE('',*,*,#6309,.F.);
#9177=ORIENTED_EDGE('',*,*,#6286,.T.);
#9178=ORIENTED_EDGE('',*,*,#6306,.F.);
#9179=ORIENTED_EDGE('',*,*,#6323,.T.);
#9180=ORIENTED_EDGE('',*,*,#6326,.T.);
#9181=ORIENTED_EDGE('',*,*,#6324,.F.);
#9182=ORIENTED_EDGE('',*,*,#6307,.F.);
#9183=ORIENTED_EDGE('',*,*,#6326,.F.);
#9184=ORIENTED_EDGE('',*,*,#6322,.F.);
#9185=ORIENTED_EDGE('',*,*,#6320,.F.);
#9186=ORIENTED_EDGE('',*,*,#6318,.F.);
#9187=ORIENTED_EDGE('',*,*,#6316,.F.);
#9188=ORIENTED_EDGE('',*,*,#6325,.F.);
#9189=ORIENTED_EDGE('',*,*,#6314,.T.);
#9190=ORIENTED_EDGE('',*,*,#6327,.F.);
#9191=ORIENTED_EDGE('',*,*,#6285,.F.);
#9192=ORIENTED_EDGE('',*,*,#6282,.F.);
#9193=ORIENTED_EDGE('',*,*,#6328,.T.);
#9194=ORIENTED_EDGE('',*,*,#6327,.T.);
#9195=ORIENTED_EDGE('',*,*,#6328,.F.);
#9196=ORIENTED_EDGE('',*,*,#6281,.F.);
#9197=ORIENTED_EDGE('',*,*,#6243,.F.);
#9198=ORIENTED_EDGE('',*,*,#6329,.F.);
#9199=ORIENTED_EDGE('',*,*,#6259,.T.);
#9200=ORIENTED_EDGE('',*,*,#6279,.T.);
#9201=ORIENTED_EDGE('',*,*,#6276,.T.);
#9202=ORIENTED_EDGE('',*,*,#6284,.T.);
#9203=ORIENTED_EDGE('',*,*,#6300,.F.);
#9204=ORIENTED_EDGE('',*,*,#6330,.T.);
#9205=ORIENTED_EDGE('',*,*,#6329,.T.);
#9206=ORIENTED_EDGE('',*,*,#6330,.F.);
#9811=ADVANCED_FACE('',(#2833),#2365,.T.);
#9812=ADVANCED_FACE('',(#2834),#2366,.T.);
#9813=ADVANCED_FACE('',(#2835),#2367,.T.);
#9814=ADVANCED_FACE('',(#2836),#2368,.T.);
#9815=ADVANCED_FACE('',(#2837),#2369,.T.);
#9816=ADVANCED_FACE('',(#2838),#2370,.T.);
#9817=ADVANCED_FACE('',(#2839),#2371,.T.);
#9818=ADVANCED_FACE('',(#2840),#2372,.T.);
#9819=ADVANCED_FACE('',(#2841),#2373,.T.);
#9820=ADVANCED_FACE('',(#2842),#2374,.T.);
#9821=ADVANCED_FACE('',(#2843),#2375,.T.);
#9822=ADVANCED_FACE('',(#2844),#2376,.T.);
#9823=ADVANCED_FACE('',(#2845),#2377,.T.);
#9824=ADVANCED_FACE('',(#2846),#2378,.T.);
#9825=ADVANCED_FACE('',(#2847),#2379,.T.);
#9826=ADVANCED_FACE('',(#2848),#2380,.T.);
#9827=ADVANCED_FACE('',(#2849),#384,.F.);
#9828=ADVANCED_FACE('',(#2850),#1177,.T.);
#9829=ADVANCED_FACE('',(#2851),#385,.F.);
#9830=ADVANCED_FACE('',(#2852),#190,.F.);
#9831=ADVANCED_FACE('',(#2853),#191,.F.);
#9832=ADVANCED_FACE('',(#2854),#192,.F.);
#9833=ADVANCED_FACE('',(#2855),#193,.F.);
#9834=ADVANCED_FACE('',(#2856),#194,.F.);
#9835=ADVANCED_FACE('',(#2857),#195,.F.);
#9836=ADVANCED_FACE('',(#2858),#279,.T.);
#9837=ADVANCED_FACE('',(#2859),#196,.F.);
#9838=ADVANCED_FACE('',(#2860),#1178,.F.);
#9839=ADVANCED_FACE('',(#2861),#1179,.F.);
#9840=ADVANCED_FACE('',(#2862),#1180,.F.);
#9841=ADVANCED_FACE('',(#2863),#1181,.F.);
#9842=ADVANCED_FACE('',(#2864),#1182,.F.);
#9843=ADVANCED_FACE('',(#2865),#1183,.F.);
#9844=ADVANCED_FACE('',(#2866,#473),#1184,.F.);
#9845=ADVANCED_FACE('',(#2867),#1185,.T.);
#9846=ADVANCED_FACE('',(#2868),#197,.T.);
#9847=ADVANCED_FACE('',(#2869,#474),#1186,.T.);
#9848=ADVANCED_FACE('',(#2870),#2381,.T.);
#9896=CLOSED_SHELL('',(#9811,#9812,#9813,#9814,#9815,#9816,#9817,#9818,
#9819,#9820,#9821,#9822,#9823,#9824,#9825,#9826,#9827,#9828,#9829,#9830,
#9831,#9832,#9833,#9834,#9835,#9836,#9837,#9838,#9839,#9840,#9841,#9842,
#9843,#9844,#9845,#9846,#9847,#9848));
#10788=AXIS2_PLACEMENT_3D('',#77890,#12802,#12803);
#10789=AXIS2_PLACEMENT_3D('',#77891,#12804,#12805);
#10790=AXIS2_PLACEMENT_3D('',#77946,#12807,#12808);
#10791=AXIS2_PLACEMENT_3D('',#77975,#12809,#12810);
#10792=AXIS2_PLACEMENT_3D('',#78243,#12812,#12813);
#10793=AXIS2_PLACEMENT_3D('',#78536,#12815,#12816);
#10794=AXIS2_PLACEMENT_3D('',#78858,#12818,#12819);
#10795=AXIS2_PLACEMENT_3D('',#79155,#12821,#12822);
#10796=AXIS2_PLACEMENT_3D('',#79478,#12824,#12825);
#10797=AXIS2_PLACEMENT_3D('',#79783,#12827,#12828);
#10798=AXIS2_PLACEMENT_3D('',#80090,#12830,#12831);
#10799=AXIS2_PLACEMENT_3D('',#80391,#12833,#12834);
#10800=AXIS2_PLACEMENT_3D('',#80718,#12836,#12837);
#10801=AXIS2_PLACEMENT_3D('',#81013,#12839,#12840);
#10802=AXIS2_PLACEMENT_3D('',#81329,#12842,#12843);
#10803=AXIS2_PLACEMENT_3D('',#81631,#12845,#12846);
#10804=AXIS2_PLACEMENT_3D('',#81860,#12848,#12849);
#10805=AXIS2_PLACEMENT_3D('',#81870,#12850,#12851);
#10806=AXIS2_PLACEMENT_3D('',#82973,#12852,#12853);
#10807=AXIS2_PLACEMENT_3D('',#84375,#12854,#12855);
#10808=AXIS2_PLACEMENT_3D('',#84414,#12856,#12857);
#10809=AXIS2_PLACEMENT_3D('',#84952,#12858,#12859);
#10810=AXIS2_PLACEMENT_3D('',#84954,#12860,#12861);
#10811=AXIS2_PLACEMENT_3D('',#84956,#12862,#12863);
#10812=AXIS2_PLACEMENT_3D('',#85440,#12864,#12865);
#10813=AXIS2_PLACEMENT_3D('',#85446,#12866,#12867);
#10814=AXIS2_PLACEMENT_3D('',#85447,#12868,#12869);
#10815=AXIS2_PLACEMENT_3D('',#85453,#12870,#12871);
#10816=AXIS2_PLACEMENT_3D('',#85454,#12872,#12873);
#10817=AXIS2_PLACEMENT_3D('',#85460,#12874,#12875);
#10818=AXIS2_PLACEMENT_3D('',#85461,#12876,#12877);
#10819=AXIS2_PLACEMENT_3D('',#85467,#12878,#12879);
#10820=AXIS2_PLACEMENT_3D('',#85468,#12880,#12881);
#10821=AXIS2_PLACEMENT_3D('',#85475,#12882,#12883);
#10822=AXIS2_PLACEMENT_3D('',#85476,#12884,#12885);
#10823=AXIS2_PLACEMENT_3D('',#85477,#12886,#12887);
#10824=AXIS2_PLACEMENT_3D('',#85483,#12888,#12889);
#10825=AXIS2_PLACEMENT_3D('',#85484,#12890,#12891);
#10826=AXIS2_PLACEMENT_3D('',#85486,#12892,#12893);
#10827=AXIS2_PLACEMENT_3D('',#85487,#12894,#12895);
#10828=AXIS2_PLACEMENT_3D('',#85489,#12896,#12897);
#10829=AXIS2_PLACEMENT_3D('',#85490,#12898,#12899);
#10830=AXIS2_PLACEMENT_3D('',#85492,#12900,#12901);
#10831=AXIS2_PLACEMENT_3D('',#85493,#12902,#12903);
#10832=AXIS2_PLACEMENT_3D('',#85495,#12904,#12905);
#10833=AXIS2_PLACEMENT_3D('',#85496,#12906,#12907);
#10834=AXIS2_PLACEMENT_3D('',#85498,#12908,#12909);
#10835=AXIS2_PLACEMENT_3D('',#85499,#12910,#12911);
#10836=AXIS2_PLACEMENT_3D('',#85501,#12912,#12913);
#10837=AXIS2_PLACEMENT_3D('',#85502,#12914,#12915);
#10838=AXIS2_PLACEMENT_3D('',#85504,#12916,#12917);
#10839=AXIS2_PLACEMENT_3D('',#85505,#12918,#12919);
#10840=AXIS2_PLACEMENT_3D('',#85506,#12920,#12921);
#10841=AXIS2_PLACEMENT_3D('',#85510,#12923,#12924);
#10842=AXIS2_PLACEMENT_3D('',#85511,#12925,#12926);
#10843=AXIS2_PLACEMENT_3D('',#85517,#12930,#12931);
#10844=AXIS2_PLACEMENT_3D('',#85521,#12934,#12935);
#10845=AXIS2_PLACEMENT_3D('',#85525,#12938,#12939);
#10846=AXIS2_PLACEMENT_3D('',#85529,#12942,#12943);
#10847=AXIS2_PLACEMENT_3D('',#85533,#12946,#12947);
#10848=AXIS2_PLACEMENT_3D('',#85535,#12949,#12950);
#10849=AXIS2_PLACEMENT_3D('',#85536,#12951,#12952);
#10850=AXIS2_PLACEMENT_3D('',#85538,#12953,#12954);
#10851=AXIS2_PLACEMENT_3D('',#85539,#12955,#12956);
#10852=AXIS2_PLACEMENT_3D('',#85541,#12958,#12959);
#10853=AXIS2_PLACEMENT_3D('',#85543,#12960,#12961);
#10854=AXIS2_PLACEMENT_3D('',#85544,#12962,#12963);
#12802=DIRECTION('axis',(0.,0.,1.));
#12803=DIRECTION('refdir',(1.,0.,0.));
#12804=DIRECTION('center_axis',(0.,0.,1.));
#12805=DIRECTION('ref_axis',(-0.6579379160252,-0.753072173603843,0.));
#12806=DIRECTION('',(0.,0.,-1.));
#12807=DIRECTION('center_axis',(0.,0.,-1.));
#12808=DIRECTION('ref_axis',(1.,8.51023079448757E-14,0.));
#12809=DIRECTION('center_axis',(0.,0.,1.));
#12810=DIRECTION('ref_axis',(-0.6579379160252,-0.753072173603843,0.));
#12811=DIRECTION('',(0.,0.,-1.));
#12812=DIRECTION('center_axis',(0.,0.,1.));
#12813=DIRECTION('ref_axis',(-0.6579379160252,-0.753072173603843,0.));
#12814=DIRECTION('',(0.,0.,-1.));
#12815=DIRECTION('center_axis',(0.,0.,1.));
#12816=DIRECTION('ref_axis',(-0.6579379160252,-0.753072173603843,0.));
#12817=DIRECTION('',(0.,0.,-1.));
#12818=DIRECTION('center_axis',(0.,0.,1.));
#12819=DIRECTION('ref_axis',(-0.6579379160252,-0.753072173603843,0.));
#12820=DIRECTION('',(0.,0.,-1.));
#12821=DIRECTION('center_axis',(0.,0.,1.));
#12822=DIRECTION('ref_axis',(-0.6579379160252,-0.753072173603843,0.));
#12823=DIRECTION('',(0.,0.,-1.));
#12824=DIRECTION('center_axis',(0.,0.,1.));
#12825=DIRECTION('ref_axis',(-0.6579379160252,-0.753072173603843,0.));
#12826=DIRECTION('',(0.,0.,-1.));
#12827=DIRECTION('center_axis',(0.,0.,1.));
#12828=DIRECTION('ref_axis',(-0.6579379160252,-0.753072173603843,0.));
#12829=DIRECTION('',(0.,0.,-1.));
#12830=DIRECTION('center_axis',(0.,0.,1.));
#12831=DIRECTION('ref_axis',(-0.6579379160252,-0.753072173603843,0.));
#12832=DIRECTION('',(0.,0.,-1.));
#12833=DIRECTION('center_axis',(0.,0.,1.));
#12834=DIRECTION('ref_axis',(-0.6579379160252,-0.753072173603843,0.));
#12835=DIRECTION('',(0.,0.,-1.));
#12836=DIRECTION('center_axis',(0.,0.,1.));
#12837=DIRECTION('ref_axis',(-0.6579379160252,-0.753072173603843,0.));
#12838=DIRECTION('',(0.,0.,-1.));
#12839=DIRECTION('center_axis',(0.,0.,1.));
#12840=DIRECTION('ref_axis',(-0.6579379160252,-0.753072173603843,0.));
#12841=DIRECTION('',(0.,0.,-1.));
#12842=DIRECTION('center_axis',(0.,0.,1.));
#12843=DIRECTION('ref_axis',(-0.6579379160252,-0.753072173603843,0.));
#12844=DIRECTION('',(0.,0.,-1.));
#12845=DIRECTION('center_axis',(0.,0.,1.));
#12846=DIRECTION('ref_axis',(-0.6579379160252,-0.753072173603843,0.));
#12847=DIRECTION('',(0.,0.,-1.));
#12848=DIRECTION('center_axis',(0.,0.,1.));
#12849=DIRECTION('ref_axis',(1.,0.,0.));
#12850=DIRECTION('center_axis',(0.,0.,1.));
#12851=DIRECTION('ref_axis',(1.,0.,0.));
#12852=DIRECTION('center_axis',(0.,0.,1.));
#12853=DIRECTION('ref_axis',(1.,0.,0.));
#12854=DIRECTION('center_axis',(0.,0.,1.));
#12855=DIRECTION('ref_axis',(-0.6579379160252,-0.753072173603843,0.));
#12856=DIRECTION('center_axis',(0.,0.,1.));
#12857=DIRECTION('ref_axis',(1.,8.51023079448757E-14,0.));
#12858=DIRECTION('center_axis',(0.,0.,1.));
#12859=DIRECTION('ref_axis',(1.,0.,0.));
#12860=DIRECTION('center_axis',(0.,0.,1.));
#12861=DIRECTION('ref_axis',(1.,0.,0.));
#12862=DIRECTION('center_axis',(0.,0.,1.));
#12863=DIRECTION('ref_axis',(1.,0.,0.));
#12864=DIRECTION('center_axis',(0.,0.,1.));
#12865=DIRECTION('ref_axis',(1.,0.,0.));
#12866=DIRECTION('center_axis',(0.,0.,-1.));
#12867=DIRECTION('ref_axis',(1.,0.,0.));
#12868=DIRECTION('center_axis',(0.,0.,1.));
#12869=DIRECTION('ref_axis',(1.,0.,0.));
#12870=DIRECTION('center_axis',(0.,0.,-1.));
#12871=DIRECTION('ref_axis',(1.,0.,0.));
#12872=DIRECTION('center_axis',(0.,0.,1.));
#12873=DIRECTION('ref_axis',(1.,0.,0.));
#12874=DIRECTION('center_axis',(0.,0.,-1.));
#12875=DIRECTION('ref_axis',(1.,0.,0.));
#12876=DIRECTION('center_axis',(0.,0.,1.));
#12877=DIRECTION('ref_axis',(1.,0.,0.));
#12878=DIRECTION('center_axis',(0.,0.,-1.));
#12879=DIRECTION('ref_axis',(1.,0.,0.));
#12880=DIRECTION('center_axis',(0.,0.,1.));
#12881=DIRECTION('ref_axis',(-1.,-1.22464679914735E-16,0.));
#12882=DIRECTION('center_axis',(0.,0.,-1.));
#12883=DIRECTION('ref_axis',(1.,0.,0.));
#12884=DIRECTION('center_axis',(0.,0.,-1.));
#12885=DIRECTION('ref_axis',(1.,0.,0.));
#12886=DIRECTION('center_axis',(0.,0.,1.));
#12887=DIRECTION('ref_axis',(1.,0.,0.));
#12888=DIRECTION('center_axis',(0.,0.,-1.));
#12889=DIRECTION('ref_axis',(1.,0.,0.));
#12890=DIRECTION('center_axis',(1.22464679914735E-16,0.,1.));
#12891=DIRECTION('ref_axis',(1.,0.,-1.1686558153949E-16));
#12892=DIRECTION('center_axis',(1.22464679914735E-16,-1.,-7.49879891330929E-33));
#12893=DIRECTION('ref_axis',(-1.,-1.22464679914735E-16,1.1686558153949E-16));
#12894=DIRECTION('center_axis',(0.,0.,1.));
#12895=DIRECTION('ref_axis',(1.,0.,0.));
#12896=DIRECTION('center_axis',(-1.,-1.92296268638356E-16,0.));
#12897=DIRECTION('ref_axis',(0.,0.,-1.));
#12898=DIRECTION('center_axis',(-0.5,0.866025403784439,0.));
#12899=DIRECTION('ref_axis',(0.,0.,-1.));
#12900=DIRECTION('center_axis',(-0.5,0.866025403784439,0.));
#12901=DIRECTION('ref_axis',(0.,0.,-1.));
#12902=DIRECTION('center_axis',(0.5,0.866025403784439,0.));
#12903=DIRECTION('ref_axis',(0.,0.,-1.));
#12904=DIRECTION('center_axis',(0.5,0.866025403784439,0.));
#12905=DIRECTION('ref_axis',(0.,0.,-1.));
#12906=DIRECTION('center_axis',(1.,-3.84592537276713E-16,0.));
#12907=DIRECTION('ref_axis',(0.,0.,1.));
#12908=DIRECTION('center_axis',(1.,-3.84592537276713E-16,0.));
#12909=DIRECTION('ref_axis',(0.,0.,1.));
#12910=DIRECTION('center_axis',(0.5,-0.866025403784439,0.));
#12911=DIRECTION('ref_axis',(0.,0.,1.));
#12912=DIRECTION('center_axis',(0.5,-0.866025403784439,0.));
#12913=DIRECTION('ref_axis',(0.,0.,1.));
#12914=DIRECTION('center_axis',(-0.5,-0.866025403784439,0.));
#12915=DIRECTION('ref_axis',(0.,0.,1.));
#12916=DIRECTION('center_axis',(-0.5,-0.866025403784439,0.));
#12917=DIRECTION('ref_axis',(0.,0.,1.));
#12918=DIRECTION('center_axis',(-1.,-1.92296268638356E-16,0.));
#12919=DIRECTION('ref_axis',(0.,0.,-1.));
#12920=DIRECTION('center_axis',(0.,0.,1.));
#12921=DIRECTION('ref_axis',(1.,0.,0.));
#12922=DIRECTION('',(-0.854074023911687,-1.04593901961835E-16,0.520151479551197));
#12923=DIRECTION('center_axis',(0.,0.,-1.));
#12924=DIRECTION('ref_axis',(1.,0.,0.));
#12925=DIRECTION('center_axis',(-0.5,-0.866025403784439,0.));
#12926=DIRECTION('ref_axis',(-0.866025403784439,0.5,0.));
#12927=DIRECTION('',(0.,0.,-1.));
#12928=DIRECTION('',(-0.866025403784439,0.5,0.));
#12929=DIRECTION('',(0.,0.,-1.));
#12930=DIRECTION('center_axis',(-1.,-1.92296268638356E-16,0.));
#12931=DIRECTION('ref_axis',(-1.92296268638356E-16,1.,0.));
#12932=DIRECTION('',(-1.92296268638356E-16,1.,0.));
#12933=DIRECTION('',(0.,0.,-1.));
#12934=DIRECTION('center_axis',(-0.5,0.866025403784439,0.));
#12935=DIRECTION('ref_axis',(0.866025403784439,0.5,0.));
#12936=DIRECTION('',(0.866025403784439,0.5,0.));
#12937=DIRECTION('',(0.,0.,-1.));
#12938=DIRECTION('center_axis',(0.5,0.866025403784439,0.));
#12939=DIRECTION('ref_axis',(0.866025403784439,-0.5,0.));
#12940=DIRECTION('',(0.866025403784439,-0.5,0.));
#12941=DIRECTION('',(0.,0.,-1.));
#12942=DIRECTION('center_axis',(0.5,-0.866025403784439,0.));
#12943=DIRECTION('ref_axis',(-0.866025403784439,-0.5,0.));
#12944=DIRECTION('',(0.,0.,-1.));
#12945=DIRECTION('',(-0.866025403784439,-0.5,0.));
#12946=DIRECTION('center_axis',(1.,-3.84592537276713E-16,0.));
#12947=DIRECTION('ref_axis',(-3.84592537276713E-16,-1.,0.));
#12948=DIRECTION('',(-3.84592537276713E-16,-1.,0.));
#12949=DIRECTION('center_axis',(0.,0.,-1.));
#12950=DIRECTION('ref_axis',(-1.,0.,0.));
#12951=DIRECTION('center_axis',(0.,0.,-1.));
#12952=DIRECTION('ref_axis',(-1.,0.,0.));
#12953=DIRECTION('center_axis',(0.,0.,1.));
#12954=DIRECTION('ref_axis',(1.,0.,0.));
#12955=DIRECTION('center_axis',(0.,0.,1.));
#12956=DIRECTION('ref_axis',(1.,0.,0.));
#12957=DIRECTION('',(0.707106781186547,8.65956056235493E-17,-0.707106781186548));
#12958=DIRECTION('center_axis',(0.,0.,-1.));
#12959=DIRECTION('ref_axis',(-1.,0.,0.));
#12960=DIRECTION('center_axis',(0.,0.,1.));
#12961=DIRECTION('ref_axis',(1.,0.,0.));
#12962=DIRECTION('center_axis',(0.,0.,1.));
#12963=DIRECTION('ref_axis',(1.,0.,0.));
#12964=DIRECTION('',(0.,0.,-1.));
#77890=CARTESIAN_POINT('',(0.,0.,0.));
#77891=CARTESIAN_POINT('Origin',(0.,0.,-1.10400562256037));
#77892=CARTESIAN_POINT('',(0.10234224283772,0.117140376604078,-0.940688754930896));
#77893=CARTESIAN_POINT('',(0.10234224283772,0.117140376604078,-0.954511891220802));
#77894=CARTESIAN_POINT('',(0.10234224283772,0.117140376604078,-1.10400562256037));
#77895=CARTESIAN_POINT('',(-0.0903576739864822,-0.126614743421738,-0.974595553498516));
#77896=CARTESIAN_POINT('Ctrl Pts',(-0.0903576739864822,-0.126614743421738,
-0.974595553498516));
#77897=CARTESIAN_POINT('Ctrl Pts',(-0.0821020793447133,-0.132506287400316,
-0.973865238560292));
#77898=CARTESIAN_POINT('Ctrl Pts',(-0.0732355876927443,-0.137609834113344,
-0.973134923622068));
#77899=CARTESIAN_POINT('Ctrl Pts',(-0.0639336210870726,-0.141803718550307,
-0.972404608683844));
#77900=CARTESIAN_POINT('Ctrl Pts',(-0.0546429158501588,-0.145992525686826,
-0.971675177896917));
#77901=CARTESIAN_POINT('Ctrl Pts',(-0.0449185996211577,-0.149273384832242,
-0.970945747109989));
#77902=CARTESIAN_POINT('Ctrl Pts',(-0.0349613681409583,-0.151570133066222,
-0.970216316323061));
#77903=CARTESIAN_POINT('Ctrl Pts',(-0.0250122354972982,-0.153865013211813,
-0.969487478827624));
#77904=CARTESIAN_POINT('Ctrl Pts',(-0.0148314833881561,-0.155177149067038,
-0.968758641332187));
#77905=CARTESIAN_POINT('Ctrl Pts',(-0.00463218640829535,-0.155481012824971,
-0.968029803836751));
#77906=CARTESIAN_POINT('Ctrl Pts',(0.00559025742364215,-0.155785566188224,
-0.967299312276947));
#77907=CARTESIAN_POINT('Ctrl Pts',(0.0158303791967561,-0.155077282770819,
-0.966568820717144));
#77908=CARTESIAN_POINT('Ctrl Pts',(0.0258748256235762,-0.153382840953444,
-0.965838329157341));
#77909=CARTESIAN_POINT('Ctrl Pts',(0.0326789164752719,-0.152235028960784,
-0.96534349542255));
#77910=CARTESIAN_POINT('Ctrl Pts',(0.039393259145739,-0.150635817813979,
-0.964848661687758));
#77911=CARTESIAN_POINT('Ctrl Pts',(0.045955143606566,-0.148606619220343,
-0.964353827952967));
#77912=CARTESIAN_POINT('Ctrl Pts',(0.0557528548327958,-0.145576772846209,
-0.963614979521936));
#77913=CARTESIAN_POINT('Ctrl Pts',(0.0652846037394777,-0.141563026261673,
-0.962876131090906));
#77914=CARTESIAN_POINT('Ctrl Pts',(0.0743438561876921,-0.13663379357664,
-0.962137282659876));
#77915=CARTESIAN_POINT('Ctrl Pts',(0.0834049481319706,-0.131703560002827,
-0.96139828420446));
#77916=CARTESIAN_POINT('Ctrl Pts',(0.091992485818785,-0.125857799939113,
-0.960659285749044));
#77917=CARTESIAN_POINT('Ctrl Pts',(0.099920187723521,-0.119213080596453,
-0.959920287293628));
#77918=CARTESIAN_POINT('Ctrl Pts',(0.107829175180873,-0.112584047041681,
-0.959183033347261));
#77919=CARTESIAN_POINT('Ctrl Pts',(0.11508071757252,-0.105160402097257,
-0.958445779400894));
#77920=CARTESIAN_POINT('Ctrl Pts',(0.121522063240699,-0.0970988704657448,
-0.957708525454528));
#77921=CARTESIAN_POINT('Ctrl Pts',(0.12798627142293,-0.0890087257322975,
-0.956968654744587));
#77922=CARTESIAN_POINT('Ctrl Pts',(0.13363394877096,-0.0802768955027428,
-0.956228784034647));
#77923=CARTESIAN_POINT('Ctrl Pts',(0.138353019634039,-0.0710932096486248,
-0.955488913324707));
#77924=CARTESIAN_POINT('Ctrl Pts',(0.143072090497117,-0.0619095237945068,
-0.954749042614766));
#77925=CARTESIAN_POINT('Ctrl Pts',(0.146862245092671,-0.0522748617005637,
-0.954009171904826));
#77926=CARTESIAN_POINT('Ctrl Pts',(0.149660270154457,-0.0423981843631897,
-0.953269301194886));
#77927=CARTESIAN_POINT('Ctrl Pts',(0.152445749361897,-0.0325657923172453,
-0.952532747935632));
#77928=CARTESIAN_POINT('Ctrl Pts',(0.154268738348244,-0.0224202029068401,
-0.951796194676377));
#77929=CARTESIAN_POINT('Ctrl Pts',(0.155073160606334,-0.0121703475530541,
-0.951059641417123));
#77930=CARTESIAN_POINT('Ctrl Pts',(0.155880880035407,-0.00187848002803857,
-0.950320069168764));
#77931=CARTESIAN_POINT('Ctrl Pts',(0.155661426215852,0.00851759185665578,
-0.949580496920404));
#77932=CARTESIAN_POINT('Ctrl Pts',(0.154410120702099,0.0187967317574963,
-0.948840924672044));
#77933=CARTESIAN_POINT('Ctrl Pts',(0.153166842230774,0.0290099316531165,
-0.948106096730931));
#77934=CARTESIAN_POINT('Ctrl Pts',(0.150905032779441,0.0391067646233177,
-0.947371268789817));
#77935=CARTESIAN_POINT('Ctrl Pts',(0.147672136222049,0.0488747653049779,
-0.946636440848704));
#77936=CARTESIAN_POINT('Ctrl Pts',(0.144407930591391,0.0587373644507617,
-0.945894496446721));
#77937=CARTESIAN_POINT('Ctrl Pts',(0.140153999677468,0.0682638040917823,
-0.945152552044738));
#77938=CARTESIAN_POINT('Ctrl Pts',(0.135009692886142,0.0772540311361782,
-0.944410607642755));
#77939=CARTESIAN_POINT('Ctrl Pts',(0.129865386094816,0.0862442581805741,
-0.943668663240772));
#77940=CARTESIAN_POINT('Ctrl Pts',(0.123831294364284,0.0946975055529981,
-0.942926718838789));
#77941=CARTESIAN_POINT('Ctrl Pts',(0.117050458195957,0.102445071800046,
-0.942184774436806));
#77942=CARTESIAN_POINT('Ctrl Pts',(0.112492945464506,0.107652339890906,
-0.94168610126817));
#77943=CARTESIAN_POINT('Ctrl Pts',(0.107575895728917,0.112567881699699,
-0.941187428099533));
#77944=CARTESIAN_POINT('Ctrl Pts',(0.10234224283772,0.117140376604078,-0.940688754930896));
#77945=CARTESIAN_POINT('',(0.0903606778650181,-0.126612599672285,-0.9746));
#77946=CARTESIAN_POINT('Origin',(0.,0.,-0.9746));
#77947=CARTESIAN_POINT('Ctrl Pts',(0.0903606778650178,-0.126612599672286,
-0.9746));
#77948=CARTESIAN_POINT('Ctrl Pts',(0.0989423350469826,-0.120488056284229,
-0.973844886200287));
#77949=CARTESIAN_POINT('Ctrl Pts',(0.106910670833421,-0.113479022235499,
-0.973089772400574));
#77950=CARTESIAN_POINT('Ctrl Pts',(0.11409063599182,-0.105731401574849,
-0.972334658600861));
#77951=CARTESIAN_POINT('Ctrl Pts',(0.121274299065747,-0.0979797906376286,
-0.971579155892987));
#77952=CARTESIAN_POINT('Ctrl Pts',(0.127668165389618,-0.0894894421859699,
-0.970823653185113));
#77953=CARTESIAN_POINT('Ctrl Pts',(0.133134293154607,-0.0804429144562979,
-0.970068150477239));
#77954=CARTESIAN_POINT('Ctrl Pts',(0.138600356882239,-0.0713964927094613,
-0.96931265662031));
#77955=CARTESIAN_POINT('Ctrl Pts',(0.143138276591898,-0.0617946583516004,
-0.968557162763381));
#77956=CARTESIAN_POINT('Ctrl Pts',(0.146655326515842,-0.0518460963287661,
-0.967801668906452));
#77957=CARTESIAN_POINT('Ctrl Pts',(0.150183534797359,-0.0418659710313748,
-0.967043778134273));
#77958=CARTESIAN_POINT('Ctrl Pts',(0.15268414454631,-0.031537752234968,
-0.966285887362093));
#77959=CARTESIAN_POINT('Ctrl Pts',(0.154114131731867,-0.0210864150706726,
-0.965527996589914));
#77960=CARTESIAN_POINT('Ctrl Pts',(0.155379873755172,-0.011835495354623,
-0.964857155473916));
#77961=CARTESIAN_POINT('Ctrl Pts',(0.155807551061526,-0.00248871112968671,
-0.964186314357918));
#77962=CARTESIAN_POINT('Ctrl Pts',(0.155401438548432,0.00679671958212004,
-0.96351547324192));
#77963=CARTESIAN_POINT('Ctrl Pts',(0.154947224274956,0.0171819577333334,
-0.96276517474016));
#77964=CARTESIAN_POINT('Ctrl Pts',(0.15344503494107,0.0275697639167967,
-0.962014876238401));
#77965=CARTESIAN_POINT('Ctrl Pts',(0.150904946143938,0.0377292953723635,
-0.961264577736641));
#77966=CARTESIAN_POINT('Ctrl Pts',(0.148439190723746,0.0475915174259657,
-0.960536236034742));
#77967=CARTESIAN_POINT('Ctrl Pts',(0.144995737284637,0.0572376793730887,
-0.959807894332843));
#77968=CARTESIAN_POINT('Ctrl Pts',(0.140635976190268,0.0664629573597977,
-0.959079552630945));
#77969=CARTESIAN_POINT('Ctrl Pts',(0.136079069165201,0.07610539719902,-0.958318275729254));
#77970=CARTESIAN_POINT('Ctrl Pts',(0.130521124612019,0.0852868296405983,
-0.957556998827564));
#77971=CARTESIAN_POINT('Ctrl Pts',(0.124088333471531,0.0937970575031978,
-0.956795721925873));
#77972=CARTESIAN_POINT('Ctrl Pts',(0.117655542331043,0.102307285365797,
-0.956034445024183));
#77973=CARTESIAN_POINT('Ctrl Pts',(0.110348660155481,0.110145395632112,
-0.955273168122492));
#77974=CARTESIAN_POINT('Ctrl Pts',(0.10234224283772,0.117140376604078,-0.954511891220802));
#77975=CARTESIAN_POINT('Origin',(0.,0.,-1.10400562256037));
#77976=CARTESIAN_POINT('',(0.10234224283772,0.117140376604078,-0.870692680653027));
#77977=CARTESIAN_POINT('',(0.102342240207423,0.117140378902094,-0.884408356863363));
#77978=CARTESIAN_POINT('',(0.10234224283772,0.117140376604078,-1.10400562256037));
#77979=CARTESIAN_POINT('',(-0.155549990439246,5.45376069021774E-5,-0.915194377445425));
#77980=CARTESIAN_POINT('Ctrl Pts',(-0.155549990439274,5.45375255761138E-5,
-0.91519437743963));
#77981=CARTESIAN_POINT('Ctrl Pts',(-0.155553695565796,-0.0105130925417861,
-0.914441312361376));
#77982=CARTESIAN_POINT('Ctrl Pts',(-0.154476175611492,-0.0210724552290184,
-0.913688247283122));
#77983=CARTESIAN_POINT('Ctrl Pts',(-0.152348281357228,-0.0313975105302782,
-0.912935182204868));
#77984=CARTESIAN_POINT('Ctrl Pts',(-0.150212869444931,-0.0417590433185059,
-0.912179456615772));
#77985=CARTESIAN_POINT('Ctrl Pts',(-0.147019895179501,-0.051883773121568,
-0.911423731026675));
#77986=CARTESIAN_POINT('Ctrl Pts',(-0.142850970898113,-0.0615581238624639,
-0.910668005437579));
#77987=CARTESIAN_POINT('Ctrl Pts',(-0.139657291957392,-0.0689693331195593,
-0.910089068345908));
#77988=CARTESIAN_POINT('Ctrl Pts',(-0.135891972280923,-0.0761164594459378,
-0.909510131254238));
#77989=CARTESIAN_POINT('Ctrl Pts',(-0.131609697969464,-0.08291374976677,
-0.908931194162567));
#77990=CARTESIAN_POINT('Ctrl Pts',(-0.126153759250654,-0.091574007552026,
-0.908193584877298));
#77991=CARTESIAN_POINT('Ctrl Pts',(-0.119819100241729,-0.0997255876699728,
-0.907455975592029));
#77992=CARTESIAN_POINT('Ctrl Pts',(-0.11272431583233,-0.107186898080564,
-0.90671836630676));
#77993=CARTESIAN_POINT('Ctrl Pts',(-0.10561318980285,-0.114665394341068,
-0.905979058064904));
#77994=CARTESIAN_POINT('Ctrl Pts',(-0.0977389649286095,-0.121449664158534,
-0.905239749823048));
#77995=CARTESIAN_POINT('Ctrl Pts',(-0.0892626926281267,-0.127389066268564,
-0.904500441581192));
#77996=CARTESIAN_POINT('Ctrl Pts',(-0.0808251947826937,-0.133301298760633,
-0.903764515282857));
#77997=CARTESIAN_POINT('Ctrl Pts',(-0.0717919070181361,-0.138375838170688,
-0.903028588984522));
#77998=CARTESIAN_POINT('Ctrl Pts',(-0.0623530724919041,-0.142505778306774,
-0.902292662686187));
#77999=CARTESIAN_POINT('Ctrl Pts',(-0.0528491738308247,-0.146664187104025,
-0.90155166347257));
#78000=CARTESIAN_POINT('Ctrl Pts',(-0.0429349806278062,-0.149864532282499,
-0.900810664258953));
#78001=CARTESIAN_POINT('Ctrl Pts',(-0.0328243966067401,-0.152047234395774,
-0.900069665045336));
#78002=CARTESIAN_POINT('Ctrl Pts',(-0.022713812585674,-0.154229936509049,
-0.89932866583172));
#78003=CARTESIAN_POINT('Ctrl Pts',(-0.0124077867892572,-0.155394922432058,
-0.898587666618103));
#78004=CARTESIAN_POINT('Ctrl Pts',(-0.00212611195938367,-0.15553546909929,
-0.897846667404486));
#78005=CARTESIAN_POINT('Ctrl Pts',(0.0081081454405522,-0.155675367587907,
-0.897109085560012));
#78006=CARTESIAN_POINT('Ctrl Pts',(0.0183942801159778,-0.15480133283454,
-0.896371503715537));
#78007=CARTESIAN_POINT('Ctrl Pts',(0.0285154184472853,-0.152913941191692,
-0.895633921871063));
#78008=CARTESIAN_POINT('Ctrl Pts',(0.0386603406337221,-0.151022114331388,
-0.894894606769008));
#78009=CARTESIAN_POINT('Ctrl Pts',(0.048638551484433,-0.148112187289814,
-0.894155291666953));
#78010=CARTESIAN_POINT('Ctrl Pts',(0.0582359863388471,-0.144237208774787,
-0.893415976564898));
#78011=CARTESIAN_POINT('Ctrl Pts',(0.0677890842962877,-0.140380131347479,
-0.892680076848101));
#78012=CARTESIAN_POINT('Ctrl Pts',(0.0769640506140051,-0.135567245221165,
-0.891944177131304));
#78013=CARTESIAN_POINT('Ctrl Pts',(0.0855676359870254,-0.129899892885221,
-0.891208277414506));
#78014=CARTESIAN_POINT('Ctrl Pts',(0.0942311165291288,-0.124193086413391,
-0.890467254619823));
#78015=CARTESIAN_POINT('Ctrl Pts',(0.102314429869336,-0.117620382437007,
-0.889726231825139));
#78016=CARTESIAN_POINT('Ctrl Pts',(0.109651105763752,-0.110328770068312,
-0.888985209030456));
#78017=CARTESIAN_POINT('Ctrl Pts',(0.116987781658168,-0.103037157699618,
-0.888244186235772));
#78018=CARTESIAN_POINT('Ctrl Pts',(0.123577241802067,-0.0950273934776604,
-0.887503163441089));
#78019=CARTESIAN_POINT('Ctrl Pts',(0.129294154728679,-0.0864801945707602,
-0.886762140646405));
#78020=CARTESIAN_POINT('Ctrl Pts',(0.134984233931287,-0.0779731140248378,
-0.886024596022792));
#78021=CARTESIAN_POINT('Ctrl Pts',(0.139852269637792,-0.0688704151456475,
-0.885287051399179));
#78022=CARTESIAN_POINT('Ctrl Pts',(0.1437806382265,-0.0593542801420444,
-0.884549506775566));
#78023=CARTESIAN_POINT('Ctrl Pts',(0.147718486439882,-0.0498151815630685,
-0.883810182368296));
#78024=CARTESIAN_POINT('Ctrl Pts',(0.15071163599617,-0.0398614498671554,
-0.883070857961026));
#78025=CARTESIAN_POINT('Ctrl Pts',(0.152687987532983,-0.0297015313263073,
-0.882331533553756));
#78026=CARTESIAN_POINT('Ctrl Pts',(0.154655078065095,-0.0195892212456017,
-0.881595673553847));
#78027=CARTESIAN_POINT('Ctrl Pts',(0.155614697529464,-0.00927356739940421,
-0.880859813553937));
#78028=CARTESIAN_POINT('Ctrl Pts',(0.155546601845199,0.00102818014534441,
-0.880123953554028));
#78029=CARTESIAN_POINT('Ctrl Pts',(0.155478025272198,0.011402678179368,
-0.879382896943078));
#78030=CARTESIAN_POINT('Ctrl Pts',(0.154367154022987,0.0217621226354572,
-0.878641840332127));
#78031=CARTESIAN_POINT('Ctrl Pts',(0.152246624058229,0.0318867991945324,
-0.877900783721177));
#78032=CARTESIAN_POINT('Ctrl Pts',(0.15012609409347,0.0420114757536077,
-0.877159727110227));
#78033=CARTESIAN_POINT('Ctrl Pts',(0.146996225216177,0.0519004868433207,
-0.876418670499277));
#78034=CARTESIAN_POINT('Ctrl Pts',(0.142940364535494,0.0613502623177764,
-0.875677613888326));
#78035=CARTESIAN_POINT('Ctrl Pts',(0.138903416737029,0.0707559725482313,
-0.874940012898144));
#78036=CARTESIAN_POINT('Ctrl Pts',(0.133919123239017,0.0797964660534999,
-0.874202411907961));
#78037=CARTESIAN_POINT('Ctrl Pts',(0.128076264758454,0.0882738517655276,
-0.873464810917779));
#78038=CARTESIAN_POINT('Ctrl Pts',(0.12224578062805,0.0967332835703058,
-0.872728772062459));
#78039=CARTESIAN_POINT('Ctrl Pts',(0.115560796270105,0.104631174276986,
-0.871992733207139));
#78040=CARTESIAN_POINT('Ctrl Pts',(0.108154991620488,0.111795797271508,
-0.871256694351819));
#78041=CARTESIAN_POINT('Ctrl Pts',(0.106263345437786,0.113625839026497,
-0.871068689785555));
#78042=CARTESIAN_POINT('Ctrl Pts',(0.104324881639651,0.115408201007507,
-0.870880685219291));
#78043=CARTESIAN_POINT('Ctrl Pts',(0.10234224283772,0.117140376604078,-0.870692680653027));
#78044=CARTESIAN_POINT('Ctrl Pts',(0.10234224283772,0.117140376604078,-0.940688754930896));
#78045=CARTESIAN_POINT('Ctrl Pts',(0.0946113887193601,0.123894605781591,
-0.939952143313806));
#78046=CARTESIAN_POINT('Ctrl Pts',(0.0861883742852771,0.129898311105041,
-0.939215531696717));
#78047=CARTESIAN_POINT('Ctrl Pts',(0.0772432491414857,0.135015861890618,
-0.938478920079627));
#78048=CARTESIAN_POINT('Ctrl Pts',(0.0683023925004671,0.140130970644432,
-0.937742659964465));
#78049=CARTESIAN_POINT('Ctrl Pts',(0.0588406921375984,0.1443602554083,-0.937006399849303));
#78050=CARTESIAN_POINT('Ctrl Pts',(0.0490562919704071,0.147611932844585,
-0.936270139734141));
#78051=CARTESIAN_POINT('Ctrl Pts',(0.0392744119919948,0.15086277273939,
-0.935534069259064));
#78052=CARTESIAN_POINT('Ctrl Pts',(0.0291708820205725,0.153136232213258,
-0.934797998783987));
#78053=CARTESIAN_POINT('Ctrl Pts',(0.0189595642724556,0.154390211550469,
-0.93406192830891));
#78054=CARTESIAN_POINT('Ctrl Pts',(0.00872456505581199,0.155647099040471,
-0.93332415078385));
#78055=CARTESIAN_POINT('Ctrl Pts',(-0.00161779436127116,0.15587973642895,
-0.93258637325879));
#78056=CARTESIAN_POINT('Ctrl Pts',(-0.0118498928897874,0.155097977222466,
-0.93184859573373));
#78057=CARTESIAN_POINT('Ctrl Pts',(-0.0153094593003107,0.154833657260698,
-0.931599146382062));
#78058=CARTESIAN_POINT('Ctrl Pts',(-0.0187564643405992,0.154453813501656,
-0.931349697030394));
#78059=CARTESIAN_POINT('Ctrl Pts',(-0.0221827247955545,0.153960154652575,
-0.931100247678727));
#78060=CARTESIAN_POINT('Ctrl Pts',(-0.0323154695014615,0.152500219205368,
-0.930362531842254));
#78061=CARTESIAN_POINT('Ctrl Pts',(-0.0423409400692818,0.150030283649637,
-0.929624816005781));
#78062=CARTESIAN_POINT('Ctrl Pts',(-0.0520449532400662,0.14658487419321,
-0.928887100169308));
#78063=CARTESIAN_POINT('Ctrl Pts',(-0.0617695627278741,0.143132152015315,
-0.928147818565253));
#78064=CARTESIAN_POINT('Ctrl Pts',(-0.0711704273079884,0.138699984168947,
-0.927408536961198));
#78065=CARTESIAN_POINT('Ctrl Pts',(-0.0800444925456803,0.133374216822835,
-0.926669255357143));
#78066=CARTESIAN_POINT('Ctrl Pts',(-0.0888796922985958,0.128071774584683,
-0.925933211563173));
#78067=CARTESIAN_POINT('Ctrl Pts',(-0.0971918959959097,0.121884019072182,
-0.925197167769204));
#78068=CARTESIAN_POINT('Ctrl Pts',(-0.104806016875265,0.114941295132522,
-0.924461123975234));
#78069=CARTESIAN_POINT('Ctrl Pts',(-0.112470378808711,0.107952760287768,
-0.923720223466136));
#78070=CARTESIAN_POINT('Ctrl Pts',(-0.119426704616414,0.100199888626462,
-0.922979322957038));
#78071=CARTESIAN_POINT('Ctrl Pts',(-0.125533638113307,0.0918537326516312,
-0.92223842244794));
#78072=CARTESIAN_POINT('Ctrl Pts',(-0.131640571610199,0.0835075766768,-0.921497521938842));
#78073=CARTESIAN_POINT('Ctrl Pts',(-0.136897660774886,0.0745689720957777,
-0.920756621429744));
#78074=CARTESIAN_POINT('Ctrl Pts',(-0.141209383237786,0.0652358228705983,
-0.920015720920646));
#78075=CARTESIAN_POINT('Ctrl Pts',(-0.145885740973675,0.0551133845747866,
-0.919212163674776));
#78076=CARTESIAN_POINT('Ctrl Pts',(-0.149481238527706,0.0444612846556873,
-0.918408606428906));
#78077=CARTESIAN_POINT('Ctrl Pts',(-0.151896399595966,0.0335154634427567,
-0.917605049183036));
#78078=CARTESIAN_POINT('Ctrl Pts',(-0.154311560664225,0.0225696422298262,
-0.916801491937166));
#78079=CARTESIAN_POINT('Ctrl Pts',(-0.155546036882257,0.011330715400011,
-0.915997934691295));
#78080=CARTESIAN_POINT('Ctrl Pts',(-0.155549990439246,5.45376069020738E-5,
-0.915194377445425));
#78081=CARTESIAN_POINT('',(-0.155549963323784,0.000106817458056085,-0.929005622560371));
#78082=CARTESIAN_POINT('Ctrl Pts',(0.10234224283772,0.117140376604078,-0.954511891220802));
#78083=CARTESIAN_POINT('Ctrl Pts',(0.0950470821490095,0.123513952721795,
-0.953818242975148));
#78084=CARTESIAN_POINT('Ctrl Pts',(0.0871722852291945,0.129187673667992,
-0.953124594729494));
#78085=CARTESIAN_POINT('Ctrl Pts',(0.0788756227046464,0.134068783253054,
-0.952430946483841));
#78086=CARTESIAN_POINT('Ctrl Pts',(0.0700399201463668,0.13926702198102,
-0.951692231420943));
#78087=CARTESIAN_POINT('Ctrl Pts',(0.0606559263352574,0.14360701660631,
-0.950953516358044));
#78088=CARTESIAN_POINT('Ctrl Pts',(0.0509130047566652,0.146981864346074,
-0.950214801295146));
#78089=CARTESIAN_POINT('Ctrl Pts',(0.0411659057623924,0.150358159099627,
-0.949475769497697));
#78090=CARTESIAN_POINT('Ctrl Pts',(0.0310603979437165,0.152768056474797,
-0.948736737700248));
#78091=CARTESIAN_POINT('Ctrl Pts',(0.0208080947762397,0.154151956496773,
-0.947997705902799));
#78092=CARTESIAN_POINT('Ctrl Pts',(0.0105837859788066,0.155532077718154,
-0.947260692064561));
#78093=CARTESIAN_POINT('Ctrl Pts',(0.000214397467965564,0.155891654329331,
-0.946523678226324));
#78094=CARTESIAN_POINT('Ctrl Pts',(-0.010081436783493,0.155222959424115,
-0.945786664388086));
#78095=CARTESIAN_POINT('Ctrl Pts',(-0.0204195563472874,0.154551518168071,
-0.945046623611031));
#78096=CARTESIAN_POINT('Ctrl Pts',(-0.0306825824822815,0.152843406969938,
-0.944306582833977));
#78097=CARTESIAN_POINT('Ctrl Pts',(-0.0406543023893487,0.150143365478583,
-0.943566542056923));
#78098=CARTESIAN_POINT('Ctrl Pts',(-0.0506260222964158,0.147443323987229,
-0.942826501279868));
#78099=CARTESIAN_POINT('Ctrl Pts',(-0.0603055729763678,0.143751713730547,
-0.942086460502814));
#78100=CARTESIAN_POINT('Ctrl Pts',(-0.0694954311322223,0.139162450221842,
-0.941346419725759));
#78101=CARTESIAN_POINT('Ctrl Pts',(-0.0786704779145675,0.134580583268645,
-0.940607571678797));
#78102=CARTESIAN_POINT('Ctrl Pts',(-0.0874231978033075,0.129071120965396,
-0.939868723631834));
#78103=CARTESIAN_POINT('Ctrl Pts',(-0.0955609209755141,0.122735133039858,
-0.939129875584871));
#78104=CARTESIAN_POINT('Ctrl Pts',(-0.103700301814298,0.11639785446395,
-0.938390877033439));
#78105=CARTESIAN_POINT('Ctrl Pts',(-0.111223634830413,0.109234181245416,
-0.937651878482006));
#78106=CARTESIAN_POINT('Ctrl Pts',(-0.117966058921268,0.101389404981901,
-0.936912879930574));
#78107=CARTESIAN_POINT('Ctrl Pts',(-0.124692561830681,0.0935631529323152,
-0.936175626408802));
#78108=CARTESIAN_POINT('Ctrl Pts',(-0.130641222457451,0.0850597003544771,
-0.93543837288703));
#78109=CARTESIAN_POINT('Ctrl Pts',(-0.135686790429376,0.0760585130210588,
-0.934701119365258));
#78110=CARTESIAN_POINT('Ctrl Pts',(-0.140750272183004,0.0670253678771716,
-0.933961248298995));
#78111=CARTESIAN_POINT('Ctrl Pts',(-0.144903792076823,0.0574917680180006,
-0.933221377232732));
#78112=CARTESIAN_POINT('Ctrl Pts',(-0.148067614915439,0.0476632343977336,
-0.932481506166469));
#78113=CARTESIAN_POINT('Ctrl Pts',(-0.151231437754054,0.0378347007774667,
-0.931741635100206));
#78114=CARTESIAN_POINT('Ctrl Pts',(-0.153405400787358,0.0277121514410604,
-0.931001764033943));
#78115=CARTESIAN_POINT('Ctrl Pts',(-0.154561090975207,0.017512043186154,
-0.93026189296768));
#78116=CARTESIAN_POINT('Ctrl Pts',(-0.155215195656062,0.011738922824918,
-0.929843136165244));
#78117=CARTESIAN_POINT('Ctrl Pts',(-0.15554596577893,0.00592813137733295,
-0.929424379362807));
#78118=CARTESIAN_POINT('Ctrl Pts',(-0.155549963323784,0.000106817458056085,
-0.929005622560371));
#78119=CARTESIAN_POINT('Ctrl Pts',(-0.155549958606928,0.000113478556899634,
-0.92890670318866));
#78120=CARTESIAN_POINT('Ctrl Pts',(-0.15555842151029,-0.0114869885586137,
-0.928125533282183));
#78121=CARTESIAN_POINT('Ctrl Pts',(-0.154269217954487,-0.0230528665738872,
-0.927379180799272));
#78122=CARTESIAN_POINT('Ctrl Pts',(-0.150513718193053,-0.0396298028538525,
-0.926241852967461));
#78123=CARTESIAN_POINT('Ctrl Pts',(-0.149049117672017,-0.044824673419037,
-0.925875717519125));
#78124=CARTESIAN_POINT('Ctrl Pts',(-0.146757293093334,-0.0515863198642148,
-0.925379644446853));
#78125=CARTESIAN_POINT('Ctrl Pts',(-0.146168987948676,-0.0532304236852607,
-0.92525746973569));
#78126=CARTESIAN_POINT('Ctrl Pts',(-0.145139226726601,-0.0559623497425928,
-0.92505165225389));
#78127=CARTESIAN_POINT('Ctrl Pts',(-0.1447128985104,-0.0570557323292614,
-0.924968516834851));
#78128=CARTESIAN_POINT('Ctrl Pts',(-0.143846311692037,-0.0592060112854775,
-0.924803451688519));
#78129=CARTESIAN_POINT('Ctrl Pts',(-0.143406674663571,-0.0602630790138749,
-0.92472154729743));
#78130=CARTESIAN_POINT('Ctrl Pts',(-0.142406127794732,-0.062595839297176,
-0.924539060713868));
#78131=CARTESIAN_POINT('Ctrl Pts',(-0.141839668107321,-0.0638690272896489,
-0.924438294737681));
#78132=CARTESIAN_POINT('Ctrl Pts',(-0.139797417899609,-0.0682980312682417,
-0.92408355206488));
#78133=CARTESIAN_POINT('Ctrl Pts',(-0.138232886602676,-0.0714115161349304,
-0.923826580298416));
#78134=CARTESIAN_POINT('Ctrl Pts',(-0.130724420504484,-0.0851808277748374,
-0.922654677420037));
#78135=CARTESIAN_POINT('Ctrl Pts',(-0.123644260256459,-0.0951664776931758,
-0.921701866914742));
#78136=CARTESIAN_POINT('Ctrl Pts',(-0.112873075524329,-0.107100517719257,
-0.920460860689665));
#78137=CARTESIAN_POINT('Ctrl Pts',(-0.110166837651926,-0.109882318244648,
-0.920163377955844));
#78138=CARTESIAN_POINT('Ctrl Pts',(-0.106160694170145,-0.113703354844055,
-0.919745763824101));
#78139=CARTESIAN_POINT('Ctrl Pts',(-0.104943898542185,-0.114827368496542,
-0.919621728517606));
#78140=CARTESIAN_POINT('Ctrl Pts',(-0.102757422110185,-0.116783329100972,
-0.919404088725975));
#78141=CARTESIAN_POINT('Ctrl Pts',(-0.101795024295629,-0.11762315700496,
-0.919310026777228));
#78142=CARTESIAN_POINT('Ctrl Pts',(-0.100304733027344,-0.118891652662218,
-0.919167140697068));
#78143=CARTESIAN_POINT('Ctrl Pts',(-0.0997842198864589,-0.119328848352267,
-0.919117741711322));
#78144=CARTESIAN_POINT('Ctrl Pts',(-0.0987712684934094,-0.120168395810172,
-0.919022611287186));
#78145=CARTESIAN_POINT('Ctrl Pts',(-0.0982792248757209,-0.120571144173996,
-0.918976856533665));
#78146=CARTESIAN_POINT('Ctrl Pts',(-0.0971327282583652,-0.121497894651514,
-0.918871269731137));
#78147=CARTESIAN_POINT('Ctrl Pts',(-0.0964764885396974,-0.122019640005255,
-0.918811595098707));
#78148=CARTESIAN_POINT('Ctrl Pts',(-0.0942898170734549,-0.123729489257913,
-0.918615135912167));
#78149=CARTESIAN_POINT('Ctrl Pts',(-0.0927413373229463,-0.124894360761535,
-0.918479834861871));
#78150=CARTESIAN_POINT('Ctrl Pts',(-0.0820325027653891,-0.132641238757061,
-0.917566724344907));
#78151=CARTESIAN_POINT('Ctrl Pts',(-0.0722004711885394,-0.13823959997331,
-0.916837193149984));
#78152=CARTESIAN_POINT('Ctrl Pts',(-0.0569487009972901,-0.144848753469477,
-0.9157381921726));
#78153=CARTESIAN_POINT('Ctrl Pts',(-0.0519434028377933,-0.146718071010014,
-0.915382582329865));
#78154=CARTESIAN_POINT('Ctrl Pts',(-0.0434263309068883,-0.149408378661567,
-0.914775915053912));
#78155=CARTESIAN_POINT('Ctrl Pts',(-0.0399642777693343,-0.150371416958858,
-0.914528938529619));
#78156=CARTESIAN_POINT('Ctrl Pts',(-0.0349849308613356,-0.151572417561809,
-0.914171389992701));
#78157=CARTESIAN_POINT('Ctrl Pts',(-0.0334924983206864,-0.151909168314297,
-0.914063935441392));
#78158=CARTESIAN_POINT('Ctrl Pts',(-0.030876305638117,-0.152459056533917,
-0.913874941381056));
#78159=CARTESIAN_POINT('Ctrl Pts',(-0.0297546925034738,-0.152681918762541,
-0.913793715666761));
#78160=CARTESIAN_POINT('Ctrl Pts',(-0.0274188034895556,-0.153119339201618,
-0.913624087053861));
#78161=CARTESIAN_POINT('Ctrl Pts',(-0.0262042337487496,-0.153331864905213,
-0.913535626270902));
#78162=CARTESIAN_POINT('Ctrl Pts',(-0.023017402475677,-0.153850527967523,
-0.913302773887562));
#78163=CARTESIAN_POINT('Ctrl Pts',(-0.0210416083350701,-0.154133175567375,
-0.913157661256946));
#78164=CARTESIAN_POINT('Ctrl Pts',(-0.00974461085087905,-0.155528014957357,
-0.912323311217469));
#78165=CARTESIAN_POINT('Ctrl Pts',(-0.000344868758064268,-0.15583242440491,
-0.91160938709679));
#78166=CARTESIAN_POINT('Ctrl Pts',(0.0165438813602932,-0.154851060657897,
-0.910302674155081));
#78167=CARTESIAN_POINT('Ctrl Pts',(0.0240228052629501,-0.153868324355632,
-0.909715929865619));
#78168=CARTESIAN_POINT('Ctrl Pts',(0.0349236227189631,-0.151621494124985,
-0.908867518524567));
#78169=CARTESIAN_POINT('Ctrl Pts',(0.0384201141209241,-0.150773460572484,
-0.908596564898194));
#78170=CARTESIAN_POINT('Ctrl Pts',(0.0429060754647373,-0.149519218539199,
-0.908252953211336));
#78171=CARTESIAN_POINT('Ctrl Pts',(0.0439248875361686,-0.149223096214924,
-0.90817518938402));
#78172=CARTESIAN_POINT('Ctrl Pts',(0.0455875894249146,-0.14872131949046,
-0.908048815918406));
#78173=CARTESIAN_POINT('Ctrl Pts',(0.0462332895240024,-0.148521857539368,
-0.907999873114021));
#78174=CARTESIAN_POINT('Ctrl Pts',(0.0474454915087443,-0.148138727028628,
-0.90790826866143));
#78175=CARTESIAN_POINT('Ctrl Pts',(0.048012273645673,-0.147956002642827,
-0.907865553136803));
#78176=CARTESIAN_POINT('Ctrl Pts',(0.0495232473370512,-0.147459284270958,
-0.907751952195431));
#78177=CARTESIAN_POINT('Ctrl Pts',(0.0504655201013391,-0.147139471121678,
-0.907681394870265));
#78178=CARTESIAN_POINT('Ctrl Pts',(0.0540083180363241,-0.145898985756029,
-0.907416961297221));
#78179=CARTESIAN_POINT('Ctrl Pts',(0.0565874327973771,-0.14491817422107,
-0.907226194084785));
#78180=CARTESIAN_POINT('Ctrl Pts',(0.0686888153355076,-0.13994374572501,
-0.906333231584437));
#78181=CARTESIAN_POINT('Ctrl Pts',(0.0778246251406242,-0.135076913950358,
-0.905664045626618));
#78182=CARTESIAN_POINT('Ctrl Pts',(0.0916292727235142,-0.125854113764415,
-0.904565446489061));
#78183=CARTESIAN_POINT('Ctrl Pts',(0.0966309803781564,-0.122055822292311,
-0.904146332832308));
#78184=CARTESIAN_POINT('Ctrl Pts',(0.103502439801638,-0.116149951043788,
-0.903525641945619));
#78185=CARTESIAN_POINT('Ctrl Pts',(0.105566244601748,-0.114277436758061,
-0.903332825297031));
#78186=CARTESIAN_POINT('Ctrl Pts',(0.108582479215364,-0.111389315733298,
-0.903040393862723));
#78187=CARTESIAN_POINT('Ctrl Pts',(0.109573450010169,-0.110414642525321,
-0.902942508744874));
#78188=CARTESIAN_POINT('Ctrl Pts',(0.111343262674267,-0.108626645195505,
-0.902764281958235));
#78189=CARTESIAN_POINT('Ctrl Pts',(0.112126595735637,-0.107817886257278,
-0.902684144553977));
#78190=CARTESIAN_POINT('Ctrl Pts',(0.113800234515506,-0.106051957897308,
-0.902510139443805));
#78191=CARTESIAN_POINT('Ctrl Pts',(0.114687386248433,-0.105091933053241,
-0.9024161456162));
#78192=CARTESIAN_POINT('Ctrl Pts',(0.117100294653814,-0.102413879437565,
-0.902155505899546));
#78193=CARTESIAN_POINT('Ctrl Pts',(0.118600190079188,-0.100673112524103,
-0.901987813116794));
#78194=CARTESIAN_POINT('Ctrl Pts',(0.127276947925487,-0.09013983597288,
-0.900982625261368));
#78195=CARTESIAN_POINT('Ctrl Pts',(0.133511321274578,-0.0806179077762679,
-0.900108617563444));
#78196=CARTESIAN_POINT('Ctrl Pts',(0.141241602570841,-0.0654156670434553,
-0.898786769142857));
#78197=CARTESIAN_POINT('Ctrl Pts',(0.143547438384335,-0.0601875377353895,
-0.898344602034502));
#78198=CARTESIAN_POINT('Ctrl Pts',(0.146648259301679,-0.0519577249634245,
-0.897676800378137));
#78199=CARTESIAN_POINT('Ctrl Pts',(0.147649821725688,-0.0490392744700454,
-0.897445261816214));
#78200=CARTESIAN_POINT('Ctrl Pts',(0.148862017529785,-0.0451321805692637,
-0.89714384082322));
#78201=CARTESIAN_POINT('Ctrl Pts',(0.149150723171202,-0.0441687209002071,
-0.897070192712309));
#78202=CARTESIAN_POINT('Ctrl Pts',(0.149613954053185,-0.042566484172706,
-0.896948915333778));
#78203=CARTESIAN_POINT('Ctrl Pts',(0.149793778122319,-0.0419292847221374,
-0.8969009968103));
#78204=CARTESIAN_POINT('Ctrl Pts',(0.150129414352071,-0.0407102469382308,
-0.896809943620297));
#78205=CARTESIAN_POINT('Ctrl Pts',(0.150285923951169,-0.0401286226355811,
-0.89676676747304));
#78206=CARTESIAN_POINT('Ctrl Pts',(0.150702927809063,-0.0385422795841766,
-0.896649695699459));
#78207=CARTESIAN_POINT('Ctrl Pts',(0.150956756701925,-0.0375358165755575,
-0.896576168407868));
#78208=CARTESIAN_POINT('Ctrl Pts',(0.151931342057554,-0.0335015846534703,
-0.896284155252757));
#78209=CARTESIAN_POINT('Ctrl Pts',(0.152571283944592,-0.0304548090914521,
-0.896069688485559));
#78210=CARTESIAN_POINT('Ctrl Pts',(0.154680206779767,-0.0186654885958557,
-0.895255817057433));
#78211=CARTESIAN_POINT('Ctrl Pts',(0.15549249588109,-0.00982221229263341,
-0.894678100031022));
#78212=CARTESIAN_POINT('Ctrl Pts',(0.155596368136116,0.00705547200853701,
-0.893564403954027));
#78213=CARTESIAN_POINT('Ctrl Pts',(0.155026478307746,0.0150591704219786,
-0.893031400062748));
#78214=CARTESIAN_POINT('Ctrl Pts',(0.153494542755068,0.0253136736343002,
-0.892317405356613));
#78215=CARTESIAN_POINT('Ctrl Pts',(0.153093419290391,0.0276362205882911,
-0.892153659271439));
#78216=CARTESIAN_POINT('Ctrl Pts',(0.152388489219965,0.0312290467472916,
-0.891896699176937));
#78217=CARTESIAN_POINT('Ctrl Pts',(0.152121177132059,0.0325061885045768,
-0.89180463454713));
#78218=CARTESIAN_POINT('Ctrl Pts',(0.151593684669239,0.0348772314423096,
-0.891632287084306));
#78219=CARTESIAN_POINT('Ctrl Pts',(0.151337647220616,0.0359719740527535,
-0.891552141177227));
#78220=CARTESIAN_POINT('Ctrl Pts',(0.150738960129293,0.0384121845790077,
-0.891372166065112));
#78221=CARTESIAN_POINT('Ctrl Pts',(0.150390121939428,0.0397560186280247,
-0.8912721442879));
#78222=CARTESIAN_POINT('Ctrl Pts',(0.149449828631076,0.0431887009147026,
-0.891014230151929));
#78223=CARTESIAN_POINT('Ctrl Pts',(0.148832564837417,0.0452700997887852,
-0.890855525713056));
#78224=CARTESIAN_POINT('Ctrl Pts',(0.145471409157558,0.0557908465162443,
-0.890041107666606));
#78225=CARTESIAN_POINT('Ctrl Pts',(0.142052888732019,0.0639959328316331,
-0.889364166383715));
#78226=CARTESIAN_POINT('Ctrl Pts',(0.134522879154025,0.0784510369806034,
-0.888103850397088));
#78227=CARTESIAN_POINT('Ctrl Pts',(0.130623917018437,0.0847842466628702,
-0.887525118175059));
#78228=CARTESIAN_POINT('Ctrl Pts',(0.124875396044254,0.0927781560968537,
-0.886774399550553));
#78229=CARTESIAN_POINT('Ctrl Pts',(0.123417829154911,0.0947084555639051,
-0.886591479859804));
#78230=CARTESIAN_POINT('Ctrl Pts',(0.120843059062481,0.0979578529855939,
-0.886281675226426));
#78231=CARTESIAN_POINT('Ctrl Pts',(0.119747820664398,0.0992937358630493,
-0.886153739821052));
#78232=CARTESIAN_POINT('Ctrl Pts',(0.118106938789238,0.101228497572341,
-0.885967932821096));
#78233=CARTESIAN_POINT('Ctrl Pts',(0.117578552177343,0.101841749082174,
-0.885908960179795));
#78234=CARTESIAN_POINT('Ctrl Pts',(0.116627582185086,0.1029281884201,-0.885804385885963));
#78235=CARTESIAN_POINT('Ctrl Pts',(0.116206864855181,0.103402947254518,
-0.885758657679481));
#78236=CARTESIAN_POINT('Ctrl Pts',(0.115257902278136,0.104460697390482,
-0.885656704705278));
#78237=CARTESIAN_POINT('Ctrl Pts',(0.114728125867569,0.105042270265658,
-0.885600593770631));
#78238=CARTESIAN_POINT('Ctrl Pts',(0.113105532242885,0.10679658470307,-0.885431073735817));
#78239=CARTESIAN_POINT('Ctrl Pts',(0.111998939130881,0.107956519409209,
-0.885318628931571));
#78240=CARTESIAN_POINT('Ctrl Pts',(0.108131847055068,0.111886540242922,
-0.884935505996942));
#78241=CARTESIAN_POINT('Ctrl Pts',(0.105285666458265,0.114568790529068,
-0.884670242381571));
#78242=CARTESIAN_POINT('Ctrl Pts',(0.102342240207423,0.117140378902094,
-0.884408356863363));
#78243=CARTESIAN_POINT('Origin',(0.,0.,-1.10400562256037));
#78244=CARTESIAN_POINT('',(0.10234224283772,0.117140376604078,-0.800700826369365));
#78245=CARTESIAN_POINT('',(0.102342242814364,0.117140376624483,-0.814640372754811));
#78246=CARTESIAN_POINT('',(0.10234224283772,0.117140376604078,-1.10400562256037));
#78247=CARTESIAN_POINT('',(-0.155549936897438,-0.000140111395033391,-0.845194377435982));
#78248=CARTESIAN_POINT('Ctrl Pts',(-0.155549936897438,-0.000140111395033152,
-0.845194377435982));
#78249=CARTESIAN_POINT('Ctrl Pts',(-0.155538319828762,-0.0130372372788212,
-0.84427092949535));
#78250=CARTESIAN_POINT('Ctrl Pts',(-0.1539193025723,-0.0258623074908684,
-0.843347481554718));
#78251=CARTESIAN_POINT('Ctrl Pts',(-0.150765547234312,-0.0382825321411526,
-0.842424033614087));
#78252=CARTESIAN_POINT('Ctrl Pts',(-0.148246611384062,-0.0482026894732453,
-0.841686466531606));
#78253=CARTESIAN_POINT('Ctrl Pts',(-0.144735020415677,-0.0579100309946745,
-0.840948899449126));
#78254=CARTESIAN_POINT('Ctrl Pts',(-0.140287561326135,-0.0671952575496648,
-0.840211332366645));
#78255=CARTESIAN_POINT('Ctrl Pts',(-0.135829539592097,-0.0765025363698251,
-0.839472013574092));
#78256=CARTESIAN_POINT('Ctrl Pts',(-0.130431466357588,-0.0853847925415279,
-0.838732694781539));
#78257=CARTESIAN_POINT('Ctrl Pts',(-0.124200087059014,-0.0936490302914732,
-0.837993375988985));
#78258=CARTESIAN_POINT('Ctrl Pts',(-0.117997662165273,-0.101874867861623,
-0.837257492476904));
#78259=CARTESIAN_POINT('Ctrl Pts',(-0.110970216967241,-0.109487670969301,
-0.836521608964823));
#78260=CARTESIAN_POINT('Ctrl Pts',(-0.103265733734167,-0.116327085136455,
-0.835785725452742));
#78261=CARTESIAN_POINT('Ctrl Pts',(-0.0955073009417575,-0.12321439133858,
-0.835044689019953));
#78262=CARTESIAN_POINT('Ctrl Pts',(-0.0870630130899514,-0.129316795090957,
-0.834303652587163));
#78263=CARTESIAN_POINT('Ctrl Pts',(-0.0781180168921039,-0.134511627515412,
-0.833562616154374));
#78264=CARTESIAN_POINT('Ctrl Pts',(-0.0691730206942564,-0.139706459939867,
-0.832821579721584));
#78265=CARTESIAN_POINT('Ctrl Pts',(-0.0597281969952501,-0.143993358605103,
-0.832080543288795));
#78266=CARTESIAN_POINT('Ctrl Pts',(-0.0499906020627426,-0.14729814053614,
-0.831339506856006));
#78267=CARTESIAN_POINT('Ctrl Pts',(-0.0402986120533905,-0.150587444895245,
-0.830601940983432));
#78268=CARTESIAN_POINT('Ctrl Pts',(-0.0302445674700445,-0.152928295698067,
-0.829864375110859));
#78269=CARTESIAN_POINT('Ctrl Pts',(-0.0200349361239818,-0.154254347862574,
-0.829126809238286));
#78270=CARTESIAN_POINT('Ctrl Pts',(-0.00980103609139822,-0.155583552104095,
-0.828387490143256));
#78271=CARTESIAN_POINT('Ctrl Pts',(0.000588290641111029,-0.15589286142406,
-0.827648171048226));
#78272=CARTESIAN_POINT('Ctrl Pts',(0.0109130440681473,-0.155166710247935,
-0.826908851953196));
#78273=CARTESIAN_POINT('Ctrl Pts',(0.0211898017065059,-0.154443934668007,
-0.826172969666928));
#78274=CARTESIAN_POINT('Ctrl Pts',(0.0314016544816177,-0.15269536639436,
-0.825437087380661));
#78275=CARTESIAN_POINT('Ctrl Pts',(0.0413335254017949,-0.14995780132377,
-0.824701205094393));
#78276=CARTESIAN_POINT('Ctrl Pts',(0.0513349739058709,-0.147201058279069,
-0.823960167594982));
#78277=CARTESIAN_POINT('Ctrl Pts',(0.0610515833788873,-0.143441647462304,
-0.823219130095571));
#78278=CARTESIAN_POINT('Ctrl Pts',(0.0702796451137023,-0.138768058221956,
-0.822478092596159));
#78279=CARTESIAN_POINT('Ctrl Pts',(0.079507706848517,-0.134094468981608,
-0.821737055096748));
#78280=CARTESIAN_POINT('Ctrl Pts',(0.0882464371862269,-0.128507242758074,
-0.820996017597337));
#78281=CARTESIAN_POINT('Ctrl Pts',(0.0963208635534173,-0.122139648535289,
-0.820254980097926));
#78282=CARTESIAN_POINT('Ctrl Pts',(0.104357457510738,-0.115801889426922,
-0.81951741470082));
#78283=CARTESIAN_POINT('Ctrl Pts',(0.111795714032649,-0.108643985892654,
-0.818779849303714));
#78284=CARTESIAN_POINT('Ctrl Pts',(0.118467555690701,-0.100802979860075,
-0.818042283906609));
#78285=CARTESIAN_POINT('Ctrl Pts',(0.125155261959505,-0.0929433291241313,
-0.817302964692712));
#78286=CARTESIAN_POINT('Ctrl Pts',(0.131072190559215,-0.0843979338543903,
-0.816563645478815));
#78287=CARTESIAN_POINT('Ctrl Pts',(0.1360854849751,-0.0753428382734008,
-0.815824326264918));
#78288=CARTESIAN_POINT('Ctrl Pts',(0.141075470205837,-0.0663298441294938,
-0.815088444496942));
#78289=CARTESIAN_POINT('Ctrl Pts',(0.145169750922882,-0.056812693240137,
-0.814352562728965));
#78290=CARTESIAN_POINT('Ctrl Pts',(0.148282068834788,-0.0469918137772452,
-0.813616680960989));
#78291=CARTESIAN_POINT('Ctrl Pts',(0.151416194104158,-0.0371021214761001,
-0.812875643024132));
#78292=CARTESIAN_POINT('Ctrl Pts',(0.153554242780962,-0.0269053291409457,
-0.812134605087275));
#78293=CARTESIAN_POINT('Ctrl Pts',(0.154659503832709,-0.0166204805652641,
-0.811393567150417));
#78294=CARTESIAN_POINT('Ctrl Pts',(0.155764764884456,-0.00633563198958233,
-0.81065252921356));
#78295=CARTESIAN_POINT('Ctrl Pts',(0.155837265691724,0.00403632070063776,
-0.809911491276702));
#78296=CARTESIAN_POINT('Ctrl Pts',(0.154893501714532,0.0142760508058142,
-0.809170453339845));
#78297=CARTESIAN_POINT('Ctrl Pts',(0.153954014253801,0.0244693812015213,
-0.808432773298618));
#78298=CARTESIAN_POINT('Ctrl Pts',(0.152000507162109,0.0346074596889915,
-0.807695093257391));
#78299=CARTESIAN_POINT('Ctrl Pts',(0.149056410292548,0.0444745888199042,
-0.806957413216164));
#78300=CARTESIAN_POINT('Ctrl Pts',(0.146118584279151,0.0543207012009377,
-0.806221304415843));
#78301=CARTESIAN_POINT('Ctrl Pts',(0.142194543330265,0.0638961073393962,
-0.805485195615522));
#78302=CARTESIAN_POINT('Ctrl Pts',(0.137358517895996,0.072996164703465,
-0.804749086815201));
#78303=CARTESIAN_POINT('Ctrl Pts',(0.132521054937009,0.0820989270899887,
-0.80401275920408));
#78304=CARTESIAN_POINT('Ctrl Pts',(0.126771460493011,0.0907252182537294,
-0.803276431592959));
#78305=CARTESIAN_POINT('Ctrl Pts',(0.12023091747951,0.0986931050379669,
-0.802540103981838));
#78306=CARTESIAN_POINT('Ctrl Pts',(0.114785028921007,0.105327450746598,
-0.801927011444347));
#78307=CARTESIAN_POINT('Ctrl Pts',(0.108791818876103,0.111505563943781,
-0.801313918906856));
#78308=CARTESIAN_POINT('Ctrl Pts',(0.10234224283772,0.117140376604078,-0.800700826369366));
#78309=CARTESIAN_POINT('Ctrl Pts',(0.10234224283772,0.117140376604078,-0.870692680653027));
#78310=CARTESIAN_POINT('Ctrl Pts',(0.0945823687409577,0.123919959718149,
-0.869956847296794));
#78311=CARTESIAN_POINT('Ctrl Pts',(0.0861434261176855,0.129927435099362,
-0.86922101394056));
#78312=CARTESIAN_POINT('Ctrl Pts',(0.0772043632031639,0.135038101298833,
-0.868485180584327));
#78313=CARTESIAN_POINT('Ctrl Pts',(0.06824357246428,0.14016118979118,-0.867747558667248));
#78314=CARTESIAN_POINT('Ctrl Pts',(0.0587810565339102,0.144382678263256,
-0.867009936750168));
#78315=CARTESIAN_POINT('Ctrl Pts',(0.0490207580366101,0.147623737188557,
-0.866272314833089));
#78316=CARTESIAN_POINT('Ctrl Pts',(0.0416141796594417,0.150083206738787,
-0.865712572265475));
#78317=CARTESIAN_POINT('Ctrl Pts',(0.0340367145713927,0.15197906578916,
-0.86515282969786));
#78318=CARTESIAN_POINT('Ctrl Pts',(0.0263818859332598,0.153296440254184,
-0.864593087130246));
#78319=CARTESIAN_POINT('Ctrl Pts',(0.0162951940079565,0.155032331546741,
-0.8638555198895));
#78320=CARTESIAN_POINT('Ctrl Pts',(0.00599895782048205,0.155774870891324,
-0.863117952648755));
#78321=CARTESIAN_POINT('Ctrl Pts',(-0.00429252786504568,0.15549076083333,
-0.86238038540801));
#78322=CARTESIAN_POINT('Ctrl Pts',(-0.014608452899512,0.155205976094823,
-0.861641066655023));
#78323=CARTESIAN_POINT('Ctrl Pts',(-0.0249186737362951,0.15388953793924,
-0.860901747902036));
#78324=CARTESIAN_POINT('Ctrl Pts',(-0.0350034587763083,0.151560418228821,
-0.860162429149049));
#78325=CARTESIAN_POINT('Ctrl Pts',(-0.0450413890419768,0.149242119807902,
-0.859426545334259));
#78326=CARTESIAN_POINT('Ctrl Pts',(-0.0548550642084026,0.145920735726236,
-0.858690661519468));
#78327=CARTESIAN_POINT('Ctrl Pts',(-0.0642377884513287,0.141666188749759,
-0.857954777704678));
#78328=CARTESIAN_POINT('Ctrl Pts',(-0.0736862073268392,0.137381852887539,
-0.857213741482593));
#78329=CARTESIAN_POINT('Ctrl Pts',(-0.0826967467014411,0.132151616254013,
-0.856472705260507));
#78330=CARTESIAN_POINT('Ctrl Pts',(-0.0910820121346721,0.126094684921687,
-0.855731669038422));
#78331=CARTESIAN_POINT('Ctrl Pts',(-0.0994672775679031,0.12003775358936,
-0.854990632816337));
#78332=CARTESIAN_POINT('Ctrl Pts',(-0.107226579556024,0.113154784688802,
-0.854249596594251));
#78333=CARTESIAN_POINT('Ctrl Pts',(-0.114207897837056,0.105604727979577,
-0.853508560372166));
#78334=CARTESIAN_POINT('Ctrl Pts',(-0.121078206097479,0.0981747248071135,
-0.852779307375394));
#78335=CARTESIAN_POINT('Ctrl Pts',(-0.127248819633919,0.0900404725511059,
-0.852050054378621));
#78336=CARTESIAN_POINT('Ctrl Pts',(-0.13257631495945,0.0813592232741483,
-0.851320801381849));
#78337=CARTESIAN_POINT('Ctrl Pts',(-0.137892545783061,0.0726963297052993,
-0.850593090323882));
#78338=CARTESIAN_POINT('Ctrl Pts',(-0.142368631298909,0.0634894916783257,
-0.849865379265916));
#78339=CARTESIAN_POINT('Ctrl Pts',(-0.145903110021304,0.0539266630351919,
-0.84913766820795));
#78340=CARTESIAN_POINT('Ctrl Pts',(-0.149439269993569,0.0443592856295196,
-0.848409610998764));
#78341=CARTESIAN_POINT('Ctrl Pts',(-0.152032558253122,0.0344364565318959,
-0.847681553789577));
#78342=CARTESIAN_POINT('Ctrl Pts',(-0.153629756766561,0.0243659667538019,
-0.846953496580391));
#78343=CARTESIAN_POINT('Ctrl Pts',(-0.154916131170997,0.0162552527870187,
-0.846367123533471));
#78344=CARTESIAN_POINT('Ctrl Pts',(-0.155557313527155,0.00804933460988067,
-0.84578075048655));
#78345=CARTESIAN_POINT('Ctrl Pts',(-0.155549936897484,-0.000140111344081384,
-0.84519437743963));
#78346=CARTESIAN_POINT('Ctrl Pts',(0.102342240207423,0.117140378902094,
-0.884408356863363));
#78347=CARTESIAN_POINT('Ctrl Pts',(0.0997671282763309,0.119390181457651,
-0.884179241381932));
#78348=CARTESIAN_POINT('Ctrl Pts',(0.0971175853369499,0.121555284170953,
-0.883952710064294));
#78349=CARTESIAN_POINT('Ctrl Pts',(0.0890846091051486,0.127688771197036,
-0.883285685527337));
#78350=CARTESIAN_POINT('Ctrl Pts',(0.0835155932020043,0.131398754954517,
-0.882847875137769));
#78351=CARTESIAN_POINT('Ctrl Pts',(0.0725185033115193,0.137742517529728,
-0.882001156533603));
#78352=CARTESIAN_POINT('Ctrl Pts',(0.0671425600539784,0.140441440762792,
-0.881594546776866));
#78353=CARTESIAN_POINT('Ctrl Pts',(0.0599616565701782,0.143539825929432,
-0.881051536440173));
#78354=CARTESIAN_POINT('Ctrl Pts',(0.0582865847286211,0.144228136828107,
-0.880924901066003));
#78355=CARTESIAN_POINT('Ctrl Pts',(0.055488758935558,0.14532110402266,-0.880713222267803));
#78356=CARTESIAN_POINT('Ctrl Pts',(0.0543726526414778,0.145742375941171,
-0.880628737717708));
#78357=CARTESIAN_POINT('Ctrl Pts',(0.0521746009066699,0.146543263309774,
-0.880462214047268));
#78358=CARTESIAN_POINT('Ctrl Pts',(0.0510930837640482,0.146923836268053,
-0.880380212840648));
#78359=CARTESIAN_POINT('Ctrl Pts',(0.0487055126520772,0.147734444401238,
-0.880198994134006));
#78360=CARTESIAN_POINT('Ctrl Pts',(0.0473977770678758,0.148159183077436,
-0.880099610653952));
#78361=CARTESIAN_POINT('Ctrl Pts',(0.0429029277076668,0.149553463774429,
-0.879757494595172));
#78362=CARTESIAN_POINT('Ctrl Pts',(0.0396905910409664,0.15043787298108,
-0.879512077143425));
#78363=CARTESIAN_POINT('Ctrl Pts',(0.0244892534603979,0.154102291398103,
-0.878345747661989));
#78364=CARTESIAN_POINT('Ctrl Pts',(0.0122272967379565,0.155555917668405,
-0.877385815592969));
#78365=CARTESIAN_POINT('Ctrl Pts',(-0.00395682392747703,0.155548108973284,
-0.876137357943913));
#78366=CARTESIAN_POINT('Ctrl Pts',(-0.00783742415145313,0.155400930795403,
-0.875839861719982));
#78367=CARTESIAN_POINT('Ctrl Pts',(-0.0141161428952155,0.154926969635022,
-0.875365066384795));
#78368=CARTESIAN_POINT('Ctrl Pts',(-0.0165192227783718,0.154689199107901,
-0.875184920615359));
#78369=CARTESIAN_POINT('Ctrl Pts',(-0.0198307495234539,0.154283483517612,
-0.874939683428125));
#78370=CARTESIAN_POINT('Ctrl Pts',(-0.0207445615505518,0.15416327445371,
-0.874872329212308));
#78371=CARTESIAN_POINT('Ctrl Pts',(-0.022297935207071,0.153944870448678,
-0.87475843765664));
#78372=CARTESIAN_POINT('Ctrl Pts',(-0.0229380407323316,0.153850795921362,
-0.874711681576258));
#78373=CARTESIAN_POINT('Ctrl Pts',(-0.0242864240581363,0.153644024918888,
-0.874613579798878));
#78374=CARTESIAN_POINT('Ctrl Pts',(-0.024994534615702,0.153530420701988,
-0.87456228389501));
#78375=CARTESIAN_POINT('Ctrl Pts',(-0.026945898851513,0.153203499061469,
-0.874421477394967));
#78376=CARTESIAN_POINT('Ctrl Pts',(-0.0281874157381815,0.1529799446005,
-0.874332510943112));
#78377=CARTESIAN_POINT('Ctrl Pts',(-0.0370025397288145,0.15128168122978,
-0.873704341384225));
#78378=CARTESIAN_POINT('Ctrl Pts',(-0.0444609586518216,0.149260146615439,
-0.873191099903673));
#78379=CARTESIAN_POINT('Ctrl Pts',(-0.0575259777953991,0.144652046449809,
-0.872276380153128));
#78380=CARTESIAN_POINT('Ctrl Pts',(-0.0631866447456239,0.142270514328931,
-0.871874391579915));
#78381=CARTESIAN_POINT('Ctrl Pts',(-0.0726669278005061,0.137604323624873,
-0.871171998524482));
#78382=CARTESIAN_POINT('Ctrl Pts',(-0.0765563933905407,0.135478952118518,
-0.870874802023289));
#78383=CARTESIAN_POINT('Ctrl Pts',(-0.0830527535334971,0.131559904896758,
-0.870357239933504));
#78384=CARTESIAN_POINT('Ctrl Pts',(-0.0857054190130834,0.129847400029952,
-0.870139485435968));
#78385=CARTESIAN_POINT('Ctrl Pts',(-0.089502773244607,0.127228835022822,
-0.869817003896838));
#78386=CARTESIAN_POINT('Ctrl Pts',(-0.0906898368429427,0.126385426850809,
-0.869714599276118));
#78387=CARTESIAN_POINT('Ctrl Pts',(-0.092777725646137,0.124857421873039,
-0.869531510048099));
#78388=CARTESIAN_POINT('Ctrl Pts',(-0.0936832633564158,0.124179419458814,
-0.869451082492525));
#78389=CARTESIAN_POINT('Ctrl Pts',(-0.0955837069435231,0.122723883948887,
-0.869280064118647));
#78390=CARTESIAN_POINT('Ctrl Pts',(-0.096576696592691,0.121943996271376,
-0.869189384796161));
#78391=CARTESIAN_POINT('Ctrl Pts',(-0.0992330214888864,0.11980494010852,
-0.868943136814336));
#78392=CARTESIAN_POINT('Ctrl Pts',(-0.100877821880938,0.118423310335433,
-0.868786681553506));
#78393=CARTESIAN_POINT('Ctrl Pts',(-0.112088202102204,0.10860356397806,
-0.867691708277005));
#78394=CARTESIAN_POINT('Ctrl Pts',(-0.1206110683486,0.0990522134992969,
-0.866705139288486));
#78395=CARTESIAN_POINT('Ctrl Pts',(-0.131646621599032,0.0831200044697117,
-0.8652044475045));
#78396=CARTESIAN_POINT('Ctrl Pts',(-0.135070139394415,0.0774328280398601,
-0.86469354213076));
#78397=CARTESIAN_POINT('Ctrl Pts',(-0.138855693315738,0.0701245624971615,
-0.864079780611562));
#78398=CARTESIAN_POINT('Ctrl Pts',(-0.1395690434261,0.0686938168425374,
-0.863961574871956));
#78399=CARTESIAN_POINT('Ctrl Pts',(-0.140599945018185,0.0665437847546757,
-0.863787096766562));
#78400=CARTESIAN_POINT('Ctrl Pts',(-0.140934281721406,0.0658327284511854,
-0.863729900603186));
#78401=CARTESIAN_POINT('Ctrl Pts',(-0.141502424124003,0.0646002549072531,
-0.863631673002615));
#78402=CARTESIAN_POINT('Ctrl Pts',(-0.141738759784731,0.0640800512791535,
-0.863590493218231));
#78403=CARTESIAN_POINT('Ctrl Pts',(-0.142290043716558,0.0628486349069057,
-0.863493670488512));
#78404=CARTESIAN_POINT('Ctrl Pts',(-0.142602531019311,0.0621363473822941,
-0.863438175058531));
#78405=CARTESIAN_POINT('Ctrl Pts',(-0.143524812051775,0.0599904799806183,
-0.863272423990894));
#78406=CARTESIAN_POINT('Ctrl Pts',(-0.144118447906321,0.0585500027093065,
-0.863163071607694));
#78407=CARTESIAN_POINT('Ctrl Pts',(-0.147946243807693,0.048850569272976,
-0.862437886456258));
#78408=CARTESIAN_POINT('Ctrl Pts',(-0.150490969000253,0.0403358387532395,
-0.861854293833215));
#78409=CARTESIAN_POINT('Ctrl Pts',(-0.154456532512761,0.0212537731323482,
-0.860570491332088));
#78410=CARTESIAN_POINT('Ctrl Pts',(-0.155546637215152,0.0106653881160218,
-0.859872051404209));
#78411=CARTESIAN_POINT('Ctrl Pts',(-0.155550662972886,-0.00207321574764465,
-0.858991922614664));
#78412=CARTESIAN_POINT('Ctrl Pts',(-0.155507896198807,-0.00419528657780355,
-0.85884408058168));
#78413=CARTESIAN_POINT('Ctrl Pts',(-0.155370685355025,-0.00757186267443317,
-0.858606536825204));
#78414=CARTESIAN_POINT('Ctrl Pts',(-0.155304416114564,-0.00882729527448303,
-0.858517709903541));
#78415=CARTESIAN_POINT('Ctrl Pts',(-0.155149559113993,-0.0112115388778581,
-0.858347982177621));
#78416=CARTESIAN_POINT('Ctrl Pts',(-0.155063848826277,-0.0123404603062701,
-0.858267176330289));
#78417=CARTESIAN_POINT('Ctrl Pts',(-0.154838926148483,-0.0149284097686903,
-0.858080873451588));
#78418=CARTESIAN_POINT('Ctrl Pts',(-0.154691402416279,-0.0163865864669549,
-0.857975123887429));
#78419=CARTESIAN_POINT('Ctrl Pts',(-0.154154765621627,-0.021034101086388,
-0.857635478570857));
#78420=CARTESIAN_POINT('Ctrl Pts',(-0.153687459278953,-0.0242133691343534,
-0.857399194350234));
#78421=CARTESIAN_POINT('Ctrl Pts',(-0.152322614182279,-0.0318474405099905,
-0.856821904163447));
#78422=CARTESIAN_POINT('Ctrl Pts',(-0.151327704693815,-0.0362816411973021,
-0.8564782751213));
#78423=CARTESIAN_POINT('Ctrl Pts',(-0.148559496246306,-0.0465020596157439,
-0.855668085080076));
#78424=CARTESIAN_POINT('Ctrl Pts',(-0.14663977828123,-0.0522411195865409,
-0.85519905851238));
#78425=CARTESIAN_POINT('Ctrl Pts',(-0.141556398189741,-0.0649282239794905,
-0.854140253815778));
#78426=CARTESIAN_POINT('Ctrl Pts',(-0.138205332782677,-0.0717857935177119,
-0.853552062493638));
#78427=CARTESIAN_POINT('Ctrl Pts',(-0.133731201897603,-0.0794565829015627,
-0.852893974340787));
#78428=CARTESIAN_POINT('Ctrl Pts',(-0.133084644076084,-0.0805348415629863,
-0.852801479481863));
#78429=CARTESIAN_POINT('Ctrl Pts',(-0.132049377513543,-0.0822148234197764,
-0.852657522278592));
#78430=CARTESIAN_POINT('Ctrl Pts',(-0.131669481939945,-0.0828218743580949,
-0.852605536468524));
#78431=CARTESIAN_POINT('Ctrl Pts',(-0.130938461524903,-0.0839722587121252,
-0.852507114644129));
#78432=CARTESIAN_POINT('Ctrl Pts',(-0.130588133545813,-0.0845160359553828,
-0.852460635436555));
#78433=CARTESIAN_POINT('Ctrl Pts',(-0.129729846967908,-0.0858301853310774,
-0.852348382684133));
#78434=CARTESIAN_POINT('Ctrl Pts',(-0.129218407138713,-0.0865982521501915,
-0.852282835621129));
#78435=CARTESIAN_POINT('Ctrl Pts',(-0.12733852067511,-0.0893676755047455,
-0.852046532388373));
#78436=CARTESIAN_POINT('Ctrl Pts',(-0.125930088463256,-0.0913416374443751,
-0.851878178488348));
#78437=CARTESIAN_POINT('Ctrl Pts',(-0.122133443362587,-0.0964079005467835,
-0.851443969903988));
#78438=CARTESIAN_POINT('Ctrl Pts',(-0.119673813856034,-0.0994446770489137,
-0.851181539686132));
#78439=CARTESIAN_POINT('Ctrl Pts',(-0.108884178413976,-0.111785166226848,
-0.850090792539563));
#78440=CARTESIAN_POINT('Ctrl Pts',(-0.0995647974595149,-0.120160454955035,
-0.849285448836767));
#78441=CARTESIAN_POINT('Ctrl Pts',(-0.0869332712028222,-0.129023584407323,
-0.848234002348013));
#78442=CARTESIAN_POINT('Ctrl Pts',(-0.0844746116981484,-0.130646535008912,
-0.84803122726872));
#78443=CARTESIAN_POINT('Ctrl Pts',(-0.0806125329624861,-0.133041267370624,
-0.847714492311786));
#78444=CARTESIAN_POINT('Ctrl Pts',(-0.0792407124934048,-0.133862871799446,
-0.847602325732475));
#78445=CARTESIAN_POINT('Ctrl Pts',(-0.0768688834660482,-0.135234162530654,
-0.847408822482591));
#78446=CARTESIAN_POINT('Ctrl Pts',(-0.0758750260699779,-0.13579427180251,
-0.847327866271435));
#78447=CARTESIAN_POINT('Ctrl Pts',(-0.0738223906530052,-0.136921508926426,
-0.84716087214164));
#78448=CARTESIAN_POINT('Ctrl Pts',(-0.0727630277661404,-0.137487405277673,
-0.847074797433248));
#78449=CARTESIAN_POINT('Ctrl Pts',(-0.0700536867930569,-0.138894612808811,
-0.846854879198575));
#78450=CARTESIAN_POINT('Ctrl Pts',(-0.0683950827528329,-0.139718805495557,
-0.846720452145391));
#78451=CARTESIAN_POINT('Ctrl Pts',(-0.0608172248132356,-0.143317127094337,
-0.846106918717946));
#78452=CARTESIAN_POINT('Ctrl Pts',(-0.0547421791731601,-0.145745690069455,
-0.845616403006151));
#78453=CARTESIAN_POINT('Ctrl Pts',(-0.0426330918047611,-0.149722366343413,
-0.844642642465732));
#78454=CARTESIAN_POINT('Ctrl Pts',(-0.0366225663557615,-0.151304817116957,
-0.844161154393155));
#78455=CARTESIAN_POINT('Ctrl Pts',(-0.0234821047226767,-0.153935421569936,
-0.843122885561882));
#78456=CARTESIAN_POINT('Ctrl Pts',(-0.0163401850692006,-0.154856519753629,
-0.842567370507838));
#78457=CARTESIAN_POINT('Ctrl Pts',(-0.00756115771862474,-0.155374370978998,
-0.841911547290137));
#78458=CARTESIAN_POINT('Ctrl Pts',(-0.00596131666418646,-0.15544397541448,
-0.841793143905305));
#78459=CARTESIAN_POINT('Ctrl Pts',(-0.00357461197005635,-0.155510909334888,
-0.841618427000853));
#78460=CARTESIAN_POINT('Ctrl Pts',(-0.00278843905428665,-0.155526992678888,
-0.841561186546572));
#78461=CARTESIAN_POINT('Ctrl Pts',(-0.00136746486178335,-0.155545284206716,
-0.841458327982413));
#78462=CARTESIAN_POINT('Ctrl Pts',(-0.000732740710060755,-0.155549569351714,
-0.841412603273821));
#78463=CARTESIAN_POINT('Ctrl Pts',(0.000712877770075411,-0.155550479842053,
-0.841308956398088));
#78464=CARTESIAN_POINT('Ctrl Pts',(0.00152374054465577,-0.155544650392086,
-0.841251168197913));
#78465=CARTESIAN_POINT('Ctrl Pts',(0.00406633944534416,-0.155506485953609,
-0.841070951163574));
#78466=CARTESIAN_POINT('Ctrl Pts',(0.00579767349409387,-0.155451567759823,
-0.84094967271617));
#78467=CARTESIAN_POINT('Ctrl Pts',(0.00995174313134238,-0.155250296299062,
-0.840661354013299));
#78468=CARTESIAN_POINT('Ctrl Pts',(0.0123727255873134,-0.155076138383495,
-0.840495505375031));
#78469=CARTESIAN_POINT('Ctrl Pts',(0.0222313210250158,-0.154134576357237,
-0.839825477031806));
#78470=CARTESIAN_POINT('Ctrl Pts',(0.0296134357082729,-0.152888059379158,
-0.839335812474905));
#78471=CARTESIAN_POINT('Ctrl Pts',(0.0454168440599835,-0.149031448714727,
-0.838263783535376));
#78472=CARTESIAN_POINT('Ctrl Pts',(0.0537630446269459,-0.146227808723351,
-0.837681688765196));
#78473=CARTESIAN_POINT('Ctrl Pts',(0.0638237060851255,-0.141869906694057,
-0.836927208658677));
#78474=CARTESIAN_POINT('Ctrl Pts',(0.065801645290444,-0.140963394445596,
-0.836776261977263));
#78475=CARTESIAN_POINT('Ctrl Pts',(0.0690114468421759,-0.13941002868216,
-0.836526568133483));
#78476=CARTESIAN_POINT('Ctrl Pts',(0.0702548354752405,-0.13878758504794,
-0.836428652226879));
#78477=CARTESIAN_POINT('Ctrl Pts',(0.072489241070864,-0.137631315881724,
-0.836250429825517));
#78478=CARTESIAN_POINT('Ctrl Pts',(0.0734831363574897,-0.137103237497877,
-0.836170328421121));
#78479=CARTESIAN_POINT('Ctrl Pts',(0.0756174819075255,-0.135939338152933,
-0.835996471681533));
#78480=CARTESIAN_POINT('Ctrl Pts',(0.0767558242897936,-0.135299853929816,
-0.835902591035302));
#78481=CARTESIAN_POINT('Ctrl Pts',(0.0799261440184571,-0.133465984963104,
-0.83563778955541));
#78482=CARTESIAN_POINT('Ctrl Pts',(0.081939142236088,-0.132239681979833,
-0.835465738952083));
#78483=CARTESIAN_POINT('Ctrl Pts',(0.0906653730638681,-0.12664798013438,
-0.834702041913793));
#78484=CARTESIAN_POINT('Ctrl Pts',(0.0970626604596442,-0.121814305874785,
-0.834093700797114));
#78485=CARTESIAN_POINT('Ctrl Pts',(0.109690555364888,-0.110644374858337,
-0.832793313323083));
#78486=CARTESIAN_POINT('Ctrl Pts',(0.11580949203002,-0.104222662220506,
-0.832101436562797));
#78487=CARTESIAN_POINT('Ctrl Pts',(0.123303788589299,-0.0948775090641157,
-0.831191149830478));
#78488=CARTESIAN_POINT('Ctrl Pts',(0.125184911314852,-0.0923813142306498,
-0.830956398470307));
#78489=CARTESIAN_POINT('Ctrl Pts',(0.12759024427023,-0.0889809725565789,
-0.830649248111102));
#78490=CARTESIAN_POINT('Ctrl Pts',(0.128182283630052,-0.0881259679657376,
-0.830573043999079));
#78491=CARTESIAN_POINT('Ctrl Pts',(0.129104033436509,-0.0867658613867691,
-0.830453513456204));
#78492=CARTESIAN_POINT('Ctrl Pts',(0.129439444153673,-0.0862646885010198,
-0.830409826392481));
#78493=CARTESIAN_POINT('Ctrl Pts',(0.130137006505214,-0.0852091571824253,
-0.830318584407875));
#78494=CARTESIAN_POINT('Ctrl Pts',(0.130498548045944,-0.0846544146276616,
-0.830271073253424));
#78495=CARTESIAN_POINT('Ctrl Pts',(0.131400067594264,-0.0832516391280894,
-0.830151995174289));
#78496=CARTESIAN_POINT('Ctrl Pts',(0.131935399757691,-0.0824006287165008,
-0.83008072386194));
#78497=CARTESIAN_POINT('Ctrl Pts',(0.134077117150483,-0.0789215798138939,
-0.829793010548335));
#78498=CARTESIAN_POINT('Ctrl Pts',(0.135613648893791,-0.0762511014932603,
-0.829580549374698));
#78499=CARTESIAN_POINT('Ctrl Pts',(0.139763116065837,-0.0685166148901526,
-0.8289835013209));
#78500=CARTESIAN_POINT('Ctrl Pts',(0.142178651599012,-0.063352155181564,
-0.828606352145697));
#78501=CARTESIAN_POINT('Ctrl Pts',(0.148540432715208,-0.0475419960390593,
-0.827482470307737));
#78502=CARTESIAN_POINT('Ctrl Pts',(0.151610870149014,-0.0365870505274984,
-0.826740838813642));
#78503=CARTESIAN_POINT('Ctrl Pts',(0.153837466405655,-0.0231322715663798,
-0.825801211634254));
#78504=CARTESIAN_POINT('Ctrl Pts',(0.15416195283639,-0.0208604751253779,
-0.825641729459637));
#78505=CARTESIAN_POINT('Ctrl Pts',(0.154592091199917,-0.01728565339994,
-0.825389025731491));
#78506=CARTESIAN_POINT('Ctrl Pts',(0.154731781255011,-0.0159869997163653,
-0.825296865463052));
#78507=CARTESIAN_POINT('Ctrl Pts',(0.154961357265479,-0.0135663856183572,
-0.825124339333427));
#78508=CARTESIAN_POINT('Ctrl Pts',(0.155055452413844,-0.0124449033596596,
-0.825044110568599));
#78509=CARTESIAN_POINT('Ctrl Pts',(0.155238532158182,-0.0099364073161369,
-0.824863946016108));
#78510=CARTESIAN_POINT('Ctrl Pts',(0.155321111762918,-0.00854903891208235,
-0.82476381742091));
#78511=CARTESIAN_POINT('Ctrl Pts',(0.155513415667156,-0.00437615359388857,
-0.824461100002319));
#78512=CARTESIAN_POINT('Ctrl Pts',(0.155566857721069,-0.00158874614488409,
-0.824256801477925));
#78513=CARTESIAN_POINT('Ctrl Pts',(0.155496884209671,0.00749315129874472,
-0.823583938968423));
#78514=CARTESIAN_POINT('Ctrl Pts',(0.155066333305595,0.01377836360493,-0.823106678952239));
#78515=CARTESIAN_POINT('Ctrl Pts',(0.152919902704755,0.0303172211991329,
-0.821824647418094));
#78516=CARTESIAN_POINT('Ctrl Pts',(0.15055571301723,0.0404550463541575,
-0.821010353685325));
#78517=CARTESIAN_POINT('Ctrl Pts',(0.14632315326996,0.0528458036152662,
-0.820019322710012));
#78518=CARTESIAN_POINT('Ctrl Pts',(0.145380374323205,0.055386759401077,
-0.819816472250009));
#78519=CARTESIAN_POINT('Ctrl Pts',(0.144003986368269,0.0588186179126531,
-0.819544167215913));
#78520=CARTESIAN_POINT('Ctrl Pts',(0.143627618025319,0.0597317786338072,
-0.819471876184374));
#78521=CARTESIAN_POINT('Ctrl Pts',(0.143011233789928,0.0611877570533963,
-0.81935694636979));
#78522=CARTESIAN_POINT('Ctrl Pts',(0.142776772713994,0.061732874618455,
-0.819313992284588));
#78523=CARTESIAN_POINT('Ctrl Pts',(0.142269406538304,0.0628941375601393,
-0.819222669364491));
#78524=CARTESIAN_POINT('Ctrl Pts',(0.141995603917309,0.0635098818342275,
-0.819174356815171));
#78525=CARTESIAN_POINT('Ctrl Pts',(0.141280289800332,0.0650907718646905,
-0.819050552115307));
#78526=CARTESIAN_POINT('Ctrl Pts',(0.140832877692933,0.0660532330223818,
-0.81897540577497));
#78527=CARTESIAN_POINT('Ctrl Pts',(0.138811969690908,0.070286656294552,
-0.81864554852775));
#78528=CARTESIAN_POINT('Ctrl Pts',(0.13713398627255,0.0735068137515336,
-0.818396434174411));
#78529=CARTESIAN_POINT('Ctrl Pts',(0.13156671691883,0.0833352189627264,
-0.817632567730148));
#78530=CARTESIAN_POINT('Ctrl Pts',(0.127300638355638,0.0897169034577439,
-0.817131026333492));
#78531=CARTESIAN_POINT('Ctrl Pts',(0.116868924342838,0.103070635427417,
-0.816013980553107));
#78532=CARTESIAN_POINT('Ctrl Pts',(0.110514645519303,0.109856189988094,
-0.815398286312547));
#78533=CARTESIAN_POINT('Ctrl Pts',(0.103178831595365,0.116405503386327,
-0.814717693594607));
#78534=CARTESIAN_POINT('Ctrl Pts',(0.102761515737733,0.116774069697995,
-0.814679076198737));
#78535=CARTESIAN_POINT('Ctrl Pts',(0.102342242814364,0.117140376624483,
-0.814640372754811));
#78536=CARTESIAN_POINT('Origin',(0.,0.,-1.10400562256037));
#78537=CARTESIAN_POINT('',(0.10234224283772,0.117140376604078,-0.730690163752328));
#78538=CARTESIAN_POINT('',(0.102342226135012,0.11714039119676,-0.744524458909986));
#78539=CARTESIAN_POINT('',(0.10234224283772,0.117140376604078,-1.10400562256037));
#78540=CARTESIAN_POINT('',(-0.155549988636594,5.94571726719256E-5,-0.775194377434571));
#78541=CARTESIAN_POINT('Ctrl Pts',(-0.155549988636594,5.94571726719256E-5,
-0.775194377434571));
#78542=CARTESIAN_POINT('Ctrl Pts',(-0.15555386600914,-0.0100844031602943,
-0.774463862461081));
#78543=CARTESIAN_POINT('Ctrl Pts',(-0.154561163212359,-0.0202683545329286,
-0.773733347487591));
#78544=CARTESIAN_POINT('Ctrl Pts',(-0.152574549297427,-0.0302788607230699,
-0.7730028325141));
#78545=CARTESIAN_POINT('Ctrl Pts',(-0.150590323408965,-0.0402773336975079,
-0.772273195662463));
#78546=CARTESIAN_POINT('Ctrl Pts',(-0.147614646911284,-0.0501018361313886,
-0.771543558810827));
#78547=CARTESIAN_POINT('Ctrl Pts',(-0.143701919267921,-0.0595446126758421,
-0.77081392195919));
#78548=CARTESIAN_POINT('Ctrl Pts',(-0.139792442521125,-0.0689795436729801,
-0.7700848913276));
#78549=CARTESIAN_POINT('Ctrl Pts',(-0.134947811940159,-0.0780325003649032,
-0.769355860696011));
#78550=CARTESIAN_POINT('Ctrl Pts',(-0.129270866042447,-0.0865150027026283,
-0.768626830064421));
#78551=CARTESIAN_POINT('Ctrl Pts',(-0.123580591224642,-0.0950174211357128,
-0.767896087739395));
#78552=CARTESIAN_POINT('Ctrl Pts',(-0.117054652334967,-0.102945937307198,
-0.767165345414368));
#78553=CARTESIAN_POINT('Ctrl Pts',(-0.109838640819849,-0.110142069541335,
-0.766434603089342));
#78554=CARTESIAN_POINT('Ctrl Pts',(-0.104564595969931,-0.115401585004865,
-0.765900517495403));
#78555=CARTESIAN_POINT('Ctrl Pts',(-0.0989228665778733,-0.120270514573088,
-0.765366431901464));
#78556=CARTESIAN_POINT('Ctrl Pts',(-0.0929813870164388,-0.124700698348082,
-0.764832346307525));
#78557=CARTESIAN_POINT('Ctrl Pts',(-0.0847762750881243,-0.130818728943149,
-0.764094780515662));
#78558=CARTESIAN_POINT('Ctrl Pts',(-0.0759342485538406,-0.136146198466278,
-0.763357214723798));
#78559=CARTESIAN_POINT('Ctrl Pts',(-0.0666312496326838,-0.140556319930436,
-0.762619648931935));
#78560=CARTESIAN_POINT('Ctrl Pts',(-0.0573061358502367,-0.144976925027374,
-0.761880329816727));
#78561=CARTESIAN_POINT('Ctrl Pts',(-0.0475186300913685,-0.148475284583797,
-0.76114101070152));
#78562=CARTESIAN_POINT('Ctrl Pts',(-0.0374732079475383,-0.150968742414185,
-0.760401691586313));
#78563=CARTESIAN_POINT('Ctrl Pts',(-0.0274744847389166,-0.153450608713227,
-0.759665809401377));
#78564=CARTESIAN_POINT('Ctrl Pts',(-0.0172211422329046,-0.154936667906122,
-0.758929927216442));
#78565=CARTESIAN_POINT('Ctrl Pts',(-0.00692912148693312,-0.155395591235464,
-0.758194045031506));
#78566=CARTESIAN_POINT('Ctrl Pts',(0.0034350024266058,-0.15585772965993,
-0.757453007451163));
#78567=CARTESIAN_POINT('Ctrl Pts',(0.0138374003939213,-0.155278229143345,
-0.756711969870819));
#78568=CARTESIAN_POINT('Ctrl Pts',(0.0240570027497603,-0.153678440643761,
-0.755970932290476));
#78569=CARTESIAN_POINT('Ctrl Pts',(0.0342766051055992,-0.152078652144177,
-0.755229894710133));
#78570=CARTESIAN_POINT('Ctrl Pts',(0.0443124994057009,-0.149458849024487,
-0.754488857129789));
#78571=CARTESIAN_POINT('Ctrl Pts',(0.0539571410731116,-0.145891841537546,
-0.753747819549446));
#78572=CARTESIAN_POINT('Ctrl Pts',(0.0635565972037738,-0.142341545625118,
-0.753010253760173));
#78573=CARTESIAN_POINT('Ctrl Pts',(0.0728398182548613,-0.13782655163654,
-0.7522726879709));
#78574=CARTESIAN_POINT('Ctrl Pts',(0.0816046551225161,-0.132425385641633,
-0.751535122181627));
#78575=CARTESIAN_POINT('Ctrl Pts',(0.0903903275843545,-0.12701138010339,
-0.750795803065772));
#78576=CARTESIAN_POINT('Ctrl Pts',(0.0986542812351905,-0.120707344980565,
-0.750056483949917));
#78577=CARTESIAN_POINT('Ctrl Pts',(0.106215842921805,-0.113639769501748,
-0.749317164834062));
#78578=CARTESIAN_POINT('Ctrl Pts',(0.11374225254917,-0.106605049647507,
-0.748581282652327));
#78579=CARTESIAN_POINT('Ctrl Pts',(0.120572102713786,-0.0988145072758199,
-0.747845400470592));
#78580=CARTESIAN_POINT('Ctrl Pts',(0.126561526551945,-0.0904321983413054,
-0.747109518288857));
#78581=CARTESIAN_POINT('Ctrl Pts',(0.132592910752094,-0.0819911651076437,
-0.746368480705942));
#78582=CARTESIAN_POINT('Ctrl Pts',(0.137771484362896,-0.0729508066652424,
-0.745627443123026));
#78583=CARTESIAN_POINT('Ctrl Pts',(0.141994771738795,-0.0635081671822421,
-0.744886405540111));
#78584=CARTESIAN_POINT('Ctrl Pts',(0.146218059114693,-0.0540655276992418,
-0.744145367957196));
#78585=CARTESIAN_POINT('Ctrl Pts',(0.149485792662233,-0.0442215213286015,
-0.74340433037428));
#78586=CARTESIAN_POINT('Ctrl Pts',(0.151746022211242,-0.0341898704745336,
-0.742663292791365));
#78587=CARTESIAN_POINT('Ctrl Pts',(0.153995662520478,-0.0242052181902564,
-0.741925726990618));
#78588=CARTESIAN_POINT('Ctrl Pts',(0.15526397707335,-0.01396047585451,-0.741188161189871));
#78589=CARTESIAN_POINT('Ctrl Pts',(0.155506747828537,-0.00366795307928527,
-0.740450595389125));
#78590=CARTESIAN_POINT('Ctrl Pts',(0.155750095688758,0.00664903667386102,
-0.739711276276138));
#78591=CARTESIAN_POINT('Ctrl Pts',(0.154962848460286,0.0170131106572213,
-0.738971957163151));
#78592=CARTESIAN_POINT('Ctrl Pts',(0.153152710900332,0.0272038534748175,
-0.738232638050165));
#78593=CARTESIAN_POINT('Ctrl Pts',(0.151350988240431,0.0373472219468521,
-0.737496755856328));
#78594=CARTESIAN_POINT('Ctrl Pts',(0.148536024465825,0.0473179483910715,
-0.73676087366249));
#78595=CARTESIAN_POINT('Ctrl Pts',(0.144767075467698,0.0569060309679909,
-0.736024991468653));
#78596=CARTESIAN_POINT('Ctrl Pts',(0.140971722298303,0.0665612848901873,
-0.735283953896092));
#78597=CARTESIAN_POINT('Ctrl Pts',(0.136209300468937,0.0758276239839394,
-0.734542916323531));
#78598=CARTESIAN_POINT('Ctrl Pts',(0.130589273582521,0.0845117987336059,
-0.733801878750969));
#78599=CARTESIAN_POINT('Ctrl Pts',(0.124969246696105,0.0931959734832724,
-0.733060841178408));
#78600=CARTESIAN_POINT('Ctrl Pts',(0.118492235761233,0.101297261649368,
-0.732319803605846));
#78601=CARTESIAN_POINT('Ctrl Pts',(0.11130920650138,0.108655708768721,-0.731578766033285));
#78602=CARTESIAN_POINT('Ctrl Pts',(0.108438071747974,0.111596959944399,
-0.731282565272966));
#78603=CARTESIAN_POINT('Ctrl Pts',(0.105446013534655,0.114428699694826,
-0.730986364512647));
#78604=CARTESIAN_POINT('Ctrl Pts',(0.10234224283772,0.117140376604078,-0.730690163752328));
#78605=CARTESIAN_POINT('Ctrl Pts',(0.10234224283772,0.117140376604078,-0.800700826369366));
#78606=CARTESIAN_POINT('Ctrl Pts',(0.0945830959428436,0.123919324382374,
-0.79996324687108));
#78607=CARTESIAN_POINT('Ctrl Pts',(0.0861632602065998,0.129910446345868,
-0.799225667372795));
#78608=CARTESIAN_POINT('Ctrl Pts',(0.0772687420922595,0.135001274051321,
-0.79848808787451));
#78609=CARTESIAN_POINT('Ctrl Pts',(0.0756521792171102,0.135926522948071,
-0.798354034110262));
#78610=CARTESIAN_POINT('Ctrl Pts',(0.0740199996624193,0.136822156691536,
-0.798219980346014));
#78611=CARTESIAN_POINT('Ctrl Pts',(0.072373396601727,0.137687668163598,
-0.798085926581766));
#78612=CARTESIAN_POINT('Ctrl Pts',(0.0633137622828552,0.142449725044736,
-0.797348360794268));
#78613=CARTESIAN_POINT('Ctrl Pts',(0.0537484429186352,0.146331481039621,
-0.796610795006771));
#78614=CARTESIAN_POINT('Ctrl Pts',(0.0438710170354423,0.149235171337979,
-0.795873229219274));
#78615=CARTESIAN_POINT('Ctrl Pts',(0.0339701107040233,0.152145764239355,
-0.795133910102975));
#78616=CARTESIAN_POINT('Ctrl Pts',(0.0237564602461081,0.154073232376168,
-0.794394590986676));
#78617=CARTESIAN_POINT('Ctrl Pts',(0.0134449381321283,0.154967855178496,
-0.793655271870377));
#78618=CARTESIAN_POINT('Ctrl Pts',(0.00318135204152644,0.155858319074011,
-0.792919389687835));
#78619=CARTESIAN_POINT('Ctrl Pts',(-0.00717826886897367,0.155725435483212,
-0.792183507505293));
#78620=CARTESIAN_POINT('Ctrl Pts',(-0.017415740338501,0.154571971872206,
-0.791447625322752));
#78621=CARTESIAN_POINT('Ctrl Pts',(-0.0277249328908003,0.153410427392855,
-0.790706587739574));
#78622=CARTESIAN_POINT('Ctrl Pts',(-0.0379093125922557,0.151214040730291,
-0.789965550156396));
#78623=CARTESIAN_POINT('Ctrl Pts',(-0.0477538536585732,0.148038413801133,
-0.789224512573219));
#78624=CARTESIAN_POINT('Ctrl Pts',(-0.0575983947248908,0.144862786871975,
-0.788483474990041));
#78625=CARTESIAN_POINT('Ctrl Pts',(-0.0671022385762959,0.140708332135486,
-0.787742437406863));
#78626=CARTESIAN_POINT('Ctrl Pts',(-0.0760717523565394,0.135679368340973,
-0.787001399823686));
#78627=CARTESIAN_POINT('Ctrl Pts',(-0.0849992430142917,0.130673965774717,
-0.786263834080107));
#78628=CARTESIAN_POINT('Ctrl Pts',(-0.0934637703868424,0.124765063504695,
-0.785526268336529));
#78629=CARTESIAN_POINT('Ctrl Pts',(-0.101277923274961,0.118061783643613,
-0.784788702592951));
#78630=CARTESIAN_POINT('Ctrl Pts',(-0.109110652416689,0.111342568360163,
-0.784049383465672));
#78631=CARTESIAN_POINT('Ctrl Pts',(-0.116289110998618,0.103825685675319,
-0.783310064338393));
#78632=CARTESIAN_POINT('Ctrl Pts',(-0.122654588270765,0.0956642800429139,
-0.782570745211114));
#78633=CARTESIAN_POINT('Ctrl Pts',(-0.128990473306033,0.0875408156737357,
-0.781834863077765));
#78634=CARTESIAN_POINT('Ctrl Pts',(-0.134520343035544,0.0787795411156073,
-0.781098980944416));
#78635=CARTESIAN_POINT('Ctrl Pts',(-0.139127706543723,0.0695649608055928,
-0.780363098811067));
#78636=CARTESIAN_POINT('Ctrl Pts',(-0.143767348618724,0.0602858243897395,
-0.779622061186824));
#78637=CARTESIAN_POINT('Ctrl Pts',(-0.147471071797916,0.0505478495391549,
-0.77888102356258));
#78638=CARTESIAN_POINT('Ctrl Pts',(-0.150168418866794,0.0405616626267601,
-0.778139985938336));
#78639=CARTESIAN_POINT('Ctrl Pts',(-0.152865765935671,0.0305754757143654,
-0.777398948314093));
#78640=CARTESIAN_POINT('Ctrl Pts',(-0.15455661529663,0.0203420214609023,
-0.776657910689849));
#78641=CARTESIAN_POINT('Ctrl Pts',(-0.155223019478323,0.0100805120917568,
-0.775916873065605));
#78642=CARTESIAN_POINT('Ctrl Pts',(-0.155439596023901,0.00674559566620943,
-0.77567604119028));
#78643=CARTESIAN_POINT('Ctrl Pts',(-0.155548710365706,0.00340362539228194,
-0.775435209314955));
#78644=CARTESIAN_POINT('Ctrl Pts',(-0.155549988636567,5.94572429166567E-5,
-0.77519437743963));
#78645=CARTESIAN_POINT('',(-0.155549929833988,-0.000141245247018929,-0.789026374106901));
#78646=CARTESIAN_POINT('Ctrl Pts',(0.102342242814364,0.117140376624483,
-0.814640372754811));
#78647=CARTESIAN_POINT('Ctrl Pts',(0.101247987115879,0.118096396961982,
-0.814539361070758));
#78648=CARTESIAN_POINT('Ctrl Pts',(0.100140400890045,0.119037027434954,
-0.814437762401209));
#78649=CARTESIAN_POINT('Ctrl Pts',(0.0980683028869122,0.120747392027465,
-0.81424874066824));
#78650=CARTESIAN_POINT('Ctrl Pts',(0.097107512032578,0.121521420591653,
-0.814161500428143));
#78651=CARTESIAN_POINT('Ctrl Pts',(0.0952423368108456,0.122987791192865,
-0.81399284801475));
#78652=CARTESIAN_POINT('Ctrl Pts',(0.0943393533588697,0.123681792456681,
-0.813911508780979));
#78653=CARTESIAN_POINT('Ctrl Pts',(0.0922173013781256,0.125275967722571,
-0.813721023289307));
#78654=CARTESIAN_POINT('Ctrl Pts',(0.0909925561961174,0.126168352526021,
-0.813611585108866));
#78655=CARTESIAN_POINT('Ctrl Pts',(0.0868837031025962,0.129071236516884,
-0.813245951189801));
#78656=CARTESIAN_POINT('Ctrl Pts',(0.0839446808462585,0.131001713317316,
-0.812986820087241));
#78657=CARTESIAN_POINT('Ctrl Pts',(0.0765225369886381,0.135524537521265,
-0.812337797865434));
#78658=CARTESIAN_POINT('Ctrl Pts',(0.0719707794888592,0.137995640176101,
-0.811944305583081));
#78659=CARTESIAN_POINT('Ctrl Pts',(0.0580641705603296,0.144670006263189,
-0.810758696607579));
#78660=CARTESIAN_POINT('Ctrl Pts',(0.0484080750056315,0.148180695886636,
-0.809955167656746));
#78661=CARTESIAN_POINT('Ctrl Pts',(0.0357238872036029,0.151418885865566,
-0.808963026583044));
#78662=CARTESIAN_POINT('Ctrl Pts',(0.0329519874985958,0.152046190829675,
-0.80875007282081));
#78663=CARTESIAN_POINT('Ctrl Pts',(0.0291782851967918,0.152792147350082,
-0.808466653849693));
#78664=CARTESIAN_POINT('Ctrl Pts',(0.028190416146552,0.15297749245713,-0.808393059295612));
#78665=CARTESIAN_POINT('Ctrl Pts',(0.0266134420730029,0.153257570955974,
-0.80827660097801));
#78666=CARTESIAN_POINT('Ctrl Pts',(0.0260254897585766,0.153358508956619,
-0.808233407028251));
#78667=CARTESIAN_POINT('Ctrl Pts',(0.0247764292561043,0.153565553883757,
-0.808142144143772));
#78668=CARTESIAN_POINT('Ctrl Pts',(0.0241151862038325,0.153670779979575,
-0.808094127178692));
#78669=CARTESIAN_POINT('Ctrl Pts',(0.0224240763594421,0.153928708106129,
-0.807972035005134));
#78670=CARTESIAN_POINT('Ctrl Pts',(0.0213932958912589,0.154075349832642,
-0.807898287230063));
#78671=CARTESIAN_POINT('Ctrl Pts',(0.0169715942593336,0.154659162060053,
-0.807584500646974));
#78672=CARTESIAN_POINT('Ctrl Pts',(0.0135679637438788,0.154994857779847,
-0.807349407302497));
#78673=CARTESIAN_POINT('Ctrl Pts',(0.00332708986492769,0.155664906549473,
-0.806653897580513));
#78674=CARTESIAN_POINT('Ctrl Pts',(-0.00352409285299623,0.155660613162722,
-0.806204126969112));
#78675=CARTESIAN_POINT('Ctrl Pts',(-0.0199791529533464,0.154562960106711,
-0.805117866157702));
#78676=CARTESIAN_POINT('Ctrl Pts',(-0.0295234485217771,0.153026834034583,
-0.804481723355181));
#78677=CARTESIAN_POINT('Ctrl Pts',(-0.040956746243398,0.150076717431665,
-0.803669014212957));
#78678=CARTESIAN_POINT('Ctrl Pts',(-0.0430384737204866,0.149493027210443,
-0.803518998861588));
#78679=CARTESIAN_POINT('Ctrl Pts',(-0.0464341781460082,0.148464109851312,
-0.803270523055676));
#78680=CARTESIAN_POINT('Ctrl Pts',(-0.0477556039096431,0.148044340958285,
-0.80317287967734));
#78681=CARTESIAN_POINT('Ctrl Pts',(-0.0501389954308398,0.147251994300334,
-0.802994943111323));
#78682=CARTESIAN_POINT('Ctrl Pts',(-0.0512028761965604,0.146885445284617,
-0.80291485185034));
#78683=CARTESIAN_POINT('Ctrl Pts',(-0.0534953528867185,0.1460676644918,
-0.802740775802747));
#78684=CARTESIAN_POINT('Ctrl Pts',(-0.0547224094469159,0.145612407101328,
-0.802646663127608));
#78685=CARTESIAN_POINT('Ctrl Pts',(-0.0581571172396773,0.144288530681654,
-0.802380499465904));
#78686=CARTESIAN_POINT('Ctrl Pts',(-0.0603507658864985,0.143384846785658,
-0.802207299846554));
#78687=CARTESIAN_POINT('Ctrl Pts',(-0.0699657033930099,0.139164199672636,
-0.801433390857135));
#78688=CARTESIAN_POINT('Ctrl Pts',(-0.0771399352777933,0.135319132107625,
-0.800815449785842));
#78689=CARTESIAN_POINT('Ctrl Pts',(-0.0916372093746799,0.126020546836185,
-0.799486427765102));
#78690=CARTESIAN_POINT('Ctrl Pts',(-0.0988489298787561,0.120446894595726,
-0.798775394045735));
#78691=CARTESIAN_POINT('Ctrl Pts',(-0.107600153025353,0.112365172782629,
-0.797872836036262));
#78692=CARTESIAN_POINT('Ctrl Pts',(-0.109615917275998,0.110399629145226,
-0.797661919819693));
#78693=CARTESIAN_POINT('Ctrl Pts',(-0.112275236374755,0.107661864106398,
-0.797380736848244));
#78694=CARTESIAN_POINT('Ctrl Pts',(-0.112966170103791,0.106936664613663,
-0.797307400789476));
#78695=CARTESIAN_POINT('Ctrl Pts',(-0.114056935431468,0.1057694335537,-0.797191246418278));
#78696=CARTESIAN_POINT('Ctrl Pts',(-0.114461300448228,0.105331706177061,
-0.797148100879334));
#78697=CARTESIAN_POINT('Ctrl Pts',(-0.115315185736076,0.104396646546545,
-0.797056830079302));
#78698=CARTESIAN_POINT('Ctrl Pts',(-0.115764027862494,0.103898709158497,
-0.797008757626578));
#78699=CARTESIAN_POINT('Ctrl Pts',(-0.116812393927484,0.10272044267184,
-0.796896201714844));
#78700=CARTESIAN_POINT('Ctrl Pts',(-0.117409224795774,0.102037732011308,
-0.796831910585526));
#78701=CARTESIAN_POINT('Ctrl Pts',(-0.119320645519724,0.0998122936287535,
-0.79662516157429));
#78702=CARTESIAN_POINT('Ctrl Pts',(-0.120611122538167,0.0982490126800226,
-0.796484252002993));
#78703=CARTESIAN_POINT('Ctrl Pts',(-0.122382151175805,0.0960160863864426,
-0.796288231891698));
#78704=CARTESIAN_POINT('Ctrl Pts',(-0.122888437734998,0.0953672464496936,
-0.796231878543083));
#78705=CARTESIAN_POINT('Ctrl Pts',(-0.126446090409272,0.0907325006148665,
-0.795833370166034));
#78706=CARTESIAN_POINT('Ctrl Pts',(-0.129308308145013,0.0866046719690133,
-0.795499378150036));
#78707=CARTESIAN_POINT('Ctrl Pts',(-0.137060632348669,0.0741808571452341,
-0.794531469747891));
#78708=CARTESIAN_POINT('Ctrl Pts',(-0.141386272580957,0.0655616365079737,
-0.793904277177543));
#78709=CARTESIAN_POINT('Ctrl Pts',(-0.146358028189157,0.0528342593432668,
-0.792980698981075));
#78710=CARTESIAN_POINT('Ctrl Pts',(-0.147681003810113,0.049014773027456,
-0.792704063434883));
#78711=CARTESIAN_POINT('Ctrl Pts',(-0.149328838784549,0.0435818773564268,
-0.792308650382566));
#78712=CARTESIAN_POINT('Ctrl Pts',(-0.149779191414869,0.0420080419823773,
-0.792193890879958));
#78713=CARTESIAN_POINT('Ctrl Pts',(-0.150502804418005,0.0393195215335305,
-0.791997333286324));
#78714=CARTESIAN_POINT('Ctrl Pts',(-0.150788725864499,0.0382083621246268,
-0.791915947757818));
#78715=CARTESIAN_POINT('Ctrl Pts',(-0.151346192988089,0.0359381325070211,
-0.791749312714464));
#78716=CARTESIAN_POINT('Ctrl Pts',(-0.151616776667209,0.0347789072338163,
-0.791664038493042));
#78717=CARTESIAN_POINT('Ctrl Pts',(-0.152134325830938,0.0324407173661172,
-0.791491615906685));
#78718=CARTESIAN_POINT('Ctrl Pts',(-0.152380954422049,0.0312617628735881,
-0.791404463267835));
#78719=CARTESIAN_POINT('Ctrl Pts',(-0.15294585172281,0.0283957093218414,
-0.791192031437218));
#78720=CARTESIAN_POINT('Ctrl Pts',(-0.153249921783962,0.0267060088715932,
-0.791066319562526));
#78721=CARTESIAN_POINT('Ctrl Pts',(-0.154880940457497,0.0166945391990566,
-0.790318513571554));
#78722=CARTESIAN_POINT('Ctrl Pts',(-0.155557588103049,0.00828257885722836,
-0.789676994178376));
#78723=CARTESIAN_POINT('Ctrl Pts',(-0.155549935820354,-0.000141302101484485,
-0.789026380191115));
#78724=CARTESIAN_POINT('Ctrl Pts',(-0.155549935871255,-0.000141246056687843,
-0.789026384519706));
#78725=CARTESIAN_POINT('Ctrl Pts',(-0.155540361813676,-0.0106848610596033,
-0.788212054034337));
#78726=CARTESIAN_POINT('Ctrl Pts',(-0.15445882295033,-0.0212010662537019,
-0.787386500385918));
#78727=CARTESIAN_POINT('Ctrl Pts',(-0.152093774235884,-0.0326273994928223,
-0.786516650549246));
#78728=CARTESIAN_POINT('Ctrl Pts',(-0.151854274310337,-0.033724514967364,
-0.786433438329619));
#78729=CARTESIAN_POINT('Ctrl Pts',(-0.151387612508525,-0.0357563748508333,
-0.786280015877868));
#78730=CARTESIAN_POINT('Ctrl Pts',(-0.151163621620343,-0.0366917863787319,
-0.786209656527296));
#78731=CARTESIAN_POINT('Ctrl Pts',(-0.150772843442499,-0.0382593713036209,
-0.786092271465715));
#78732=CARTESIAN_POINT('Ctrl Pts',(-0.15061072380648,-0.0388926696503636,
-0.786044993520268));
#78733=CARTESIAN_POINT('Ctrl Pts',(-0.150266476782737,-0.0402029838497188,
-0.785947498336013));
#78734=CARTESIAN_POINT('Ctrl Pts',(-0.150083757949649,-0.0408798190591607,
-0.785897314452474));
#78735=CARTESIAN_POINT('Ctrl Pts',(-0.149579387694897,-0.0426991564627536,
-0.78576283827918));
#78736=CARTESIAN_POINT('Ctrl Pts',(-0.149249217960623,-0.043839278603837,
-0.785679012369898));
#78737=CARTESIAN_POINT('Ctrl Pts',(-0.147493071270416,-0.0496535661741509,
-0.785253278113192));
#78738=CARTESIAN_POINT('Ctrl Pts',(-0.145860302366329,-0.0542629286958753,
-0.784921564565051));
#78739=CARTESIAN_POINT('Ctrl Pts',(-0.140804862483097,-0.0666471977348302,
-0.784026898361794));
#78740=CARTESIAN_POINT('Ctrl Pts',(-0.136958713094505,-0.0742305790355904,
-0.78347456109652));
#78741=CARTESIAN_POINT('Ctrl Pts',(-0.128887350463018,-0.0873600570599175,
-0.782452563088397));
#78742=CARTESIAN_POINT('Ctrl Pts',(-0.124872549919944,-0.0930083740591326,
-0.781987736428872));
#78743=CARTESIAN_POINT('Ctrl Pts',(-0.119239431260928,-0.0999084792263256,
-0.781371409933041));
#78744=CARTESIAN_POINT('Ctrl Pts',(-0.117954269111278,-0.101422561448616,
-0.781232939892915));
#78745=CARTESIAN_POINT('Ctrl Pts',(-0.116592486349677,-0.102966013317513,
-0.781088197856267));
#78746=CARTESIAN_POINT('Ctrl Pts',(-0.116544412000777,-0.103020424203474,
-0.781083090606553));
#78747=CARTESIAN_POINT('Ctrl Pts',(-0.116448794084408,-0.103128492647877,
-0.781072937459522));
#78748=CARTESIAN_POINT('Ctrl Pts',(-0.116401251481458,-0.103182151039102,
-0.781067891602064));
#78749=CARTESIAN_POINT('Ctrl Pts',(-0.116306096630273,-0.103289396964021,
-0.781057797343336));
#78750=CARTESIAN_POINT('Ctrl Pts',(-0.116258484400569,-0.103342984490548,
-0.781052748943587));
#78751=CARTESIAN_POINT('Ctrl Pts',(-0.116162552829664,-0.103450805197948,
-0.78104258202524));
#78752=CARTESIAN_POINT('Ctrl Pts',(-0.116114232511959,-0.103505037481928,
-0.781037463467647));
#78753=CARTESIAN_POINT('Ctrl Pts',(-0.116016173118801,-0.103614939308742,
-0.781027081064067));
#78754=CARTESIAN_POINT('Ctrl Pts',(-0.115966431922367,-0.103670606925235,
-0.781021817132265));
#78755=CARTESIAN_POINT('Ctrl Pts',(-0.115864695375924,-0.103784300045495,
-0.781011056018143));
#78756=CARTESIAN_POINT('Ctrl Pts',(-0.115812696472497,-0.103842322326781,
-0.781005558691186));
#78757=CARTESIAN_POINT('Ctrl Pts',(-0.115705414504048,-0.103961850664916,
-0.78099422262899));
#78758=CARTESIAN_POINT('Ctrl Pts',(-0.115650125949224,-0.104023351739451,
-0.780988383669284));
#78759=CARTESIAN_POINT('Ctrl Pts',(-0.115534932447873,-0.10415128365,-0.780976224775889));
#78760=CARTESIAN_POINT('Ctrl Pts',(-0.115475019207543,-0.104217706943855,
-0.780969904501767));
#78761=CARTESIAN_POINT('Ctrl Pts',(-0.114649175765539,-0.105131698443217,
-0.780882836392923));
#78762=CARTESIAN_POINT('Ctrl Pts',(-0.113874007494642,-0.105970834725577,
-0.780801707822105));
#78763=CARTESIAN_POINT('Ctrl Pts',(-0.112249175796799,-0.107691334773083,
-0.780632823909134));
#78764=CARTESIAN_POINT('Ctrl Pts',(-0.111398212217701,-0.108571355381265,
-0.780545016185137));
#78765=CARTESIAN_POINT('Ctrl Pts',(-0.109155225321393,-0.110836799659655,
-0.780315155031285));
#78766=CARTESIAN_POINT('Ctrl Pts',(-0.107747233539381,-0.11220602651901,
-0.780172409007194));
#78767=CARTESIAN_POINT('Ctrl Pts',(-0.100563045108552,-0.118932493504905,
-0.779451315632692));
#78768=CARTESIAN_POINT('Ctrl Pts',(-0.0944125420257412,-0.123871304973134,
-0.778856016829919));
#78769=CARTESIAN_POINT('Ctrl Pts',(-0.0820500672480588,-0.132340997422237,
-0.777703411444543));
#78770=CARTESIAN_POINT('Ctrl Pts',(-0.0759160979816154,-0.135952549266159,
-0.777149526854872));
#78771=CARTESIAN_POINT('Ctrl Pts',(-0.0646969383402677,-0.141561403034217,
-0.776182943557273));
#78772=CARTESIAN_POINT('Ctrl Pts',(-0.0597124762297606,-0.143735026533935,
-0.77576852311152));
#78773=CARTESIAN_POINT('Ctrl Pts',(-0.053514326589391,-0.146059658514288,
-0.775278701711074));
#78774=CARTESIAN_POINT('Ctrl Pts',(-0.0523999236604124,-0.146463153121103,
-0.775191614930757));
#78775=CARTESIAN_POINT('Ctrl Pts',(-0.050619487413628,-0.147084876565803,
-0.775054152215269));
#78776=CARTESIAN_POINT('Ctrl Pts',(-0.0499564302855662,-0.147311399915856,
-0.775003325200406));
#78777=CARTESIAN_POINT('Ctrl Pts',(-0.0486788244400447,-0.147738256041039,
-0.774906121333233));
#78778=CARTESIAN_POINT('Ctrl Pts',(-0.0480645264175407,-0.147939249579884,
-0.774859709962524));
#78779=CARTESIAN_POINT('Ctrl Pts',(-0.0465378184976351,-0.148428263307493,
-0.774745133454824));
#78780=CARTESIAN_POINT('Ctrl Pts',(-0.0456239496969946,-0.148711711830498,
-0.774677226394651));
#78781=CARTESIAN_POINT('Ctrl Pts',(-0.0423337696441344,-0.149699019311516,
-0.774434968570961));
#78782=CARTESIAN_POINT('Ctrl Pts',(-0.0399431932220235,-0.150354539262761,
-0.77426309639432));
#78783=CARTESIAN_POINT('Ctrl Pts',(-0.0284462463219715,-0.153213515720549,
-0.773451669167112));
#78784=CARTESIAN_POINT('Ctrl Pts',(-0.019168107651984,-0.154648600244095,
-0.772840966160701));
#78785=CARTESIAN_POINT('Ctrl Pts',(-0.00157081811658123,-0.15576134675307,
-0.771678043984229));
#78786=CARTESIAN_POINT('Ctrl Pts',(0.00670230030455253,-0.155624936353979,
-0.771129289911328));
#78787=CARTESIAN_POINT('Ctrl Pts',(0.0173029677610404,-0.154603097077782,
-0.770396184701846));
#78788=CARTESIAN_POINT('Ctrl Pts',(0.019675335927424,-0.154319118797238,
-0.770230237335172));
#78789=CARTESIAN_POINT('Ctrl Pts',(0.0233390549807971,-0.153794709972185,
-0.769970529580591));
#78790=CARTESIAN_POINT('Ctrl Pts',(0.0246355499457885,-0.153592362422327,
-0.76987795714009));
#78791=CARTESIAN_POINT('Ctrl Pts',(0.0270385882975622,-0.153186105583339,
-0.769705051736707));
#78792=CARTESIAN_POINT('Ctrl Pts',(0.0281457866905497,-0.15298654441234,
-0.769624860864986));
#78793=CARTESIAN_POINT('Ctrl Pts',(0.0306082602684932,-0.152515072832981,
-0.769445290773247));
#78794=CARTESIAN_POINT('Ctrl Pts',(0.0319622568503667,-0.152237074812078,
-0.769345724736426));
#78795=CARTESIAN_POINT('Ctrl Pts',(0.0354097445539801,-0.151481230192004,
-0.769090011064117));
#78796=CARTESIAN_POINT('Ctrl Pts',(0.0374973116462244,-0.150978024507789,
-0.76893307687826));
#78797=CARTESIAN_POINT('Ctrl Pts',(0.0495751899860725,-0.147800728363296,
-0.768012496422411));
#78798=CARTESIAN_POINT('Ctrl Pts',(0.0592876576204334,-0.144179255168847,
-0.767219055379777));
#78799=CARTESIAN_POINT('Ctrl Pts',(0.0742654154855587,-0.136823785911608,
-0.7659262439432));
#78800=CARTESIAN_POINT('Ctrl Pts',(0.0797870575307063,-0.133679216994205,
-0.765433391095634));
#78801=CARTESIAN_POINT('Ctrl Pts',(0.0869641792978983,-0.128988320546768,
-0.764781252227293));
#78802=CARTESIAN_POINT('Ctrl Pts',(0.0888008267869434,-0.127730848093961,
-0.764613311690958));
#78803=CARTESIAN_POINT('Ctrl Pts',(0.0919303011013704,-0.125488090789782,
-0.764326081944204));
#78804=CARTESIAN_POINT('Ctrl Pts',(0.0932358179562072,-0.124521178874232,
-0.764205923840216));
#78805=CARTESIAN_POINT('Ctrl Pts',(0.0951539725622292,-0.123053440510008,
-0.764029153775479));
#78806=CARTESIAN_POINT('Ctrl Pts',(0.0957782768439896,-0.122568142161201,
-0.763971583962522));
#78807=CARTESIAN_POINT('Ctrl Pts',(0.0968475330359851,-0.121723804822965,
-0.763872958779872));
#78808=CARTESIAN_POINT('Ctrl Pts',(0.0972942356299957,-0.121367050967584,
-0.763831751121603));
#78809=CARTESIAN_POINT('Ctrl Pts',(0.098340598422019,-0.120521895377861,
-0.763735212085814));
#78810=CARTESIAN_POINT('Ctrl Pts',(0.0989385960178016,-0.120031474409887,
-0.763680024391608));
#78811=CARTESIAN_POINT('Ctrl Pts',(0.100676177529508,-0.1185846658575,-0.763519536724081));
#78812=CARTESIAN_POINT('Ctrl Pts',(0.101805766505949,-0.11761633401134,
-0.763415038428798));
#78813=CARTESIAN_POINT('Ctrl Pts',(0.111789903690692,-0.108805873041389,
-0.762488049101127));
#78814=CARTESIAN_POINT('Ctrl Pts',(0.119738237295135,-0.0999926950713225,
-0.761723909468899));
#78815=CARTESIAN_POINT('Ctrl Pts',(0.130940314683007,-0.0842968972731342,
-0.760449307373388));
#78816=CARTESIAN_POINT('Ctrl Pts',(0.134827341827729,-0.0779288240368804,
-0.759951811849063));
#78817=CARTESIAN_POINT('Ctrl Pts',(0.139289708612341,-0.0692776632389138,
-0.759280782714919));
#78818=CARTESIAN_POINT('Ctrl Pts',(0.140291708173744,-0.06722539136633,
-0.759121986540296));
#78819=CARTESIAN_POINT('Ctrl Pts',(0.141788728516491,-0.0639798783776641,
-0.758871022961164));
#78820=CARTESIAN_POINT('Ctrl Pts',(0.142314707461589,-0.0628012120356809,
-0.758779914810016));
#78821=CARTESIAN_POINT('Ctrl Pts',(0.143272316272515,-0.0605814799807456,
-0.758608322154654));
#78822=CARTESIAN_POINT('Ctrl Pts',(0.14370742048909,-0.0595419977928306,
-0.758527961760874));
#78823=CARTESIAN_POINT('Ctrl Pts',(0.144661787581648,-0.0571905621563504,
-0.758346116107824));
#78824=CARTESIAN_POINT('Ctrl Pts',(0.145174564354448,-0.0558761023018297,
-0.758244421455909));
#78825=CARTESIAN_POINT('Ctrl Pts',(0.146457315468574,-0.0524509728805534,
-0.757979237575435));
#78826=CARTESIAN_POINT('Ctrl Pts',(0.147199543685678,-0.0503303405854174,
-0.757814858431232));
#78827=CARTESIAN_POINT('Ctrl Pts',(0.152077968222773,-0.0353598014627387,
-0.756652562841552));
#78828=CARTESIAN_POINT('Ctrl Pts',(0.154571177575083,-0.0220371597327425,
-0.755601291625571));
#78829=CARTESIAN_POINT('Ctrl Pts',(0.1556411458181,-0.00263213073898166,
-0.754100906639943));
#78830=CARTESIAN_POINT('Ctrl Pts',(0.15562816859051,0.00331412458608902,
-0.753646471357276));
#78831=CARTESIAN_POINT('Ctrl Pts',(0.155203207089608,0.0104510875541612,
-0.753117187221257));
#78832=CARTESIAN_POINT('Ctrl Pts',(0.155117393446305,0.0116556943521194,
-0.753028415403978));
#78833=CARTESIAN_POINT('Ctrl Pts',(0.154959232546414,0.0135623186404717,
-0.752888925637902));
#78834=CARTESIAN_POINT('Ctrl Pts',(0.154896124563317,0.0142650231751105,
-0.752837734528911));
#78835=CARTESIAN_POINT('Ctrl Pts',(0.15476627017511,0.0156082939101141,
-0.75274032895042));
#78836=CARTESIAN_POINT('Ctrl Pts',(0.154700324040586,0.0162489071035265,
-0.752694075113463));
#78837=CARTESIAN_POINT('Ctrl Pts',(0.15452795744682,0.0178270320719447,
-0.752580586249592));
#78838=CARTESIAN_POINT('Ctrl Pts',(0.154416979653269,0.0187640405495154,
-0.752513598066399));
#78839=CARTESIAN_POINT('Ctrl Pts',(0.153994269122355,0.0220748593060364,
-0.752278116796344));
#78840=CARTESIAN_POINT('Ctrl Pts',(0.153636250419674,0.0244425543690881,
-0.752111926428026));
#78841=CARTESIAN_POINT('Ctrl Pts',(0.15137788180538,0.0373537521860477,
-0.751213138636186));
#78842=CARTESIAN_POINT('Ctrl Pts',(0.14844670491002,0.0476884769169512,
-0.750519487289276));
#78843=CARTESIAN_POINT('Ctrl Pts',(0.142080865755604,0.0636444168829828,
-0.749383222567223));
#78844=CARTESIAN_POINT('Ctrl Pts',(0.139313940396103,0.0694924297117077,
-0.748951702793932));
#78845=CARTESIAN_POINT('Ctrl Pts',(0.134870605302023,0.0775448084152426,
-0.748321329422321));
#78846=CARTESIAN_POINT('Ctrl Pts',(0.133486896015562,0.079903219840317,
-0.748132051624624));
#78847=CARTESIAN_POINT('Ctrl Pts',(0.131312494053935,0.08339505442286,-0.747843935807861));
#78848=CARTESIAN_POINT('Ctrl Pts',(0.130567630321665,0.0845564893583829,
-0.747746752090606));
#78849=CARTESIAN_POINT('Ctrl Pts',(0.129187608247858,0.086646579928307,
-0.747569294831481));
#78850=CARTESIAN_POINT('Ctrl Pts',(0.128557630741107,0.087578555568169,
-0.747489217874907));
#78851=CARTESIAN_POINT('Ctrl Pts',(0.127169876883921,0.0895843290581817,
-0.747314758014028));
#78852=CARTESIAN_POINT('Ctrl Pts',(0.126408494455939,0.0906555124269333,
-0.747220242767586));
#78853=CARTESIAN_POINT('Ctrl Pts',(0.124258508827839,0.0936005593540994,
-0.746956544887662));
#78854=CARTESIAN_POINT('Ctrl Pts',(0.122841248641737,0.0954529636806026,
-0.746786273784501));
#78855=CARTESIAN_POINT('Ctrl Pts',(0.115629787882961,0.104451873060104,
-0.745936484925558));
#78856=CARTESIAN_POINT('Ctrl Pts',(0.109256642187624,0.111099462666316,
-0.745234706993985));
#78857=CARTESIAN_POINT('Ctrl Pts',(0.102342226135006,0.117140391196766,
-0.744524458909986));
#78858=CARTESIAN_POINT('Origin',(0.,0.,-1.10400562256037));
#78859=CARTESIAN_POINT('',(0.102342242837719,0.117140376604078,-0.660690965868517));
#78860=CARTESIAN_POINT('',(0.102342242758987,0.117140376672865,-0.674376033428004));
#78861=CARTESIAN_POINT('',(0.10234224283772,0.117140376604078,-1.10400562256037));
#78862=CARTESIAN_POINT('',(-0.15554997247323,9.25395981759249E-5,-0.705194377443794));
#78863=CARTESIAN_POINT('Ctrl Pts',(-0.155549972473265,9.25395397988971E-5,
-0.70519437743963));
#78864=CARTESIAN_POINT('Ctrl Pts',(-0.155556164015641,-0.0103148414372451,
-0.704452036543397));
#78865=CARTESIAN_POINT('Ctrl Pts',(-0.154513525352864,-0.0207250453155431,
-0.703709695647164));
#78866=CARTESIAN_POINT('Ctrl Pts',(-0.152446462480172,-0.0309172860594462,
-0.702967354750931));
#78867=CARTESIAN_POINT('Ctrl Pts',(-0.150292093954745,-0.0415400121275881,
-0.70219365991895));
#78868=CARTESIAN_POINT('Ctrl Pts',(-0.147024820678378,-0.0519248668138346,
-0.701419965086969));
#78869=CARTESIAN_POINT('Ctrl Pts',(-0.142730557982281,-0.061836803912125,
-0.700646270254988));
#78870=CARTESIAN_POINT('Ctrl Pts',(-0.138436295286185,-0.0717487410104155,
-0.699872575423007));
#78871=CARTESIAN_POINT('Ctrl Pts',(-0.13311562594688,-0.0811868260858244,
-0.699098880591026));
#78872=CARTESIAN_POINT('Ctrl Pts',(-0.126907404165646,-0.0899461687229495,
-0.698325185759045));
#78873=CARTESIAN_POINT('Ctrl Pts',(-0.120989086182212,-0.0982964785023233,
-0.69758761996337));
#78874=CARTESIAN_POINT('Ctrl Pts',(-0.114221086521816,-0.106091191222701,
-0.696850054167695));
#78875=CARTESIAN_POINT('Ctrl Pts',(-0.106731669265914,-0.113155438560025,
-0.69611248837202));
#78876=CARTESIAN_POINT('Ctrl Pts',(-0.0992244483991311,-0.120236478807459,
-0.695373169257765));
#78877=CARTESIAN_POINT('Ctrl Pts',(-0.0909929491436147,-0.126582832737307,
-0.694633850143511));
#78878=CARTESIAN_POINT('Ctrl Pts',(-0.0822061882775618,-0.132052811817371,
-0.693894531029256));
#78879=CARTESIAN_POINT('Ctrl Pts',(-0.0734602750557194,-0.137497362214135,
-0.69315864884069));
#78880=CARTESIAN_POINT('Ctrl Pts',(-0.0641650414194839,-0.142073172211821,
-0.692422766652123));
#78881=CARTESIAN_POINT('Ctrl Pts',(-0.0545162404005626,-0.14568384273003,
-0.691686884463557));
#78882=CARTESIAN_POINT('Ctrl Pts',(-0.0447998425313615,-0.149319808614363,
-0.690945846886458));
#78883=CARTESIAN_POINT('Ctrl Pts',(-0.0347257889390185,-0.151976714260062,
-0.690204809309359));
#78884=CARTESIAN_POINT('Ctrl Pts',(-0.0245109579853446,-0.153606690735269,
-0.68946377173226));
#78885=CARTESIAN_POINT('Ctrl Pts',(-0.0142961270316707,-0.155236667210476,
-0.688722734155162));
#78886=CARTESIAN_POINT('Ctrl Pts',(-0.00394147099037896,-0.155839693150005,
-0.687981696578063));
#78887=CARTESIAN_POINT('Ctrl Pts',(0.00633312724545194,-0.15542102174189,
-0.687240659000964));
#78888=CARTESIAN_POINT('Ctrl Pts',(0.0165595887075161,-0.155004311820773,
-0.686503093205183));
#78889=CARTESIAN_POINT('Ctrl Pts',(0.0267827483270296,-0.153572399386593,
-0.685765527409402));
#78890=CARTESIAN_POINT('Ctrl Pts',(0.0367860928839178,-0.151137638827447,
-0.685027961613621));
#78891=CARTESIAN_POINT('Ctrl Pts',(0.0468132170800498,-0.148697090431302,
-0.684288642499393));
#78892=CARTESIAN_POINT('Ctrl Pts',(0.056618543836475,-0.14524899597409,
-0.683549323385165));
#78893=CARTESIAN_POINT('Ctrl Pts',(0.0659911969356596,-0.140857958337465,
-0.682810004270937));
#78894=CARTESIAN_POINT('Ctrl Pts',(0.0753202787130791,-0.136487333631066,
-0.68207412208227));
#78895=CARTESIAN_POINT('Ctrl Pts',(0.0842198547940364,-0.131182906131836,
-0.681338239893603));
#78896=CARTESIAN_POINT('Ctrl Pts',(0.0925024753279771,-0.125056365524499,
-0.680602357704937));
#78897=CARTESIAN_POINT('Ctrl Pts',(0.100843121624735,-0.118886904057669,
-0.679861320127928));
#78898=CARTESIAN_POINT('Ctrl Pts',(0.108557362934198,-0.11188431993569,
-0.679120282550919));
#78899=CARTESIAN_POINT('Ctrl Pts',(0.115486949262858,-0.104204448321355,
-0.678379244973911));
#78900=CARTESIAN_POINT('Ctrl Pts',(0.122416535591518,-0.0965245767070206,
-0.677638207396902));
#78901=CARTESIAN_POINT('Ctrl Pts',(0.128560930459896,-0.0881682046654229,
-0.676897169819893));
#78902=CARTESIAN_POINT('Ctrl Pts',(0.133804802816841,-0.0793226149540368,
-0.676156132242885));
#78903=CARTESIAN_POINT('Ctrl Pts',(0.139024107490351,-0.0705184670690396,
-0.675418566446912));
#78904=CARTESIAN_POINT('Ctrl Pts',(0.143390134454677,-0.0611642608263117,
-0.67468100065094));
#78905=CARTESIAN_POINT('Ctrl Pts',(0.14679534359319,-0.0514483196942064,
-0.673943434854968));
#78906=CARTESIAN_POINT('Ctrl Pts',(0.150208647487746,-0.0417092821324859,
-0.673204115740787));
#78907=CARTESIAN_POINT('Ctrl Pts',(0.152656113760471,-0.0316076141012754,
-0.672464796626607));
#78908=CARTESIAN_POINT('Ctrl Pts',(0.154077094241808,-0.0213553630266754,
-0.671725477512427));
#78909=CARTESIAN_POINT('Ctrl Pts',(0.155491468910191,-0.0111507723202771,
-0.670989595323556));
#78910=CARTESIAN_POINT('Ctrl Pts',(0.155888749203406,-0.000797918900235615,
-0.670253713134686));
#78911=CARTESIAN_POINT('Ctrl Pts',(0.155260536823854,0.00948515709772491,
-0.669517830945815));
#78912=CARTESIAN_POINT('Ctrl Pts',(0.154627923361372,0.0198402734943268,
-0.66877679336898));
#78913=CARTESIAN_POINT('Ctrl Pts',(0.152955437516772,0.0301236821901649,
-0.668035755792145));
#78914=CARTESIAN_POINT('Ctrl Pts',(0.150287607839454,0.040117794429585,
-0.667294718215309));
#78915=CARTESIAN_POINT('Ctrl Pts',(0.147619778162136,0.0501119066690056,
-0.666553680638474));
#78916=CARTESIAN_POINT('Ctrl Pts',(0.143956972646875,0.059815843895503,
-0.665812643061639));
#78917=CARTESIAN_POINT('Ctrl Pts',(0.139393467325035,0.0690308899486625,
-0.665071605484804));
#78918=CARTESIAN_POINT('Ctrl Pts',(0.134850423137525,0.0782046190137071,
-0.664333890456828));
#78919=CARTESIAN_POINT('Ctrl Pts',(0.129381001077389,0.0869620440593471,
-0.663596175428853));
#78920=CARTESIAN_POINT('Ctrl Pts',(0.123084657699114,0.0951103019608916,
-0.662858460400877));
#78921=CARTESIAN_POINT('Ctrl Pts',(0.116918189018237,0.103090485717538,
-0.662135962223424));
#78922=CARTESIAN_POINT('Ctrl Pts',(0.109959136079929,0.11048571182954,-0.66141346404597));
#78923=CARTESIAN_POINT('Ctrl Pts',(0.102342242837719,0.117140376604078,
-0.660690965868517));
#78924=CARTESIAN_POINT('Ctrl Pts',(0.10234224283772,0.117140376604078,-0.730690163752328));
#78925=CARTESIAN_POINT('Ctrl Pts',(0.094621461509984,0.123885805468548,
-0.729953349882094));
#78926=CARTESIAN_POINT('Ctrl Pts',(0.0862069888207784,0.129885566877293,
-0.729216536011859));
#78927=CARTESIAN_POINT('Ctrl Pts',(0.0772670487836427,0.135002243211978,
-0.728479722141624));
#78928=CARTESIAN_POINT('Ctrl Pts',(0.0683342552066571,0.140114829348813,
-0.727743497269854));
#78929=CARTESIAN_POINT('Ctrl Pts',(0.0588775918214991,0.144345209434971,
-0.727007272398085));
#78930=CARTESIAN_POINT('Ctrl Pts',(0.0490940272787818,0.147599386806146,
-0.726271047526315));
#78931=CARTESIAN_POINT('Ctrl Pts',(0.0393158995224998,0.150851755811125,
-0.725535231779193));
#78932=CARTESIAN_POINT('Ctrl Pts',(0.029212111985139,0.153128710345636,
-0.724799416032071));
#78933=CARTESIAN_POINT('Ctrl Pts',(0.0189961027279428,0.154385720133533,
-0.724063600284949));
#78934=CARTESIAN_POINT('Ctrl Pts',(0.00875568083771532,0.155645733728287,
-0.72332602619958));
#78935=CARTESIAN_POINT('Ctrl Pts',(-0.00159657035185435,0.155880862690202,
-0.722588452114211));
#78936=CARTESIAN_POINT('Ctrl Pts',(-0.0118424412810255,0.155098546364901,
-0.721850878028841));
#78937=CARTESIAN_POINT('Ctrl Pts',(-0.0181242715147549,0.154618901600822,
-0.721398665110962));
#78938=CARTESIAN_POINT('Ctrl Pts',(-0.0243661104056406,0.153757839952673,
-0.720946452193084));
#78939=CARTESIAN_POINT('Ctrl Pts',(-0.0305193452349855,0.152526627401342,
-0.720494239275205));
#78940=CARTESIAN_POINT('Ctrl Pts',(-0.0405553600408,0.150518501962128,-0.719756673480126));
#78941=CARTESIAN_POINT('Ctrl Pts',(-0.0504296230703562,0.147508137328358,
-0.719019107685047));
#78942=CARTESIAN_POINT('Ctrl Pts',(-0.0599302045978709,0.143541537809992,
-0.718281541889969));
#78943=CARTESIAN_POINT('Ctrl Pts',(-0.069453370623341,0.139565509010012,
-0.717542222775565));
#78944=CARTESIAN_POINT('Ctrl Pts',(-0.0786001636476661,0.134628914473355,
-0.716802903661162));
#78945=CARTESIAN_POINT('Ctrl Pts',(-0.0871723787096418,0.128828486330092,
-0.716063584546758));
#78946=CARTESIAN_POINT('Ctrl Pts',(-0.0957047434925588,0.123055023058627,
-0.715327702358844));
#78947=CARTESIAN_POINT('Ctrl Pts',(-0.103667086401764,0.116426259922342,
-0.71459182017093));
#78948=CARTESIAN_POINT('Ctrl Pts',(-0.110891692655501,0.109081781246906,
-0.713855937983016));
#78949=CARTESIAN_POINT('Ctrl Pts',(-0.118166912528549,0.101685849158695,
-0.713114900405367));
#78950=CARTESIAN_POINT('Ctrl Pts',(-0.124693343388765,0.0935648021931653,
-0.712373862827719));
#78951=CARTESIAN_POINT('Ctrl Pts',(-0.130339004140216,0.0848972702725871,
-0.71163282525007));
#78952=CARTESIAN_POINT('Ctrl Pts',(-0.135984664891667,0.0762297383520086,
-0.710891787672421));
#78953=CARTESIAN_POINT('Ctrl Pts',(-0.140749148507157,0.067016582644528,
-0.710150750094773));
#78954=CARTESIAN_POINT('Ctrl Pts',(-0.144547776091199,0.0574607946959366,
-0.709409712517124));
#78955=CARTESIAN_POINT('Ctrl Pts',(-0.148790588070324,0.0467876211138281,
-0.70858202329467));
#78956=CARTESIAN_POINT('Ctrl Pts',(-0.151855992978236,0.0356211012833882,
-0.707754334072216));
#78957=CARTESIAN_POINT('Ctrl Pts',(-0.153653437845324,0.0242161833969177,
-0.706926644849762));
#78958=CARTESIAN_POINT('Ctrl Pts',(-0.154907392861616,0.0162597479835195,
-0.706349222381106));
#78959=CARTESIAN_POINT('Ctrl Pts',(-0.155545156440655,0.00818781718077903,
-0.70577179991245));
#78960=CARTESIAN_POINT('Ctrl Pts',(-0.15554997247323,9.25395981750804E-5,
-0.705194377443794));
#78961=CARTESIAN_POINT('Ctrl Pts',(0.102342226135006,0.117140391196766,
-0.744524458909986));
#78962=CARTESIAN_POINT('Ctrl Pts',(0.0992816917559716,0.11981429298515,
-0.744210081142987));
#78963=CARTESIAN_POINT('Ctrl Pts',(0.0961151016480072,0.122369357141659,
-0.74389430617453));
#78964=CARTESIAN_POINT('Ctrl Pts',(0.087743192154423,0.128597967857729,
-0.743087731012877));
#78965=CARTESIAN_POINT('Ctrl Pts',(0.0824082290926953,0.132080306284147,
-0.742599763532665));
#78966=CARTESIAN_POINT('Ctrl Pts',(0.0758110869509018,0.135830693983384,
-0.742037792075191));
#78967=CARTESIAN_POINT('Ctrl Pts',(0.0747407077159392,0.136422597797972,
-0.741947858731752));
#78968=CARTESIAN_POINT('Ctrl Pts',(0.073039099563667,0.137337521776461,
-0.741806972700145));
#78969=CARTESIAN_POINT('Ctrl Pts',(0.072412480296711,0.137668942406708,
-0.741755531400762));
#78970=CARTESIAN_POINT('Ctrl Pts',(0.071213587964429,0.13829258918564,-0.741657977164177));
#78971=CARTESIAN_POINT('Ctrl Pts',(0.0706417418346042,0.138585568014733,
-0.741611821584449));
#78972=CARTESIAN_POINT('Ctrl Pts',(0.0692333889481668,0.139296139332652,
-0.741499033309447));
#78973=CARTESIAN_POINT('Ctrl Pts',(0.0683948839642774,0.139709758215228,
-0.74143264023381));
#78974=CARTESIAN_POINT('Ctrl Pts',(0.0654442578128729,0.141132314963904,
-0.74120147566794));
#78975=CARTESIAN_POINT('Ctrl Pts',(0.0633130232656981,0.142101174413875,
-0.741038898343776));
#78976=CARTESIAN_POINT('Ctrl Pts',(0.0512567778007329,0.147256808209453,
-0.740139076246891));
#78977=CARTESIAN_POINT('Ctrl Pts',(0.0409388087412304,0.15045228295911,
-0.739441712389885));
#78978=CARTESIAN_POINT('Ctrl Pts',(0.0252155040855959,0.153582646212186,
-0.738381362479128));
#78979=CARTESIAN_POINT('Ctrl Pts',(0.020010149512094,0.154347136340895,
-0.738030994124772));
#78980=CARTESIAN_POINT('Ctrl Pts',(0.0112395068769008,0.155184081548472,
-0.737432382908579));
#78981=CARTESIAN_POINT('Ctrl Pts',(0.00769238439801505,0.155400288626378,
-0.737188081701392));
#78982=CARTESIAN_POINT('Ctrl Pts',(0.00262051371842576,0.155535364082152,
-0.736833883427955));
#78983=CARTESIAN_POINT('Ctrl Pts',(0.00109938221013814,0.155553552335351,
-0.736727033071687));
#78984=CARTESIAN_POINT('Ctrl Pts',(-0.00156142240452312,0.155546338365351,
-0.736538916565582));
#78985=CARTESIAN_POINT('Ctrl Pts',(-0.00270102273462084,0.155530722913021,
-0.736457959507899));
#78986=CARTESIAN_POINT('Ctrl Pts',(-0.00507123498229626,0.155472187697642,
-0.73628872077709));
#78987=CARTESIAN_POINT('Ctrl Pts',(-0.00630171035188463,0.155427175416405,
-0.736200379666704));
#78988=CARTESIAN_POINT('Ctrl Pts',(-0.00952720508736266,0.155270818578288,
-0.735967477137352));
#78989=CARTESIAN_POINT('Ctrl Pts',(-0.0115207809893011,0.155135636327244,
-0.735822188510033));
#78990=CARTESIAN_POINT('Ctrl Pts',(-0.022211329520695,0.154203529350073,
-0.735035506198311));
#78991=CARTESIAN_POINT('Ctrl Pts',(-0.0308307132378416,0.152713756217094,
-0.734372952943605));
#78992=CARTESIAN_POINT('Ctrl Pts',(-0.04550645091284,0.148883837758629,
-0.733202833956973));
#78993=CARTESIAN_POINT('Ctrl Pts',(-0.05162765390214,0.146873479861896,
-0.732701743721254));
#78994=CARTESIAN_POINT('Ctrl Pts',(-0.062443237373995,0.142561408318975,
-0.731805336973281));
#78995=CARTESIAN_POINT('Ctrl Pts',(-0.0671804717886798,0.140391271214905,
-0.731408739860987));
#78996=CARTESIAN_POINT('Ctrl Pts',(-0.0728414383288936,0.137445642443011,
-0.730936667598119));
#78997=CARTESIAN_POINT('Ctrl Pts',(-0.073876381750402,0.136892148072412,
-0.73085044695573));
#78998=CARTESIAN_POINT('Ctrl Pts',(-0.0755168808649026,0.135990774057516,
-0.73071402694491));
#78999=CARTESIAN_POINT('Ctrl Pts',(-0.0761265053878712,0.135650452092503,
-0.730663387689268));
#79000=CARTESIAN_POINT('Ctrl Pts',(-0.0772971901348672,0.134986541327693,
-0.730566280688034));
#79001=CARTESIAN_POINT('Ctrl Pts',(-0.0778585501977418,0.134663536726079,
-0.730519780964233));
#79002=CARTESIAN_POINT('Ctrl Pts',(-0.0791160054150711,0.133929509934786,
-0.730415730943672));
#79003=CARTESIAN_POINT('Ctrl Pts',(-0.0798109578556671,0.133516542139265,
-0.730358301957721));
#79004=CARTESIAN_POINT('Ctrl Pts',(-0.0822660292145733,0.132031624421179,
-0.730155574334149));
#79005=CARTESIAN_POINT('Ctrl Pts',(-0.0840081188800761,0.130930082144696,
-0.730012001848213));
#79006=CARTESIAN_POINT('Ctrl Pts',(-0.0938409267653244,0.124435599499604,
-0.729200137205314));
#79007=CARTESIAN_POINT('Ctrl Pts',(-0.101434615885145,0.118327515291702,
-0.728566227933881));
#79008=CARTESIAN_POINT('Ctrl Pts',(-0.114454298389645,0.105674413602827,
-0.727369211543443));
#79009=CARTESIAN_POINT('Ctrl Pts',(-0.120011455342144,0.0993181504842108,
-0.726809894187585));
#79010=CARTESIAN_POINT('Ctrl Pts',(-0.126459721081835,0.0906065595270534,
-0.726064006081659));
#79011=CARTESIAN_POINT('Ctrl Pts',(-0.127848147299566,0.0886366732353807,
-0.72589665562401));
#79012=CARTESIAN_POINT('Ctrl Pts',(-0.129923354084219,0.0855421378597002,
-0.725635233860369));
#79013=CARTESIAN_POINT('Ctrl Pts',(-0.130642584522529,0.0844396246227322,
-0.725542376527022));
#79014=CARTESIAN_POINT('Ctrl Pts',(-0.13195027207576,0.0823783550099891,
-0.725369206656714));
#79015=CARTESIAN_POINT('Ctrl Pts',(-0.13254249286479,0.0814220801689962,
-0.725289039655962));
#79016=CARTESIAN_POINT('Ctrl Pts',(-0.133836605675194,0.0792809053538552,
-0.725109867626132));
#79017=CARTESIAN_POINT('Ctrl Pts',(-0.134533229737273,0.0780929500259457,
-0.725010679803009));
#79018=CARTESIAN_POINT('Ctrl Pts',(-0.136266799344912,0.0750446377506869,
-0.724756636720924));
#79019=CARTESIAN_POINT('Ctrl Pts',(-0.137281447262741,0.0731720005984846,
-0.724601012552606));
#79020=CARTESIAN_POINT('Ctrl Pts',(-0.144331719028053,0.0594968841098366,
-0.723467199148181));
#79021=CARTESIAN_POINT('Ctrl Pts',(-0.14887408473509,0.0469882461764634,
-0.722437247337514));
#79022=CARTESIAN_POINT('Ctrl Pts',(-0.153061670915404,0.0283272572319096,
-0.720958902415645));
#79023=CARTESIAN_POINT('Ctrl Pts',(-0.154022297012498,0.0225267498717688,
-0.720508196758153));
#79024=CARTESIAN_POINT('Ctrl Pts',(-0.154815110970317,0.0151783165606813,
-0.719957806148216));
#79025=CARTESIAN_POINT('Ctrl Pts',(-0.154955668860915,0.0136689801187794,
-0.719845851519961));
#79026=CARTESIAN_POINT('Ctrl Pts',(-0.155134296591403,0.0113905548423789,
-0.719678726132901));
#79027=CARTESIAN_POINT('Ctrl Pts',(-0.155188752518389,0.0106228940196766,
-0.719622737674124));
#79028=CARTESIAN_POINT('Ctrl Pts',(-0.155277781995037,0.00922046481166052,
-0.71952107550627));
#79029=CARTESIAN_POINT('Ctrl Pts',(-0.155314163911447,0.00858586456539685,
-0.719475309689463));
#79030=CARTESIAN_POINT('Ctrl Pts',(-0.155388410088042,0.0071352464649925,
-0.719371221166804));
#79031=CARTESIAN_POINT('Ctrl Pts',(-0.155423738172151,0.00631913149340646,
-0.719313036946951));
#79032=CARTESIAN_POINT('Ctrl Pts',(-0.155516790167648,0.00369041454213425,
-0.719126724232841));
#79033=CARTESIAN_POINT('Ctrl Pts',(-0.155549248849663,0.00187699144480572,
-0.718999878131621));
#79034=CARTESIAN_POINT('Ctrl Pts',(-0.155553661810709,-0.00896411500264388,
-0.718249377611239));
#79035=CARTESIAN_POINT('Ctrl Pts',(-0.154771460006158,-0.0179759038482187,
-0.717657240668742));
#79036=CARTESIAN_POINT('Ctrl Pts',(-0.151558321205572,-0.0362971868528248,
-0.716432030666671));
#79037=CARTESIAN_POINT('Ctrl Pts',(-0.149038636047285,-0.0455507027420927,
-0.715800666335872));
#79038=CARTESIAN_POINT('Ctrl Pts',(-0.144926839144654,-0.0565392993009497,
-0.714993137958498));
#79039=CARTESIAN_POINT('Ctrl Pts',(-0.144126662870719,-0.058548999524496,
-0.714843046080432));
#79040=CARTESIAN_POINT('Ctrl Pts',(-0.142745120489696,-0.0618187374853886,
-0.71459447008077));
#79041=CARTESIAN_POINT('Ctrl Pts',(-0.142188321550449,-0.0630888795504469,
-0.71449680419558));
#79042=CARTESIAN_POINT('Ctrl Pts',(-0.141149103598201,-0.0653758310489519,
-0.714318843939308));
#79043=CARTESIAN_POINT('Ctrl Pts',(-0.140672485639194,-0.0663951835227835,
-0.714238751754864));
#79044=CARTESIAN_POINT('Ctrl Pts',(-0.139617800852295,-0.0685885151165409,
-0.714064693602544));
#79045=CARTESIAN_POINT('Ctrl Pts',(-0.139035899206212,-0.0697605422836783,
-0.713970599958849));
#79046=CARTESIAN_POINT('Ctrl Pts',(-0.137358187712264,-0.0730352834106492,
-0.713704548575875));
#79047=CARTESIAN_POINT('Ctrl Pts',(-0.136229029170661,-0.0751204021982916,
-0.713531443769468));
#79048=CARTESIAN_POINT('Ctrl Pts',(-0.131024625489795,-0.0842274218719544,
-0.712758381064827));
#79049=CARTESIAN_POINT('Ctrl Pts',(-0.126451529956137,-0.090948803060077,
-0.712141236413024));
#79050=CARTESIAN_POINT('Ctrl Pts',(-0.115699175673375,-0.104364197036007,
-0.710814612431317));
#79051=CARTESIAN_POINT('Ctrl Pts',(-0.109413625780804,-0.110936252433604,
-0.710105190608367));
#79052=CARTESIAN_POINT('Ctrl Pts',(-0.100455876751058,-0.11879598308888,
-0.709202028793471));
#79053=CARTESIAN_POINT('Ctrl Pts',(-0.0982699620206477,-0.120610471543629,
-0.708989160596649));
#79054=CARTESIAN_POINT('Ctrl Pts',(-0.0952449155553769,-0.122984626572255,
-0.708705836099892));
#79055=CARTESIAN_POINT('Ctrl Pts',(-0.0944483887885326,-0.123597387956105,
-0.708632252926842));
#79056=CARTESIAN_POINT('Ctrl Pts',(-0.093169661825641,-0.124561520660955,
-0.708515808394829));
#79057=CARTESIAN_POINT('Ctrl Pts',(-0.0926912991225362,-0.124917898690775,
-0.708472616972283));
#79058=CARTESIAN_POINT('Ctrl Pts',(-0.0916716508948487,-0.125668449692673,
-0.708381354556019));
#79059=CARTESIAN_POINT('Ctrl Pts',(-0.0911298455352361,-0.12606189796134,
-0.708333335566216));
#79060=CARTESIAN_POINT('Ctrl Pts',(-0.0897390442549637,-0.127058217444576,
-0.708211231123739));
#79061=CARTESIAN_POINT('Ctrl Pts',(-0.088886486288689,-0.127656098149074,
-0.70813747323873));
#79062=CARTESIAN_POINT('Ctrl Pts',(-0.085207969919963,-0.130181040967754,
-0.707823573278467));
#79063=CARTESIAN_POINT('Ctrl Pts',(-0.0823246481788521,-0.132023323810313,
-0.707588381127736));
#79064=CARTESIAN_POINT('Ctrl Pts',(-0.0734929468294431,-0.137264322270465,
-0.706892411792521));
#79065=CARTESIAN_POINT('Ctrl Pts',(-0.0673783989063612,-0.140366918619535,
-0.70644229674957));
#79066=CARTESIAN_POINT('Ctrl Pts',(-0.0522131573940497,-0.146841813022872,
-0.705356164979361));
#79067=CARTESIAN_POINT('Ctrl Pts',(-0.0430158029548496,-0.14979433680602,
-0.704720488039432));
#79068=CARTESIAN_POINT('Ctrl Pts',(-0.0314940139511692,-0.152343702801222,
-0.703908283545025));
#79069=CARTESIAN_POINT('Ctrl Pts',(-0.0293736650130515,-0.152766697052541,
-0.703758260061269));
#79070=CARTESIAN_POINT('Ctrl Pts',(-0.0258801966423407,-0.153388201423256,
-0.703509773536445));
#79071=CARTESIAN_POINT('Ctrl Pts',(-0.0245119736761926,-0.153612785408959,
-0.703412127693914));
#79072=CARTESIAN_POINT('Ctrl Pts',(-0.0220282374517586,-0.153986445673217,
-0.703234188432255));
#79073=CARTESIAN_POINT('Ctrl Pts',(-0.0209137490155912,-0.154141764870638,
-0.703154096967158));
#79074=CARTESIAN_POINT('Ctrl Pts',(-0.018499593368276,-0.154451547002176,
-0.702980022532081));
#79075=CARTESIAN_POINT('Ctrl Pts',(-0.0171994743716018,-0.154601724487356,
-0.702885911695391));
#79076=CARTESIAN_POINT('Ctrl Pts',(-0.013537886368753,-0.154977919076282,
-0.702619759232182));
#79077=CARTESIAN_POINT('Ctrl Pts',(-0.0111730113793886,-0.155166337987278,
-0.702446569133172));
#79078=CARTESIAN_POINT('Ctrl Pts',(-0.000690454988465145,-0.15576065332838,
-0.701672744691906));
#79079=CARTESIAN_POINT('Ctrl Pts',(0.00744628704844008,-0.155583976301972,
-0.701054883192174));
#79080=CARTESIAN_POINT('Ctrl Pts',(0.0245800810837738,-0.153864665123797,
-0.699726116744724));
#79081=CARTESIAN_POINT('Ctrl Pts',(0.0335323763558437,-0.152164727380259,
-0.699015260521745));
#79082=CARTESIAN_POINT('Ctrl Pts',(0.0449962346101666,-0.148926419812295,
-0.698112652310696));
#79083=CARTESIAN_POINT('Ctrl Pts',(0.0476863441962586,-0.148086983494662,
-0.69790153632695));
#79084=CARTESIAN_POINT('Ctrl Pts',(0.0513003490112249,-0.146850538171774,
-0.69762013390306));
#79085=CARTESIAN_POINT('Ctrl Pts',(0.052245213838097,-0.146517043861462,
-0.697546772307117));
#79086=CARTESIAN_POINT('Ctrl Pts',(0.0537468637978994,-0.145970655620525,
-0.697430587846476));
#79087=CARTESIAN_POINT('Ctrl Pts',(0.0543057417739201,-0.145763658409669,
-0.697387437464682));
#79088=CARTESIAN_POINT('Ctrl Pts',(0.0554906265918142,-0.145317040043381,
-0.69729616726777));
#79089=CARTESIAN_POINT('Ctrl Pts',(0.0561163036812781,-0.145076573807682,
-0.697248100178752));
#79090=CARTESIAN_POINT('Ctrl Pts',(0.0577130080627482,-0.144451037754202,
-0.697125714880949));
#79091=CARTESIAN_POINT('Ctrl Pts',(0.0586817675402088,-0.144060209367745,
-0.69705172723954));
#79092=CARTESIAN_POINT('Ctrl Pts',(0.062836518384689,-0.142335183730982,
-0.696735258029877));
#79093=CARTESIAN_POINT('Ctrl Pts',(0.0659817778331868,-0.140904726098666,
-0.696497827620692));
#79094=CARTESIAN_POINT('Ctrl Pts',(0.0753252473259032,-0.136273767735801,
-0.695791369067072));
#79095=CARTESIAN_POINT('Ctrl Pts',(0.0813585486116721,-0.132760056858453,
-0.695333379222897));
#79096=CARTESIAN_POINT('Ctrl Pts',(0.0949808041973258,-0.123548099193227,
-0.69425016844738));
#79097=CARTESIAN_POINT('Ctrl Pts',(0.10232384661509,-0.117538452668813,
-0.693625146920701));
#79098=CARTESIAN_POINT('Ctrl Pts',(0.110617496272003,-0.109381242221885,
-0.692824501079762));
#79099=CARTESIAN_POINT('Ctrl Pts',(0.112128606983927,-0.107831634280888,
-0.692674322245122));
#79100=CARTESIAN_POINT('Ctrl Pts',(0.114554371860651,-0.105237933512922,
-0.692425632495276));
#79101=CARTESIAN_POINT('Ctrl Pts',(0.115488284277159,-0.104212200520695,
-0.692327941136988));
#79102=CARTESIAN_POINT('Ctrl Pts',(0.117154716485394,-0.102332014455273,
-0.692149954195518));
#79103=CARTESIAN_POINT('Ctrl Pts',(0.1178919269267,-0.101481831978777,-0.692069861094677));
#79104=CARTESIAN_POINT('Ctrl Pts',(0.11946610854211,-0.0996261153610942,
-0.691895823614201));
#79105=CARTESIAN_POINT('Ctrl Pts',(0.120299742235132,-0.0986178775755117,
-0.6918017518011));
#79106=CARTESIAN_POINT('Ctrl Pts',(0.122607331319527,-0.0957541633233396,
-0.69153582871228));
#79107=CARTESIAN_POINT('Ctrl Pts',(0.124051690325616,-0.0938754199841913,
-0.691362832151772));
#79108=CARTESIAN_POINT('Ctrl Pts',(0.13024551285702,-0.0854261765480031,
-0.690590735168407));
#79109=CARTESIAN_POINT('Ctrl Pts',(0.134519313446427,-0.078524154440994,
-0.689974499134471));
#79110=CARTESIAN_POINT('Ctrl Pts',(0.142386524940968,-0.0632759399475228,
-0.688650589229111));
#79111=CARTESIAN_POINT('Ctrl Pts',(0.14582736188566,-0.054883112506267,
-0.687942984071129));
#79112=CARTESIAN_POINT('Ctrl Pts',(0.149371571018636,-0.0434990583616816,
-0.687039115483485));
#79113=CARTESIAN_POINT('Ctrl Pts',(0.150148550342963,-0.0407363439128798,
-0.686824020709226));
#79114=CARTESIAN_POINT('Ctrl Pts',(0.151094810050685,-0.0369753728078855,
-0.68653825692992));
#79115=CARTESIAN_POINT('Ctrl Pts',(0.151331398607144,-0.0359948295965663,
-0.686464394777725));
#79116=CARTESIAN_POINT('Ctrl Pts',(0.1516928580781,-0.0344301602855888,
-0.68634762258654));
#79117=CARTESIAN_POINT('Ctrl Pts',(0.151823926665111,-0.0338475176866469,
-0.686304379269762));
#79118=CARTESIAN_POINT('Ctrl Pts',(0.152094641011558,-0.0326108853392737,
-0.686213125168673));
#79119=CARTESIAN_POINT('Ctrl Pts',(0.152233431733234,-0.031956720221502,
-0.686165165485197));
#79120=CARTESIAN_POINT('Ctrl Pts',(0.152576706513767,-0.0302857519195269,
-0.686043408601166));
#79121=CARTESIAN_POINT('Ctrl Pts',(0.152775252392319,-0.0292677390666102,
-0.685969935264158));
#79122=CARTESIAN_POINT('Ctrl Pts',(0.153577288613936,-0.0249246596223963,
-0.685659179920169));
#79123=CARTESIAN_POINT('Ctrl Pts',(0.15408256936247,-0.021582124176489,
-0.685426725433824));
#79124=CARTESIAN_POINT('Ctrl Pts',(0.15526350892157,-0.0115725283598531,
-0.684743383860581));
#79125=CARTESIAN_POINT('Ctrl Pts',(0.155617879627099,-0.00487532178759307,
-0.684302714685869));
#79126=CARTESIAN_POINT('Ctrl Pts',(0.155423827038618,0.0116698071832762,
-0.683212862552858));
#79127=CARTESIAN_POINT('Ctrl Pts',(0.154373856334072,0.021480989589612,
-0.682564274530648));
#79128=CARTESIAN_POINT('Ctrl Pts',(0.151971952110645,0.0332413467680238,
-0.681738078002183));
#79129=CARTESIAN_POINT('Ctrl Pts',(0.151496082440588,0.0353468187923684,
-0.681588294671204));
#79130=CARTESIAN_POINT('Ctrl Pts',(0.15064308674465,0.0387863696871938,
-0.681340122326159));
#79131=CARTESIAN_POINT('Ctrl Pts',(0.150291653241152,0.0401265598385105,
-0.681242546870685));
#79132=CARTESIAN_POINT('Ctrl Pts',(0.149622452714608,0.0425463302414749,
-0.681064681269375));
#79133=CARTESIAN_POINT('Ctrl Pts',(0.149310779876542,0.0436275081232486,
-0.680984592260407));
#79134=CARTESIAN_POINT('Ctrl Pts',(0.148611042109735,0.0459594998364188,
-0.680810460322217));
#79135=CARTESIAN_POINT('Ctrl Pts',(0.148218857986491,0.0472089759043598,
-0.68071628885366));
#79136=CARTESIAN_POINT('Ctrl Pts',(0.14707077305594,0.050711306430118,-0.680449779850171));
#79137=CARTESIAN_POINT('Ctrl Pts',(0.146278987571426,0.0529519172039678,
-0.680276288879838));
#79138=CARTESIAN_POINT('Ctrl Pts',(0.142542109101753,0.0628022705402446,
-0.679499772072352));
#79139=CARTESIAN_POINT('Ctrl Pts',(0.139052670189038,0.0701904238856169,
-0.678879375835245));
#79140=CARTESIAN_POINT('Ctrl Pts',(0.130450778171729,0.0852190527600437,
-0.677543024598288));
#79141=CARTESIAN_POINT('Ctrl Pts',(0.125207673137088,0.092750961464185,
-0.676827087688327));
#79142=CARTESIAN_POINT('Ctrl Pts',(0.117576555293586,0.101877607908888,
-0.675926408963144));
#79143=CARTESIAN_POINT('Ctrl Pts',(0.115765689306785,0.103930750023422,
-0.675721458039828));
#79144=CARTESIAN_POINT('Ctrl Pts',(0.113226325296756,0.106661072918307,
-0.675446835871534));
#79145=CARTESIAN_POINT('Ctrl Pts',(0.112544252705924,0.107380522143752,
-0.675374268366817));
#79146=CARTESIAN_POINT('Ctrl Pts',(0.111442515048659,0.108520602799092,
-0.675259014619525));
#79147=CARTESIAN_POINT('Ctrl Pts',(0.111027251853162,0.108945421060729,
-0.675216009940731));
#79148=CARTESIAN_POINT('Ctrl Pts',(0.110136438899788,0.109846347764342,
-0.675124702884842));
#79149=CARTESIAN_POINT('Ctrl Pts',(0.109660210500655,0.110321772865897,
-0.675076455859219));
#79150=CARTESIAN_POINT('Ctrl Pts',(0.108428117954813,0.111535925678154,
-0.674953027409561));
#79151=CARTESIAN_POINT('Ctrl Pts',(0.107667767571077,0.112270082695363,
-0.674878187746555));
#79152=CARTESIAN_POINT('Ctrl Pts',(0.105408197655482,0.114407742129455,
-0.674659442644647));
#79153=CARTESIAN_POINT('Ctrl Pts',(0.103888656900956,0.115789318258862,
-0.674516986467108));
#79154=CARTESIAN_POINT('Ctrl Pts',(0.102342242758987,0.117140376672865,
-0.674376033428004));
#79155=CARTESIAN_POINT('Origin',(0.,0.,-1.10400562256037));
#79156=CARTESIAN_POINT('',(0.10234224283772,0.117140376604078,-0.590700225539723));
#79157=CARTESIAN_POINT('',(0.102342242827937,0.117140376612625,-0.604616163143584));
#79158=CARTESIAN_POINT('',(0.10234224283772,0.117140376604078,-1.10400562256037));
#79159=CARTESIAN_POINT('',(-0.15554994586618,-0.000129772988789563,-0.635194377433095));
#79160=CARTESIAN_POINT('Ctrl Pts',(-0.15554994586618,-0.000129772988788979,
-0.635194377433095));
#79161=CARTESIAN_POINT('Ctrl Pts',(-0.155539597239793,-0.0125339588620959,
-0.634307833869035));
#79162=CARTESIAN_POINT('Ctrl Pts',(-0.154041489336815,-0.0248731108772741,
-0.633421290304974));
#79163=CARTESIAN_POINT('Ctrl Pts',(-0.151125138991674,-0.0368374112112568,
-0.632534746740914));
#79164=CARTESIAN_POINT('Ctrl Pts',(-0.150339236238879,-0.0400615699901928,
-0.632295839564131));
#79165=CARTESIAN_POINT('Ctrl Pts',(-0.149450609198663,-0.0432586255057535,
-0.632056932387348));
#79166=CARTESIAN_POINT('Ctrl Pts',(-0.148461201799215,-0.0464227752329896,
-0.631818025210565));
#79167=CARTESIAN_POINT('Ctrl Pts',(-0.14540665540244,-0.0561912913706129,
-0.631080459414702));
#79168=CARTESIAN_POINT('Ctrl Pts',(-0.141372495840606,-0.0656933397014203,
-0.630342893618839));
#79169=CARTESIAN_POINT('Ctrl Pts',(-0.13642680457351,-0.0747230185007366,
-0.629605327822976));
#79170=CARTESIAN_POINT('Ctrl Pts',(-0.131469356563795,-0.0837741623701181,
-0.628866008708768));
#79171=CARTESIAN_POINT('Ctrl Pts',(-0.125596353745635,-0.0923498038083296,
-0.628126689594561));
#79172=CARTESIAN_POINT('Ctrl Pts',(-0.118924876618117,-0.100263035169327,
-0.627387370480353));
#79173=CARTESIAN_POINT('Ctrl Pts',(-0.112284413661745,-0.108139479727783,
-0.626651488291597));
#79174=CARTESIAN_POINT('Ctrl Pts',(-0.104853482495447,-0.115358944218995,
-0.625915606102841));
#79175=CARTESIAN_POINT('Ctrl Pts',(-0.0967885641346958,-0.121769357199354,
-0.625179723914085));
#79176=CARTESIAN_POINT('Ctrl Pts',(-0.0886671451745217,-0.128224679769585,
-0.624438686337151));
#79177=CARTESIAN_POINT('Ctrl Pts',(-0.0799035567255813,-0.133858969506248,
-0.623697648760218));
#79178=CARTESIAN_POINT('Ctrl Pts',(-0.0706893423499887,-0.138559804337788,
-0.622956611183284));
#79179=CARTESIAN_POINT('Ctrl Pts',(-0.0614751279743957,-0.143260639169328,
-0.622215573606351));
#79180=CARTESIAN_POINT('Ctrl Pts',(-0.0518111869380719,-0.147027705085406,
-0.621474536029418));
#79181=CARTESIAN_POINT('Ctrl Pts',(-0.0419083040406783,-0.149798186078584,
-0.620733498452484));
#79182=CARTESIAN_POINT('Ctrl Pts',(-0.0320518164171601,-0.152555687293471,
-0.619995932656616));
#79183=CARTESIAN_POINT('Ctrl Pts',(-0.0218853754879639,-0.154346453801442,
-0.619258366860748));
#79184=CARTESIAN_POINT('Ctrl Pts',(-0.01161875068525,-0.155115463872929,
-0.618520801064879));
#79185=CARTESIAN_POINT('Ctrl Pts',(-0.00132772038320625,-0.155886302011103,
-0.617781481950673));
#79186=CARTESIAN_POINT('Ctrl Pts',(0.0090630569164229,-0.155630303401892,
-0.617042162836467));
#79187=CARTESIAN_POINT('Ctrl Pts',(0.0193330602770041,-0.154343886436508,
-0.616302843722261));
#79188=CARTESIAN_POINT('Ctrl Pts',(0.0295553207411928,-0.153063449729333,
-0.615566961533499));
#79189=CARTESIAN_POINT('Ctrl Pts',(0.0396570018576745,-0.150762266520526,
-0.614831079344738));
#79190=CARTESIAN_POINT('Ctrl Pts',(0.0494253453003874,-0.147488771579187,
-0.614095197155977));
#79191=CARTESIAN_POINT('Ctrl Pts',(0.0592621230699126,-0.144192343432852,
-0.613354159579048));
#79192=CARTESIAN_POINT('Ctrl Pts',(0.0687599697457468,-0.13991021640765,
-0.612613122002119));
#79193=CARTESIAN_POINT('Ctrl Pts',(0.0777202887948234,-0.134741824277576,
-0.611872084425191));
#79194=CARTESIAN_POINT('Ctrl Pts',(0.0866806078439001,-0.129573432147503,
-0.611131046848262));
#79195=CARTESIAN_POINT('Ctrl Pts',(0.0951026462021396,-0.123519358158803,
-0.610390009271333));
#79196=CARTESIAN_POINT('Ctrl Pts',(0.102818935575983,-0.116722187209724,
-0.609648971694404));
#79197=CARTESIAN_POINT('Ctrl Pts',(0.110499073925748,-0.109956861190085,
-0.608911405898533));
#79198=CARTESIAN_POINT('Ctrl Pts',(0.117537168754883,-0.10240513376983,
-0.608173840102662));
#79199=CARTESIAN_POINT('Ctrl Pts',(0.123772841973527,-0.0942129825968604,
-0.607436274306792));
#79200=CARTESIAN_POINT('Ctrl Pts',(0.13002333843946,-0.0860013572984187,
-0.606696955192586));
#79201=CARTESIAN_POINT('Ctrl Pts',(0.13546691439087,-0.0771469081885431,
-0.60595763607838));
#79202=CARTESIAN_POINT('Ctrl Pts',(0.139980481331036,-0.0678326421889309,
-0.605218316964175));
#79203=CARTESIAN_POINT('Ctrl Pts',(0.144473065730982,-0.0585616760812977,
-0.604482434775411));
#79204=CARTESIAN_POINT('Ctrl Pts',(0.148043859148208,-0.0488359966751181,
-0.603746552586647));
#79205=CARTESIAN_POINT('Ctrl Pts',(0.150617627849007,-0.0388604256427797,
-0.603010670397883));
#79206=CARTESIAN_POINT('Ctrl Pts',(0.153209427665242,-0.0288149685042174,
-0.602269632820956));
#79207=CARTESIAN_POINT('Ctrl Pts',(0.15478992868617,-0.0185170211427482,
-0.60152859524403));
#79208=CARTESIAN_POINT('Ctrl Pts',(0.155334383310592,-0.00818729879253237,
-0.600787557667103));
#79209=CARTESIAN_POINT('Ctrl Pts',(0.155878837935013,0.00214242355768306,
-0.600046520090177));
#79210=CARTESIAN_POINT('Ctrl Pts',(0.155387325267977,0.0125029716737622,
-0.599305482513251));
#79211=CARTESIAN_POINT('Ctrl Pts',(0.153888240661186,0.0226762405659494,
-0.598564444936324));
#79212=CARTESIAN_POINT('Ctrl Pts',(0.152396068484794,0.0328025994886629,
-0.597826824358445));
#79213=CARTESIAN_POINT('Ctrl Pts',(0.149894543880813,0.0428186757317106,
-0.597089203780566));
#79214=CARTESIAN_POINT('Ctrl Pts',(0.1464187785058,0.0525104161178468,-0.596351583202687));
#79215=CARTESIAN_POINT('Ctrl Pts',(0.142950456108193,0.0621814026852035,
-0.595615542159875));
#79216=CARTESIAN_POINT('Ctrl Pts',(0.138512269623156,0.0715285415126396,
-0.594879501117063));
#79217=CARTESIAN_POINT('Ctrl Pts',(0.133189436101435,0.0803515812599966,
-0.594143460074251));
#79218=CARTESIAN_POINT('Ctrl Pts',(0.127867291225759,0.0891734795191949,
-0.593407514257366));
#79219=CARTESIAN_POINT('Ctrl Pts',(0.121661170840324,0.0974706005783878,
-0.59267156844048));
#79220=CARTESIAN_POINT('Ctrl Pts',(0.11470174867881,0.105068127184333,-0.591935622623595));
#79221=CARTESIAN_POINT('Ctrl Pts',(0.110807598843997,0.109319328834541,
-0.591523823595638));
#79222=CARTESIAN_POINT('Ctrl Pts',(0.106678376741718,0.113352018722323,
-0.59111202456768));
#79223=CARTESIAN_POINT('Ctrl Pts',(0.10234224283772,0.117140376604078,-0.590700225539723));
#79224=CARTESIAN_POINT('Ctrl Pts',(0.102342242837719,0.117140376604078,
-0.660690965868517));
#79225=CARTESIAN_POINT('Ctrl Pts',(0.0945841693280625,0.123918386595985,
-0.659955076078148));
#79226=CARTESIAN_POINT('Ctrl Pts',(0.0861441868282826,0.129927390680792,
-0.659219186287779));
#79227=CARTESIAN_POINT('Ctrl Pts',(0.0771999187120617,0.135040642218745,
-0.658483296497409));
#79228=CARTESIAN_POINT('Ctrl Pts',(0.0680918118152083,0.140247556970519,
-0.657733926868962));
#79229=CARTESIAN_POINT('Ctrl Pts',(0.0584615751935578,0.144525004141135,
-0.656984557240514));
#79230=CARTESIAN_POINT('Ctrl Pts',(0.0485226794565229,0.147788200064686,
-0.656235187612067));
#79231=CARTESIAN_POINT('Ctrl Pts',(0.0385837837194877,0.151051395988236,
-0.655485817983619));
#79232=CARTESIAN_POINT('Ctrl Pts',(0.0283372194356101,0.153300157887608,
-0.654736448355172));
#79233=CARTESIAN_POINT('Ctrl Pts',(0.0180083972417708,0.154504045671246,
-0.653987078726724));
#79234=CARTESIAN_POINT('Ctrl Pts',(0.00784227137744584,0.155688970196551,
-0.653249512930864));
#79235=CARTESIAN_POINT('Ctrl Pts',(-0.00247908354990559,0.155870624577179,
-0.652511947135003));
#79236=CARTESIAN_POINT('Ctrl Pts',(-0.0127398803529513,0.155027410313765,
-0.651774381339143));
#79237=CARTESIAN_POINT('Ctrl Pts',(-0.0230250688013239,0.154182191587769,
-0.651035062224935));
#79238=CARTESIAN_POINT('Ctrl Pts',(-0.0332484744830392,0.152307154402499,
-0.650295743110727));
#79239=CARTESIAN_POINT('Ctrl Pts',(-0.0431917212150337,0.149433188142671,
-0.649556423996518));
#79240=CARTESIAN_POINT('Ctrl Pts',(-0.0530887440673171,0.146572582294614,
-0.648820541807766));
#79241=CARTESIAN_POINT('Ctrl Pts',(-0.0627073101166465,0.142722570256699,
-0.648084659619013));
#79242=CARTESIAN_POINT('Ctrl Pts',(-0.071844831253178,0.137964208120086,
-0.64734877743026));
#79243=CARTESIAN_POINT('Ctrl Pts',(-0.0810463673491841,0.133172510207304,
-0.646607739853325));
#79244=CARTESIAN_POINT('Ctrl Pts',(-0.0897592437340419,0.127460112423326,
-0.645866702276389));
#79245=CARTESIAN_POINT('Ctrl Pts',(-0.0978028222610833,0.120956233645757,
-0.645125664699453));
#79246=CARTESIAN_POINT('Ctrl Pts',(-0.105846400788125,0.114452354868188,
-0.644384627122517));
#79247=CARTESIAN_POINT('Ctrl Pts',(-0.113220028681602,0.107157688757977,
-0.643643589545581));
#79248=CARTESIAN_POINT('Ctrl Pts',(-0.119780550983552,0.0992392165732715,
-0.642902551968645));
#79249=CARTESIAN_POINT('Ctrl Pts',(-0.126276902004641,0.0913981983593276,
-0.642168762797902));
#79250=CARTESIAN_POINT('Ctrl Pts',(-0.132025858922605,0.0828853067841873,
-0.641434973627158));
#79251=CARTESIAN_POINT('Ctrl Pts',(-0.136891903116717,0.0738675122166936,
-0.640701184456415));
#79252=CARTESIAN_POINT('Ctrl Pts',(-0.141747285352497,0.0648694764812375,
-0.639969003086433));
#79253=CARTESIAN_POINT('Ctrl Pts',(-0.145723079744574,0.0553695093407535,
-0.639236821716451));
#79254=CARTESIAN_POINT('Ctrl Pts',(-0.148727361559918,0.0455628623269607,
-0.638504640346469));
#79255=CARTESIAN_POINT('Ctrl Pts',(-0.151731044320082,0.0357581707631058,
-0.637772604973791));
#79256=CARTESIAN_POINT('Ctrl Pts',(-0.153763287048736,0.0256478034881993,
-0.637040569601112));
#79257=CARTESIAN_POINT('Ctrl Pts',(-0.15478141922985,0.0154439231153664,
-0.636308534228433));
#79258=CARTESIAN_POINT('Ctrl Pts',(-0.155297951137016,0.0102671593441833,
-0.635937148632165));
#79259=CARTESIAN_POINT('Ctrl Pts',(-0.155554281048676,0.00506651542239916,
-0.635565763035898));
#79260=CARTESIAN_POINT('Ctrl Pts',(-0.155549945866256,-0.000129772897362374,
-0.63519437743963));
#79261=CARTESIAN_POINT('',(-0.155549974362134,8.93081152335447E-5,-0.649113732242943));
#79262=CARTESIAN_POINT('Ctrl Pts',(0.102342242758987,0.117140376672865,
-0.674376033428004));
#79263=CARTESIAN_POINT('Ctrl Pts',(0.101191146679549,0.118146056846915,
-0.674271112963107));
#79264=CARTESIAN_POINT('Ctrl Pts',(0.100025160633051,0.119134827817089,
-0.674167025422502));
#79265=CARTESIAN_POINT('Ctrl Pts',(0.0930757671449147,0.124854012298398,
-0.673558102406125));
#79266=CARTESIAN_POINT('Ctrl Pts',(0.0869719332770196,0.129180186700844,
-0.673068760632657));
#79267=CARTESIAN_POINT('Ctrl Pts',(0.0730551137837119,0.137608702257919,
-0.671996546687483));
#79268=CARTESIAN_POINT('Ctrl Pts',(0.0651575809181942,0.141519146308847,
-0.671413937645293));
#79269=CARTESIAN_POINT('Ctrl Pts',(0.0549485145970029,0.145537603928452,
-0.670658934752614));
#79270=CARTESIAN_POINT('Ctrl Pts',(0.0529081943963351,0.146291679847769,
-0.67050802655823));
#79271=CARTESIAN_POINT('Ctrl Pts',(0.0495389084353664,0.147457220899202,
-0.67025838283206));
#79272=CARTESIAN_POINT('Ctrl Pts',(0.0482190047314951,0.147894093207751,
-0.670160477969575));
#79273=CARTESIAN_POINT('Ctrl Pts',(0.0458203554904981,0.148652494745097,
-0.669982266902835));
#79274=CARTESIAN_POINT('Ctrl Pts',(0.0447436272982595,0.148980122386781,
-0.669902165658211));
#79275=CARTESIAN_POINT('Ctrl Pts',(0.0424101767448871,0.149662568761497,
-0.669728299214583));
#79276=CARTESIAN_POINT('Ctrl Pts',(0.0411523602496633,0.150013301523527,
-0.669634408596997));
#79277=CARTESIAN_POINT('Ctrl Pts',(0.0376115687397058,0.150952742944754,
-0.669369549457639));
#79278=CARTESIAN_POINT('Ctrl Pts',(0.0353194967195086,0.151505421476829,
-0.669197450384273));
#79279=CARTESIAN_POINT('Ctrl Pts',(0.0251858815772117,0.15370645654733,
-0.668433319164996));
#79280=CARTESIAN_POINT('Ctrl Pts',(0.0172373973561568,0.154799353730613,
-0.66782456991791));
#79281=CARTESIAN_POINT('Ctrl Pts',(0.000392267604439727,0.15580189340765,
-0.666522944935293));
#79282=CARTESIAN_POINT('Ctrl Pts',(-0.008485581668265,0.155571157436399,
-0.665830232916812));
#79283=CARTESIAN_POINT('Ctrl Pts',(-0.0203867252573994,0.154239614684418,
-0.66492033771237));
#79284=CARTESIAN_POINT('Ctrl Pts',(-0.0234670678594841,0.153801096306821,
-0.664686682487581));
#79285=CARTESIAN_POINT('Ctrl Pts',(-0.0275554599292424,0.153093360696824,
-0.664380717088592));
#79286=CARTESIAN_POINT('Ctrl Pts',(-0.0285767324465484,0.152906020090096,
-0.66430463731119));
#79287=CARTESIAN_POINT('Ctrl Pts',(-0.0301878069677704,0.152593781302567,
-0.664185252924315));
#79288=CARTESIAN_POINT('Ctrl Pts',(-0.0307788671257554,0.152475660855673,
-0.664141589164485));
#79289=CARTESIAN_POINT('Ctrl Pts',(-0.032018106000498,0.152220505403247,
-0.664050347060237));
#79290=CARTESIAN_POINT('Ctrl Pts',(-0.0326661224021602,0.152082759880494,
-0.664002812867636));
#79291=CARTESIAN_POINT('Ctrl Pts',(-0.0342968378213496,0.151725223235351,
-0.663883597824645));
#79292=CARTESIAN_POINT('Ctrl Pts',(-0.0352783423295761,0.151500017010828,
-0.663812214000121));
#79293=CARTESIAN_POINT('Ctrl Pts',(-0.0392668640684486,0.150543985878361,
-0.663523382118335));
#79294=CARTESIAN_POINT('Ctrl Pts',(-0.0422541634248812,0.149732986187034,
-0.663309953831452));
#79295=CARTESIAN_POINT('Ctrl Pts',(-0.050709472318709,0.147164266272489,
-0.662708948812627));
#79296=CARTESIAN_POINT('Ctrl Pts',(-0.0561072127042601,0.145192155724305,
-0.662328927186861));
#79297=CARTESIAN_POINT('Ctrl Pts',(-0.0717400525541236,0.138478159013006,
-0.661207040752277));
#79298=CARTESIAN_POINT('Ctrl Pts',(-0.0815809885868729,0.132918564187561,
-0.660469954097329));
#79299=CARTESIAN_POINT('Ctrl Pts',(-0.0926031280196733,0.125003022254412,
-0.659535073818111));
#79300=CARTESIAN_POINT('Ctrl Pts',(-0.0944416294060303,0.123619871327327,
-0.659375195560815));
#79301=CARTESIAN_POINT('Ctrl Pts',(-0.0972757672319868,0.121387548376986,
-0.659122002252391));
#79302=CARTESIAN_POINT('Ctrl Pts',(-0.0982925610520427,0.120565683542686,
-0.659029755389586));
#79303=CARTESIAN_POINT('Ctrl Pts',(-0.100111459381183,0.119057182614937,
-0.658862089527016));
#79304=CARTESIAN_POINT('Ctrl Pts',(-0.100917170555288,0.118375004196761,
-0.658786853466611));
#79305=CARTESIAN_POINT('Ctrl Pts',(-0.101832265207055,0.117584080284343,
-0.658700266580737));
#79306=CARTESIAN_POINT('Ctrl Pts',(-0.101948523075608,0.117483295901606,
-0.658689244925735));
#79307=CARTESIAN_POINT('Ctrl Pts',(-0.102109658066315,0.117343188084639,
-0.658673939155643));
#79308=CARTESIAN_POINT('Ctrl Pts',(-0.102154662707767,0.117304010789618,
-0.658669661075927));
#79309=CARTESIAN_POINT('Ctrl Pts',(-0.102221014918879,0.117246182933686,
-0.658663348980168));
#79310=CARTESIAN_POINT('Ctrl Pts',(-0.102242379994868,0.117227552378049,
-0.658661315790858));
#79311=CARTESIAN_POINT('Ctrl Pts',(-0.10233817386207,0.117143973078278,
-0.658652196388826));
#79312=CARTESIAN_POINT('Ctrl Pts',(-0.102412545721494,0.117078959410936,
-0.658645107493641));
#79313=CARTESIAN_POINT('Ctrl Pts',(-0.102555142941754,0.116954065327314,
-0.658631498586842));
#79314=CARTESIAN_POINT('Ctrl Pts',(-0.102623377938085,0.116894195924784,
-0.658624979033036));
#79315=CARTESIAN_POINT('Ctrl Pts',(-0.102755691774694,0.116777898585883,
-0.658612322483519));
#79316=CARTESIAN_POINT('Ctrl Pts',(-0.102819776654293,0.116721477539218,
-0.658606185774921));
#79317=CARTESIAN_POINT('Ctrl Pts',(-0.102945281708731,0.116610797914942,
-0.658594154497396));
#79318=CARTESIAN_POINT('Ctrl Pts',(-0.103006705531186,0.116556543497196,
-0.658588260102407));
#79319=CARTESIAN_POINT('Ctrl Pts',(-0.10312807706735,0.116449167605556,
-0.658576600821216));
#79320=CARTESIAN_POINT('Ctrl Pts',(-0.103188026688685,0.116396048316458,
-0.658570836026945));
#79321=CARTESIAN_POINT('Ctrl Pts',(-0.103307457246567,0.116290060238851,
-0.658559339784915));
#79322=CARTESIAN_POINT('Ctrl Pts',(-0.103366938694209,0.116237192060248,
-0.658553608363612));
#79323=CARTESIAN_POINT('Ctrl Pts',(-0.103486340718961,0.116130901266918,
-0.658542091519896));
#79324=CARTESIAN_POINT('Ctrl Pts',(-0.103546260561809,0.116077477867538,
-0.658536306065882));
#79325=CARTESIAN_POINT('Ctrl Pts',(-0.103667407098685,0.115969297456227,
-0.658524596969065));
#79326=CARTESIAN_POINT('Ctrl Pts',(-0.103728631824934,0.115914538288926,
-0.65851867323754));
#79327=CARTESIAN_POINT('Ctrl Pts',(-0.103853263511517,0.115802890355983,
-0.658506601945836));
#79328=CARTESIAN_POINT('Ctrl Pts',(-0.103916667162697,0.115745997954731,
-0.658500454235187));
#79329=CARTESIAN_POINT('Ctrl Pts',(-0.105506390801845,0.114317172176548,
-0.658346143786108));
#79330=CARTESIAN_POINT('Ctrl Pts',(-0.107005387180538,0.112915281193089,
-0.658196734748946));
#79331=CARTESIAN_POINT('Ctrl Pts',(-0.110296800040051,0.109712676984326,
-0.657859612855542));
#79332=CARTESIAN_POINT('Ctrl Pts',(-0.112073683441505,0.107896912522107,
-0.657671291284155));
#79333=CARTESIAN_POINT('Ctrl Pts',(-0.11762458060116,0.101939446039894,
-0.657062122102572));
#79334=CARTESIAN_POINT('Ctrl Pts',(-0.12121931945391,0.0976373808579105,
-0.656634953057946));
#79335=CARTESIAN_POINT('Ctrl Pts',(-0.129548842673277,0.0864980587898974,
-0.655563254996515));
#79336=CARTESIAN_POINT('Ctrl Pts',(-0.133982769905782,0.0794571283625117,
-0.654914572160442));
#79337=CARTESIAN_POINT('Ctrl Pts',(-0.13962530764626,0.0686696853378198,
-0.653984048898601));
#79338=CARTESIAN_POINT('Ctrl Pts',(-0.141289192072979,0.065177619195162,
-0.653691947808538));
#79339=CARTESIAN_POINT('Ctrl Pts',(-0.143262478660383,0.0606044928527206,
-0.65332399864148));
#79340=CARTESIAN_POINT('Ctrl Pts',(-0.143692652832446,0.0595773787399836,
-0.65324228330971));
#79341=CARTESIAN_POINT('Ctrl Pts',(-0.144369644865931,0.0579109449523117,
-0.653111291884689));
#79342=CARTESIAN_POINT('Ctrl Pts',(-0.144623323584781,0.0572744814716124,
-0.653061632451789));
#79343=CARTESIAN_POINT('Ctrl Pts',(-0.145114513979685,0.0560180422748632,
-0.652964356018714));
#79344=CARTESIAN_POINT('Ctrl Pts',(-0.145352275943719,0.0553981871207527,
-0.652916726655579));
#79345=CARTESIAN_POINT('Ctrl Pts',(-0.145943082203899,0.0538279396423758,
-0.652796934779546));
#79346=CARTESIAN_POINT('Ctrl Pts',(-0.146290825206794,0.0528755608367879,
-0.652725075346112));
#79347=CARTESIAN_POINT('Ctrl Pts',(-0.147682944950127,0.0489440087403064,
-0.652431423930231));
#79348=CARTESIAN_POINT('Ctrl Pts',(-0.148645902061094,0.0459365581875476,
-0.652213822481557));
#79349=CARTESIAN_POINT('Ctrl Pts',(-0.153510914817863,0.0289814762591141,
-0.651015006652198));
#79350=CARTESIAN_POINT('Ctrl Pts',(-0.155541659225333,0.0145719708928448,
-0.65009394675668));
#79351=CARTESIAN_POINT('Ctrl Pts',(-0.155549974362134,8.93081152335447E-5,
-0.649113732242943));
#79352=CARTESIAN_POINT('Ctrl Pts',(-0.155549974470581,8.91190302388376E-5,
-0.649113719445304));
#79353=CARTESIAN_POINT('Ctrl Pts',(-0.155551459251949,-0.00250244534429518,
-0.648938317303811));
#79354=CARTESIAN_POINT('Ctrl Pts',(-0.155488178294614,-0.0050935523913905,
-0.648761442142846));
#79355=CARTESIAN_POINT('Ctrl Pts',(-0.15526486225176,-0.00961000152068747,
-0.648449601131202));
#79356=CARTESIAN_POINT('Ctrl Pts',(-0.155133636844657,-0.0115361927770886,
-0.648315482084797));
#79357=CARTESIAN_POINT('Ctrl Pts',(-0.154869829583466,-0.0145735789585794,
-0.648101942028573));
#79358=CARTESIAN_POINT('Ctrl Pts',(-0.154761045520123,-0.0156866820434499,
-0.648023251010666));
#79359=CARTESIAN_POINT('Ctrl Pts',(-0.154524027502421,-0.0178685763627349,
-0.647868091716286));
#79360=CARTESIAN_POINT('Ctrl Pts',(-0.154396683232695,-0.0189374020972839,
-0.647791655193124));
#79361=CARTESIAN_POINT('Ctrl Pts',(-0.154102257738286,-0.0212077358565061,
-0.647628333460605));
#79362=CARTESIAN_POINT('Ctrl Pts',(-0.153932194339202,-0.0224087771374998,
-0.647541359647675));
#79363=CARTESIAN_POINT('Ctrl Pts',(-0.153458170911275,-0.0254959172861875,
-0.647316260655064));
#79364=CARTESIAN_POINT('Ctrl Pts',(-0.153133487550905,-0.0273785757199024,
-0.647177495841913));
#79365=CARTESIAN_POINT('Ctrl Pts',(-0.15148296628841,-0.0359979460366745,
-0.646535030361311));
#79366=CARTESIAN_POINT('Ctrl Pts',(-0.149746862360095,-0.0426473206902234,
-0.646018716962129));
#79367=CARTESIAN_POINT('Ctrl Pts',(-0.144312107398187,-0.058962539639381,
-0.64470210320504));
#79368=CARTESIAN_POINT('Ctrl Pts',(-0.140078185731863,-0.0684153254219521,
-0.64389211107294));
#79369=CARTESIAN_POINT('Ctrl Pts',(-0.133156074428233,-0.0804866501165299,
-0.642831117833079));
#79370=CARTESIAN_POINT('Ctrl Pts',(-0.131266632263183,-0.0835327296734139,
-0.642561128678344));
#79371=CARTESIAN_POINT('Ctrl Pts',(-0.128685650421676,-0.0873894904439736,
-0.642218760198617));
#79372=CARTESIAN_POINT('Ctrl Pts',(-0.128088849172488,-0.0882619201353838,
-0.642141279424662));
#79373=CARTESIAN_POINT('Ctrl Pts',(-0.127097607787183,-0.0896797268575393,
-0.642015393009744));
#79374=CARTESIAN_POINT('Ctrl Pts',(-0.126708451022431,-0.0902287304665876,
-0.641966654610755));
#79375=CARTESIAN_POINT('Ctrl Pts',(-0.125969069580601,-0.0912575963176893,
-0.641875355922972));
#79376=CARTESIAN_POINT('Ctrl Pts',(-0.125619637324001,-0.0917380080832283,
-0.641832742045428));
#79377=CARTESIAN_POINT('Ctrl Pts',(-0.124679801572681,-0.0930146878238521,
-0.641719506095405));
#79378=CARTESIAN_POINT('Ctrl Pts',(-0.124084512211861,-0.093807350648264,
-0.64164920991549));
#79379=CARTESIAN_POINT('Ctrl Pts',(-0.121817588251036,-0.0967665517765677,
-0.64138658344035));
#79380=CARTESIAN_POINT('Ctrl Pts',(-0.120096352535078,-0.0988946849955261,
-0.641197315738529));
#79381=CARTESIAN_POINT('Ctrl Pts',(-0.112374116134005,-0.107943259892743,
-0.640385261101784));
#79382=CARTESIAN_POINT('Ctrl Pts',(-0.10582425465258,-0.114371969822372,
-0.639788240768916));
#79383=CARTESIAN_POINT('Ctrl Pts',(-0.092441879549769,-0.125366956881615,
-0.638645681777124));
#79384=CARTESIAN_POINT('Ctrl Pts',(-0.085740558252307,-0.130041951416835,
-0.638103409703136));
#79385=CARTESIAN_POINT('Ctrl Pts',(-0.0766544227550917,-0.135371889386149,
-0.637378149651699));
#79386=CARTESIAN_POINT('Ctrl Pts',(-0.0745776265641524,-0.136527013981853,
-0.637213074924721));
#79387=CARTESIAN_POINT('Ctrl Pts',(-0.071316542888142,-0.138244233817961,
-0.636954433447759));
#79388=CARTESIAN_POINT('Ctrl Pts',(-0.0701501798635377,-0.138839726131943,
-0.636862038587155));
#79389=CARTESIAN_POINT('Ctrl Pts',(-0.0679679455006226,-0.139919358764587,
-0.636689296592742));
#79390=CARTESIAN_POINT('Ctrl Pts',(-0.066954063558749,-0.140407342487198,
-0.6366090893944));
#79391=CARTESIAN_POINT('Ctrl Pts',(-0.0646801518762896,-0.141471551896206,
-0.636429264155266));
#79392=CARTESIAN_POINT('Ctrl Pts',(-0.063417551680542,-0.142042021783284,
-0.636329456733153));
#79393=CARTESIAN_POINT('Ctrl Pts',(-0.0601688684370673,-0.143457898255239,
-0.636072675100242));
#79394=CARTESIAN_POINT('Ctrl Pts',(-0.0581725614188709,-0.144278943511313,
-0.63591490297013));
#79395=CARTESIAN_POINT('Ctrl Pts',(-0.0469785878072871,-0.148612740066354,
-0.635029941825449));
#79396=CARTESIAN_POINT('Ctrl Pts',(-0.0374820739757276,-0.151287033083471,
-0.634276050847694));
#79397=CARTESIAN_POINT('Ctrl Pts',(-0.0212056352631647,-0.154243379994563,
-0.632994961965968));
#79398=CARTESIAN_POINT('Ctrl Pts',(-0.014542268405264,-0.155013640728622,
-0.632474093920613));
#79399=CARTESIAN_POINT('Ctrl Pts',(-0.00447444041750365,-0.155522357958324,
-0.631706721570313));
#79400=CARTESIAN_POINT('Ctrl Pts',(-0.0010941409852425,-0.155582876009482,
-0.631452454292036));
#79401=CARTESIAN_POINT('Ctrl Pts',(0.00332277466916035,-0.155517964800422,
-0.631126720858724));
#79402=CARTESIAN_POINT('Ctrl Pts',(0.00435968517377682,-0.155492351926568,
-0.631050722395967));
#79403=CARTESIAN_POINT('Ctrl Pts',(0.00606460273096834,-0.155433169761592,
-0.630926619248101));
#79404=CARTESIAN_POINT('Ctrl Pts',(0.00673277000123357,-0.155405661189494,
-0.630878198849048));
#79405=CARTESIAN_POINT('Ctrl Pts',(0.0079972616151005,-0.155345430989557,
-0.630786999597896));
#79406=CARTESIAN_POINT('Ctrl Pts',(0.00859360916398867,-0.155313582910381,
-0.630744171762612));
#79407=CARTESIAN_POINT('Ctrl Pts',(0.0101966026689352,-0.1552187136034,
-0.630629505179566));
#79408=CARTESIAN_POINT('Ctrl Pts',(0.0112028652170258,-0.155149333584473,
-0.630558007685805));
#79409=CARTESIAN_POINT('Ctrl Pts',(0.0150684457240935,-0.154845002855718,
-0.630284959795451));
#79410=CARTESIAN_POINT('Ctrl Pts',(0.0179219250079935,-0.15454073942436,
-0.630086793148586));
#79411=CARTESIAN_POINT('Ctrl Pts',(0.0297375545020742,-0.152949133652808,
-0.629274254225004));
#79412=CARTESIAN_POINT('Ctrl Pts',(0.0385876831871622,-0.150959528372375,
-0.628684145181647));
#79413=CARTESIAN_POINT('Ctrl Pts',(0.0549392729532534,-0.145750459846946,
-0.62755191391849));
#79414=CARTESIAN_POINT('Ctrl Pts',(0.0624584030346325,-0.142690034231669,
-0.627012955238379));
#79415=CARTESIAN_POINT('Ctrl Pts',(0.0718226847182252,-0.137996084902389,
-0.626291705810336));
#79416=CARTESIAN_POINT('Ctrl Pts',(0.0739164034357701,-0.136886017425754,
-0.626127080638367));
#79417=CARTESIAN_POINT('Ctrl Pts',(0.0771253805785011,-0.135089561497619,
-0.625868988568626));
#79418=CARTESIAN_POINT('Ctrl Pts',(0.078258762798155,-0.13443615516184,
-0.625776685326374));
#79419=CARTESIAN_POINT('Ctrl Pts',(0.0803514556195962,-0.133194265480418,
-0.625604027226321));
#79420=CARTESIAN_POINT('Ctrl Pts',(0.0813128884728513,-0.13260951256942,
-0.625523811189525));
#79421=CARTESIAN_POINT('Ctrl Pts',(0.0834451585095739,-0.131280738420449,
-0.62534385225559));
#79422=CARTESIAN_POINT('Ctrl Pts',(0.0846125442178338,-0.130531390438542,
-0.625243918636892));
#79423=CARTESIAN_POINT('Ctrl Pts',(0.0875752582063992,-0.128573172861007,
-0.624986578062361));
#79424=CARTESIAN_POINT('Ctrl Pts',(0.0893556074004888,-0.127342299298565,
-0.624828367207782));
#79425=CARTESIAN_POINT('Ctrl Pts',(0.0987857444887335,-0.1205274829385,
-0.623970521423895));
#79426=CARTESIAN_POINT('Ctrl Pts',(0.105937948927599,-0.114291699787246,
-0.623246388771629));
#79427=CARTESIAN_POINT('Ctrl Pts',(0.117294928123706,-0.102402814555705,
-0.621973771851205));
#79428=CARTESIAN_POINT('Ctrl Pts',(0.121767641019183,-0.0970416665268637,
-0.621431172570384));
#79429=CARTESIAN_POINT('Ctrl Pts',(0.12789512220191,-0.0886034443560276,
-0.620636854616848));
#79430=CARTESIAN_POINT('Ctrl Pts',(0.129831164101717,-0.0857415051591593,
-0.620376844467932));
#79431=CARTESIAN_POINT('Ctrl Pts',(0.132226596468878,-0.0819330262774496,
-0.620045018648924));
#79432=CARTESIAN_POINT('Ctrl Pts',(0.132773836970716,-0.0810432105931554,
-0.619968466270191));
#79433=CARTESIAN_POINT('Ctrl Pts',(0.133657451309003,-0.0795734721546524,
-0.619843697371071));
#79434=CARTESIAN_POINT('Ctrl Pts',(0.133999104310011,-0.0789967838365404,
-0.619795158787579));
#79435=CARTESIAN_POINT('Ctrl Pts',(0.134637472493181,-0.0779032006465429,
-0.619703925990048));
#79436=CARTESIAN_POINT('Ctrl Pts',(0.134934962843697,-0.0773867786173892,
-0.619661181046791));
#79437=CARTESIAN_POINT('Ctrl Pts',(0.13572461285842,-0.0759976041322065,
-0.619547064480951));
#79438=CARTESIAN_POINT('Ctrl Pts',(0.136211331025798,-0.0751217665464271,
-0.619476028189553));
#79439=CARTESIAN_POINT('Ctrl Pts',(0.138034211728411,-0.0717655628918832,
-0.619207031457263));
#79440=CARTESIAN_POINT('Ctrl Pts',(0.139311452478313,-0.0692536012179142,
-0.619012327884833));
#79441=CARTESIAN_POINT('Ctrl Pts',(0.144419866941461,-0.0584927917705782,
-0.618199996887239));
#79442=CARTESIAN_POINT('Ctrl Pts',(0.147592273629558,-0.04995052663425,
-0.617607210752402));
#79443=CARTESIAN_POINT('Ctrl Pts',(0.152151716982168,-0.0333422605614492,
-0.616470976073304));
#79444=CARTESIAN_POINT('Ctrl Pts',(0.153685494673246,-0.02534951036745,
-0.615930731204967));
#79445=CARTESIAN_POINT('Ctrl Pts',(0.154851298654041,-0.0149166021801462,
-0.615207924904403));
#79446=CARTESIAN_POINT('Ctrl Pts',(0.155060757134233,-0.0125534968938902,
-0.615043124944915));
#79447=CARTESIAN_POINT('Ctrl Pts',(0.155301798614254,-0.00888069085844641,
-0.614784819258134));
#79448=CARTESIAN_POINT('Ctrl Pts',(0.15537101826593,-0.00757375865328602,
-0.614692480384588));
#79449=CARTESIAN_POINT('Ctrl Pts',(0.155469066251677,-0.00514180273128026,
-0.614519789692284));
#79450=CARTESIAN_POINT('Ctrl Pts',(0.155502193026476,-0.00401703113108116,
-0.61443957712816));
#79451=CARTESIAN_POINT('Ctrl Pts',(0.155548891444341,-0.00150575205152136,
-0.614259670362665));
#79452=CARTESIAN_POINT('Ctrl Pts',(0.155556132862643,-0.000119238764841339,
-0.614159785962396));
#79453=CARTESIAN_POINT('Ctrl Pts',(0.155527226552163,0.00342907291418397,
-0.613902663430653));
#79454=CARTESIAN_POINT('Ctrl Pts',(0.155464544200951,0.00559029285697034,
-0.61374462373537));
#79455=CARTESIAN_POINT('Ctrl Pts',(0.154876635500673,0.0173764369529321,
-0.612874569885442));
#79456=CARTESIAN_POINT('Ctrl Pts',(0.153502720513309,0.0269363891684311,
-0.612137081877608));
#79457=CARTESIAN_POINT('Ctrl Pts',(0.149654764192167,0.0429671871826022,
-0.610860707820909));
#79458=CARTESIAN_POINT('Ctrl Pts',(0.147617576798016,0.0495155091307251,
-0.610327938452325));
#79459=CARTESIAN_POINT('Ctrl Pts',(0.143925777929179,0.0591005442025626,
-0.60954578105697));
#79460=CARTESIAN_POINT('Ctrl Pts',(0.142591209242072,0.0622515466705997,
-0.609288341104641));
#79461=CARTESIAN_POINT('Ctrl Pts',(0.140716190379459,0.0663011351181469,
-0.608959239596094));
#79462=CARTESIAN_POINT('Ctrl Pts',(0.14026919316207,0.0672416564308969,
-0.608882933308951));
#79463=CARTESIAN_POINT('Ctrl Pts',(0.13951929437926,0.068779483312375,-0.608758460284638));
#79464=CARTESIAN_POINT('Ctrl Pts',(0.139221928508128,0.0693794314145882,
-0.608709974308017));
#79465=CARTESIAN_POINT('Ctrl Pts',(0.13865234277528,0.0705101847287545,
-0.608618756965748));
#79466=CARTESIAN_POINT('Ctrl Pts',(0.138380928248831,0.0710413755265428,
-0.608575975642808));
#79467=CARTESIAN_POINT('Ctrl Pts',(0.137644104688197,0.0724631816651877,
-0.60846161706615));
#79468=CARTESIAN_POINT('Ctrl Pts',(0.137173100200892,0.0733508893903533,
-0.608390377746996));
#79469=CARTESIAN_POINT('Ctrl Pts',(0.135338214724856,0.0767296232912663,
-0.608119605517211));
#79470=CARTESIAN_POINT('Ctrl Pts',(0.133914723007637,0.0791878584081466,
-0.607923384763523));
#79471=CARTESIAN_POINT('Ctrl Pts',(0.127047033176055,0.0903322845749481,
-0.607030912771506));
#79472=CARTESIAN_POINT('Ctrl Pts',(0.120819624200894,0.0985064803861634,
-0.606366581606531));
#79473=CARTESIAN_POINT('Ctrl Pts',(0.11030473340754,0.109797387405944,-0.605345710376678));
#79474=CARTESIAN_POINT('Ctrl Pts',(0.106590097086477,0.113406990932573,
-0.605000559159934));
#79475=CARTESIAN_POINT('Ctrl Pts',(0.102582667496328,0.116929997632619,
-0.604637895112637));
#79476=CARTESIAN_POINT('Ctrl Pts',(0.102462535204728,0.117035280556151,
-0.604627032087788));
#79477=CARTESIAN_POINT('Ctrl Pts',(0.102342242827937,0.117140376612625,
-0.604616163143584));
#79478=CARTESIAN_POINT('Origin',(0.,0.,-1.10400562256037));
#79479=CARTESIAN_POINT('',(0.10234224283772,0.117140376604078,-0.520692779095311));
#79480=CARTESIAN_POINT('',(0.102342237477092,0.117140381287507,-0.534570457414543));
#79481=CARTESIAN_POINT('',(0.10234224283772,0.117140376604078,-1.10400562256037));
#79482=CARTESIAN_POINT('',(-0.155549999681985,9.9465836413514E-6,-0.565194377435295));
#79483=CARTESIAN_POINT('Ctrl Pts',(-0.155549999681985,9.9465836413514E-6,
-0.565194377435295));
#79484=CARTESIAN_POINT('Ctrl Pts',(-0.155550652961944,-0.0102063951447715,
-0.564458166637774));
#79485=CARTESIAN_POINT('Ctrl Pts',(-0.154540483344138,-0.0204614277915781,
-0.563721955840253));
#79486=CARTESIAN_POINT('Ctrl Pts',(-0.152522697323478,-0.0305389800283305,
-0.562985745042732));
#79487=CARTESIAN_POINT('Ctrl Pts',(-0.150507519952113,-0.0406035037282293,
-0.56225048603879));
#79488=CARTESIAN_POINT('Ctrl Pts',(-0.147487397691107,-0.0504900784062613,
-0.561515227034848));
#79489=CARTESIAN_POINT('Ctrl Pts',(-0.143517271214654,-0.059988293550488,
-0.560779968030905));
#79490=CARTESIAN_POINT('Ctrl Pts',(-0.139551022262881,-0.0694772320220811,
-0.560045427136311));
#79491=CARTESIAN_POINT('Ctrl Pts',(-0.134636952228676,-0.0785776981356956,
-0.559310886241716));
#79492=CARTESIAN_POINT('Ctrl Pts',(-0.12887853867428,-0.0870983626090755,
-0.558576345347122));
#79493=CARTESIAN_POINT('Ctrl Pts',(-0.123105816881007,-0.0956401988342802,
-0.557839979299386));
#79494=CARTESIAN_POINT('Ctrl Pts',(-0.116485094228212,-0.103598584776286,
-0.557103613251651));
#79495=CARTESIAN_POINT('Ctrl Pts',(-0.109163042999335,-0.110811698584244,
-0.556367247203916));
#79496=CARTESIAN_POINT('Ctrl Pts',(-0.102067003550593,-0.117802163213564,
-0.555653610770612));
#79497=CARTESIAN_POINT('Ctrl Pts',(-0.0943130906390056,-0.124092347201511,
-0.554939974337308));
#79498=CARTESIAN_POINT('Ctrl Pts',(-0.0860640892451476,-0.12957150551878,
-0.554226337904004));
#79499=CARTESIAN_POINT('Ctrl Pts',(-0.0775384857385886,-0.13523438871304,
-0.553488772108135));
#79500=CARTESIAN_POINT('Ctrl Pts',(-0.0684198911666055,-0.140073252100748,
-0.552751206312266));
#79501=CARTESIAN_POINT('Ctrl Pts',(-0.0588908807238225,-0.143971061910276,
-0.552013640516397));
#79502=CARTESIAN_POINT('Ctrl Pts',(-0.0493392182155014,-0.147878137471352,
-0.551274321402191));
#79503=CARTESIAN_POINT('Ctrl Pts',(-0.0393759886201371,-0.150839192048426,
-0.550535002287985));
#79504=CARTESIAN_POINT('Ctrl Pts',(-0.0292098589783628,-0.152782808713756,
-0.549795683173779));
#79505=CARTESIAN_POINT('Ctrl Pts',(-0.0190909893478124,-0.154717389949807,
-0.549059800985017));
#79506=CARTESIAN_POINT('Ctrl Pts',(-0.00877201741954846,-0.155643793686536,
-0.548323918796255));
#79507=CARTESIAN_POINT('Ctrl Pts',(0.00152973184211935,-0.155542477865345,
-0.547588036607493));
#79508=CARTESIAN_POINT('Ctrl Pts',(0.0119036523250068,-0.155440452253383,
-0.546846999030565));
#79509=CARTESIAN_POINT('Ctrl Pts',(0.0222591580446818,-0.154296247452144,
-0.546105961453637));
#79510=CARTESIAN_POINT('Ctrl Pts',(0.0323766671306018,-0.152143202035169,
-0.545364923876708));
#79511=CARTESIAN_POINT('Ctrl Pts',(0.0424941762165218,-0.149990156618194,
-0.54462388629978));
#79512=CARTESIAN_POINT('Ctrl Pts',(0.0523727924363232,-0.146828593152129,
-0.543882848722852));
#79513=CARTESIAN_POINT('Ctrl Pts',(0.0618092367599878,-0.142742498055582,
-0.543141811145923));
#79514=CARTESIAN_POINT('Ctrl Pts',(0.0712014710871692,-0.138675546424905,
-0.542404245350054));
#79515=CARTESIAN_POINT('Ctrl Pts',(0.0802254889893704,-0.133662516726816,
-0.541666679554185));
#79516=CARTESIAN_POINT('Ctrl Pts',(0.0886837096846341,-0.127792809408713,
-0.540929113758316));
#79517=CARTESIAN_POINT('Ctrl Pts',(0.0971620369975398,-0.121909148805992,
-0.54018979464411));
#79518=CARTESIAN_POINT('Ctrl Pts',(0.105071027690536,-0.11516514002809,
-0.539450475529904));
#79519=CARTESIAN_POINT('Ctrl Pts',(0.112237152853552,-0.107696908123346,
-0.538711156415698));
#79520=CARTESIAN_POINT('Ctrl Pts',(0.119369964339924,-0.100263394320381,
-0.537975274226936));
#79521=CARTESIAN_POINT('Ctrl Pts',(0.125766153760101,-0.0921130466933787,
-0.537239392038174));
#79522=CARTESIAN_POINT('Ctrl Pts',(0.1312909864909,-0.0834175003596152,
-0.536503509849412));
#79523=CARTESIAN_POINT('Ctrl Pts',(0.136854524679874,-0.0746610354204685,
-0.535762472272484));
#79524=CARTESIAN_POINT('Ctrl Pts',(0.141533929313437,-0.0653524976398771,
-0.535021434695556));
#79525=CARTESIAN_POINT('Ctrl Pts',(0.145237589286669,-0.0556942111731263,
-0.534280397118628));
#79526=CARTESIAN_POINT('Ctrl Pts',(0.148941249259901,-0.0460359247063756,
-0.5335393595417));
#79527=CARTESIAN_POINT('Ctrl Pts',(0.151668947076162,-0.0360288169028614,
-0.532798321964772));
#79528=CARTESIAN_POINT('Ctrl Pts',(0.153380429140839,-0.0258891184973931,
-0.532057284387844));
#79529=CARTESIAN_POINT('Ctrl Pts',(0.155083892865825,-0.0157969248527707,
-0.531319718591975));
#79530=CARTESIAN_POINT('Ctrl Pts',(0.155793341611836,-0.00549837891997462,
-0.530582152796106));
#79531=CARTESIAN_POINT('Ctrl Pts',(0.155476165663079,0.00479211964654155,
-0.529844587000237));
#79532=CARTESIAN_POINT('Ctrl Pts',(0.155158235733579,0.0151070804643411,
-0.529105267886031));
#79533=CARTESIAN_POINT('Ctrl Pts',(0.153808675124117,0.0254130241057423,
-0.528365948771825));
#79534=CARTESIAN_POINT('Ctrl Pts',(0.151447160819724,0.0354902800727829,
-0.527626629657619));
#79535=CARTESIAN_POINT('Ctrl Pts',(0.149096624655142,0.0455206891819837,
-0.526890747468857));
#79536=CARTESIAN_POINT('Ctrl Pts',(0.145743732290646,0.0553236233514978,
-0.526154865280095));
#79537=CARTESIAN_POINT('Ctrl Pts',(0.141459069430118,0.0646926129937966,
-0.525418983091334));
#79538=CARTESIAN_POINT('Ctrl Pts',(0.137144389400339,0.0741272392000329,
-0.524677945514405));
#79539=CARTESIAN_POINT('Ctrl Pts',(0.131885215706989,0.0831209478566759,
-0.523936907937477));
#79540=CARTESIAN_POINT('Ctrl Pts',(0.125801356714249,0.0914867266266224,
-0.523195870360549));
#79541=CARTESIAN_POINT('Ctrl Pts',(0.119717497721509,0.0998525053965686,
-0.522454832783621));
#79542=CARTESIAN_POINT('Ctrl Pts',(0.112809612786503,0.107589666871735,
-0.521713795206692));
#79543=CARTESIAN_POINT('Ctrl Pts',(0.105237140814391,0.114546700926792,
-0.520972757629764));
#79544=CARTESIAN_POINT('Ctrl Pts',(0.104283464657723,0.115422868910494,
-0.520879431451613));
#79545=CARTESIAN_POINT('Ctrl Pts',(0.103318400484365,0.116287535202872,
-0.520786105273462));
#79546=CARTESIAN_POINT('Ctrl Pts',(0.10234224283772,0.117140376604078,-0.520692779095311));
#79547=CARTESIAN_POINT('Ctrl Pts',(0.10234224283772,0.117140376604078,-0.590700225539723));
#79548=CARTESIAN_POINT('Ctrl Pts',(0.0945759900385656,0.123925532610504,
-0.589962670975134));
#79549=CARTESIAN_POINT('Ctrl Pts',(0.0861446319710369,0.129924196060971,
-0.589225116410546));
#79550=CARTESIAN_POINT('Ctrl Pts',(0.0772334289168642,0.135021479616184,
-0.588487561845957));
#79551=CARTESIAN_POINT('Ctrl Pts',(0.0731752806521563,0.137342774764389,
-0.588151680623386));
#79552=CARTESIAN_POINT('Ctrl Pts',(0.0690179807080798,0.13947775775794,
-0.587815799400815));
#79553=CARTESIAN_POINT('Ctrl Pts',(0.0647804987047992,0.141418844174168,
-0.587479918178244));
#79554=CARTESIAN_POINT('Ctrl Pts',(0.0554753587439913,0.145681300218828,
-0.586742352382375));
#79555=CARTESIAN_POINT('Ctrl Pts',(0.0457131421812634,0.149037264109502,
-0.586004786586507));
#79556=CARTESIAN_POINT('Ctrl Pts',(0.0356924565438694,0.151399640177459,
-0.585267220790638));
#79557=CARTESIAN_POINT('Ctrl Pts',(0.0256479500460458,0.153767632011904,
-0.584527901676432));
#79558=CARTESIAN_POINT('Ctrl Pts',(0.0153446128696165,0.155136949800867,
-0.583788582562226));
#79559=CARTESIAN_POINT('Ctrl Pts',(0.00499970289725095,0.155469628773401,
-0.583049263448019));
#79560=CARTESIAN_POINT('Ctrl Pts',(-0.00529711595503014,0.155800761197492,
-0.582313381259257));
#79561=CARTESIAN_POINT('Ctrl Pts',(-0.0156341898672312,0.155104838447875,
-0.581577499070495));
#79562=CARTESIAN_POINT('Ctrl Pts',(-0.0257938077430798,0.153396486211755,
-0.580841616881734));
#79563=CARTESIAN_POINT('Ctrl Pts',(-0.0360246011067592,0.151676165729852,
-0.580100579304805));
#79564=CARTESIAN_POINT('Ctrl Pts',(-0.0460745035593139,0.148929319532569,
-0.579359541727877));
#79565=CARTESIAN_POINT('Ctrl Pts',(-0.0557318303393841,0.145223157888204,
-0.578618504150949));
#79566=CARTESIAN_POINT('Ctrl Pts',(-0.0653891571194546,0.141516996243838,
-0.57787746657402));
#79567=CARTESIAN_POINT('Ctrl Pts',(-0.0746530733419271,0.136851977681057,
-0.577136428997092));
#79568=CARTESIAN_POINT('Ctrl Pts',(-0.0833359041818016,0.131342794146468,
-0.576395391420164));
#79569=CARTESIAN_POINT('Ctrl Pts',(-0.0919780557247169,0.125859421285511,
-0.575657825624295));
#79570=CARTESIAN_POINT('Ctrl Pts',(-0.100108806789627,0.119499055496214,
-0.574920259828425));
#79571=CARTESIAN_POINT('Ctrl Pts',(-0.107546956153075,0.112380846776524,
-0.574182694032556));
#79572=CARTESIAN_POINT('Ctrl Pts',(-0.115002787252504,0.105245716873743,
-0.57344337491835));
#79573=CARTESIAN_POINT('Ctrl Pts',(-0.121761947599551,0.0973496710543972,
-0.572704055804144));
#79574=CARTESIAN_POINT('Ctrl Pts',(-0.127674287438919,0.0888542560993244,
-0.571964736689938));
#79575=CARTESIAN_POINT('Ctrl Pts',(-0.133559142162814,0.0803983343850622,
-0.571228854501176));
#79576=CARTESIAN_POINT('Ctrl Pts',(-0.138604496885118,0.0713493675232609,
-0.570492972312413));
#79577=CARTESIAN_POINT('Ctrl Pts',(-0.142704064190848,0.0618979205096121,
-0.569757090123651));
#79578=CARTESIAN_POINT('Ctrl Pts',(-0.146832351937288,0.0523802592583791,
-0.569016052546723));
#79579=CARTESIAN_POINT('Ctrl Pts',(-0.150001158894252,0.0424553226940098,
-0.568275014969795));
#79580=CARTESIAN_POINT('Ctrl Pts',(-0.152151583490725,0.0323372562420647,
-0.567533977392867));
#79581=CARTESIAN_POINT('Ctrl Pts',(-0.154302008087198,0.02221918979012,
-0.566792939815939));
#79582=CARTESIAN_POINT('Ctrl Pts',(-0.155433980268412,0.0119089433842917,
-0.566051902239011));
#79583=CARTESIAN_POINT('Ctrl Pts',(-0.155541497310893,0.00162638073205886,
-0.565310864662084));
#79584=CARTESIAN_POINT('Ctrl Pts',(-0.155547131016045,0.00108759241670174,
-0.565272035587932));
#79585=CARTESIAN_POINT('Ctrl Pts',(-0.155549965226619,0.000548774778162832,
-0.565233206513781));
#79586=CARTESIAN_POINT('Ctrl Pts',(-0.155549999681981,9.94664380414222E-6,
-0.56519437743963));
#79587=CARTESIAN_POINT('Ctrl Pts',(0.102342242827937,0.117140376612625,
-0.604616163143584));
#79588=CARTESIAN_POINT('Ctrl Pts',(0.0998150425810934,0.119348320182694,
-0.604387819509448));
#79589=CARTESIAN_POINT('Ctrl Pts',(0.0972171874948015,0.121473785577786,
-0.604156835154237));
#79590=CARTESIAN_POINT('Ctrl Pts',(0.0933494900658883,0.124434607298007,
-0.603816750628649));
#79591=CARTESIAN_POINT('Ctrl Pts',(0.0921328779487807,0.125338068064333,
-0.603710300531447));
#79592=CARTESIAN_POINT('Ctrl Pts',(0.089979157887175,0.12688912730739,-0.603522643187757));
#79593=CARTESIAN_POINT('Ctrl Pts',(0.0890477598874706,0.12754448563957,
-0.603441740309642));
#79594=CARTESIAN_POINT('Ctrl Pts',(0.0870925289375224,0.12888838602375,
-0.603272373972136));
#79595=CARTESIAN_POINT('Ctrl Pts',(0.0860675356096406,0.129575089431532,
-0.603183848682771));
#79596=CARTESIAN_POINT('Ctrl Pts',(0.0833515654433992,0.131348233833454,
-0.602949896444857));
#79597=CARTESIAN_POINT('Ctrl Pts',(0.0816475618471532,0.132414187079245,
-0.602803730197593));
#79598=CARTESIAN_POINT('Ctrl Pts',(0.071979906474285,0.138204303641591,
-0.601977470121882));
#79599=CARTESIAN_POINT('Ctrl Pts',(0.0636288439327093,0.142242226887767,
-0.60127335976255));
#79600=CARTESIAN_POINT('Ctrl Pts',(0.0477839774950291,0.148227862987484,
-0.599964745161302));
#79601=CARTESIAN_POINT('Ctrl Pts',(0.0404068131036379,0.150406457570353,
-0.599365867859013));
#79602=CARTESIAN_POINT('Ctrl Pts',(0.0293474793061623,0.152799640421348,
-0.598502774539392));
#79603=CARTESIAN_POINT('Ctrl Pts',(0.0257700240752542,0.153443524964562,
-0.598228886167105));
#79604=CARTESIAN_POINT('Ctrl Pts',(0.0211221815468206,0.154112890609183,
-0.597882412887712));
#79605=CARTESIAN_POINT('Ctrl Pts',(0.0200698099466869,0.154253468355781,
-0.59780458073061));
#79606=CARTESIAN_POINT('Ctrl Pts',(0.0183471744985145,0.154465652691051,
-0.59767827085864));
#79607=CARTESIAN_POINT('Ctrl Pts',(0.0176777600081493,0.154543694536126,
-0.597629456313642));
#79608=CARTESIAN_POINT('Ctrl Pts',(0.0164180600914171,0.154682260957708,
-0.597538129693187));
#79609=CARTESIAN_POINT('Ctrl Pts',(0.0158278981167646,0.15474376312115,
-0.597495562978908));
#79610=CARTESIAN_POINT('Ctrl Pts',(0.0142547836392661,0.154898607173697,
-0.597382647552801));
#79611=CARTESIAN_POINT('Ctrl Pts',(0.0132712494284984,0.154985971730992,
-0.597312621305776));
#79612=CARTESIAN_POINT('Ctrl Pts',(0.00958792636806592,0.155277829880607,
-0.597052279371541));
#79613=CARTESIAN_POINT('Ctrl Pts',(0.00688360760620281,0.155421204888379,
-0.596864958160466));
#79614=CARTESIAN_POINT('Ctrl Pts',(-0.00620469275255882,0.15577277024577,
-0.595970848623132));
#79615=CARTESIAN_POINT('Ctrl Pts',(-0.0165888740100899,0.155011304330156,
-0.595297961995004));
#79616=CARTESIAN_POINT('Ctrl Pts',(-0.0319408257475522,0.152324022328808,
-0.594266841627171));
#79617=CARTESIAN_POINT('Ctrl Pts',(-0.0370127121583655,0.15117168092893,
-0.593920310074924));
#79618=CARTESIAN_POINT('Ctrl Pts',(-0.0454116615595252,0.148815366142515,
-0.593327470087366));
#79619=CARTESIAN_POINT('Ctrl Pts',(-0.0487725891355586,0.147747973333673,
-0.593084997483356));
#79620=CARTESIAN_POINT('Ctrl Pts',(-0.0535234700514198,0.146059377216428,
-0.592732974518025));
#79621=CARTESIAN_POINT('Ctrl Pts',(-0.0549452297824081,0.145530494944406,
-0.592626417803915));
#79622=CARTESIAN_POINT('Ctrl Pts',(-0.0574206648089724,0.144568209673151,
-0.592438638260483));
#79623=CARTESIAN_POINT('Ctrl Pts',(-0.0584777532867934,0.144143859532027,
-0.592357721056862));
#79624=CARTESIAN_POINT('Ctrl Pts',(-0.0606692766908525,0.143236035548666,
-0.59218838925527));
#79625=CARTESIAN_POINT('Ctrl Pts',(-0.0618028094756738,0.142750606281139,
-0.592099913468413));
#79626=CARTESIAN_POINT('Ctrl Pts',(-0.0647655474086041,0.141439927650801,
-0.591866243367773));
#79627=CARTESIAN_POINT('Ctrl Pts',(-0.0665847082572372,0.140592692544722,
-0.591720313012288));
#79628=CARTESIAN_POINT('Ctrl Pts',(-0.0762840186394345,0.13584497829176,
-0.590928551740038));
#79629=CARTESIAN_POINT('Ctrl Pts',(-0.0838378225090265,0.131317481324936,
-0.590261266066728));
#79630=CARTESIAN_POINT('Ctrl Pts',(-0.0963137362461794,0.122322938234272,
-0.589074461510489));
#79631=CARTESIAN_POINT('Ctrl Pts',(-0.101409337993056,0.118132904568405,
-0.588561285514936));
#79632=CARTESIAN_POINT('Ctrl Pts',(-0.109875602360243,0.110218616444432,
-0.587669892211835));
#79633=CARTESIAN_POINT('Ctrl Pts',(-0.113361117766913,0.106630479186699,
-0.587289611919188));
#79634=CARTESIAN_POINT('Ctrl Pts',(-0.117436684371496,0.102008715945132,
-0.586833887023946));
#79635=CARTESIAN_POINT('Ctrl Pts',(-0.118195529853454,0.101128482148289,
-0.586748527041274));
#79636=CARTESIAN_POINT('Ctrl Pts',(-0.119392774864695,0.0997078320408923,
-0.586613143448292));
#79637=CARTESIAN_POINT('Ctrl Pts',(-0.119837519380592,0.0991728564655517,
-0.586562690970635));
#79638=CARTESIAN_POINT('Ctrl Pts',(-0.120690219920308,0.0981330451347261,
-0.58646567493535));
#79639=CARTESIAN_POINT('Ctrl Pts',(-0.121098627389087,0.0976286136213852,
-0.586419081957774));
#79640=CARTESIAN_POINT('Ctrl Pts',(-0.12201199976512,0.0964859404853927,
-0.586314556959513));
#79641=CARTESIAN_POINT('Ctrl Pts',(-0.122515145201835,0.0958462522484865,
-0.586256749872446));
#79642=CARTESIAN_POINT('Ctrl Pts',(-0.124296687781666,0.0935442846325675,
-0.58605112161421));
#79643=CARTESIAN_POINT('Ctrl Pts',(-0.125546529077658,0.0918600561001543,
-0.58590509206591));
#79644=CARTESIAN_POINT('Ctrl Pts',(-0.132378116478352,0.0822541056238159,
-0.585093434538568));
#79645=CARTESIAN_POINT('Ctrl Pts',(-0.137244675340278,0.0738488055202322,
-0.584461666518785));
#79646=CARTESIAN_POINT('Ctrl Pts',(-0.143863392622656,0.0594707889023248,
-0.583418043644269));
#79647=CARTESIAN_POINT('Ctrl Pts',(-0.146096925250789,0.0537506359950271,
-0.58301172543894));
#79648=CARTESIAN_POINT('Ctrl Pts',(-0.14919736666206,0.0441746031745235,
-0.582330250654473));
#79649=CARTESIAN_POINT('Ctrl Pts',(-0.150265767300542,0.0403911468521191,
-0.582060756532267));
#79650=CARTESIAN_POINT('Ctrl Pts',(-0.151560640401428,0.035038036523898,
-0.581676722930967));
#79651=CARTESIAN_POINT('Ctrl Pts',(-0.151908216563964,0.0334990319844365,
-0.581566010055453));
#79652=CARTESIAN_POINT('Ctrl Pts',(-0.152468265765353,0.0308309850849261,
-0.58137341197574));
#79653=CARTESIAN_POINT('Ctrl Pts',(-0.152691755866943,0.0297043644808611,
-0.581291881994168));
#79654=CARTESIAN_POINT('Ctrl Pts',(-0.153125091452318,0.0273856497022283,
-0.581123616003314));
#79655=CARTESIAN_POINT('Ctrl Pts',(-0.15333353923917,0.0261933776743655,
-0.581036841893671));
#79656=CARTESIAN_POINT('Ctrl Pts',(-0.153833001250387,0.023125976408806,
-0.580812886185986));
#79657=CARTESIAN_POINT('Ctrl Pts',(-0.154103647294522,0.0212477848560813,
-0.580675077451669));
#79658=CARTESIAN_POINT('Ctrl Pts',(-0.155151431861578,0.0128969787120623,
-0.580059072281348));
#79659=CARTESIAN_POINT('Ctrl Pts',(-0.155555484778032,0.0063850521473003,
-0.579569611269345));
#79660=CARTESIAN_POINT('Ctrl Pts',(-0.155544704558447,-0.00629461430374163,
-0.578600509511741));
#79661=CARTESIAN_POINT('Ctrl Pts',(-0.155173271014237,-0.0124509474070228,
-0.578122674400401));
#79662=CARTESIAN_POINT('Ctrl Pts',(-0.153582229072617,-0.025683818750784,
-0.577090070143279));
#79663=CARTESIAN_POINT('Ctrl Pts',(-0.152235975584404,-0.0327320539478683,
-0.576536569310194));
#79664=CARTESIAN_POINT('Ctrl Pts',(-0.150000131164609,-0.0412107456605931,
-0.575882667976528));
#79665=CARTESIAN_POINT('Ctrl Pts',(-0.149568073470682,-0.042752272818136,
-0.575764296136786));
#79666=CARTESIAN_POINT('Ctrl Pts',(-0.148888440711779,-0.0450405682797534,
-0.575589619869348));
#79667=CARTESIAN_POINT('Ctrl Pts',(-0.148658891058573,-0.0457925184823436,
-0.575532388915344));
#79668=CARTESIAN_POINT('Ctrl Pts',(-0.148233731198725,-0.047148343390999,
-0.575429542628247));
#79669=CARTESIAN_POINT('Ctrl Pts',(-0.148040117251705,-0.0477527912165003,
-0.575383820772694));
#79670=CARTESIAN_POINT('Ctrl Pts',(-0.147590721842001,-0.0491267628697209,
-0.575280175421845));
#79671=CARTESIAN_POINT('Ctrl Pts',(-0.147332616790405,-0.0498954918868905,
-0.575222385944596));
#79672=CARTESIAN_POINT('Ctrl Pts',(-0.146504349781652,-0.0522998883581296,
-0.575042156789933));
#79673=CARTESIAN_POINT('Ctrl Pts',(-0.145912848620371,-0.0539281381255683,
-0.57492086776839));
#79674=CARTESIAN_POINT('Ctrl Pts',(-0.144427542935354,-0.0578133031334713,
-0.574632518032726));
#79675=CARTESIAN_POINT('Ctrl Pts',(-0.143507854474433,-0.0600598886467181,
-0.574466649324829));
#79676=CARTESIAN_POINT('Ctrl Pts',(-0.139541509471743,-0.0691367819357211,
-0.573796476482044));
#79677=CARTESIAN_POINT('Ctrl Pts',(-0.136056627786375,-0.0757650086505105,
-0.573306694306837));
#79678=CARTESIAN_POINT('Ctrl Pts',(-0.127469274359271,-0.0895801442974672,
-0.5722347070958));
#79679=CARTESIAN_POINT('Ctrl Pts',(-0.122206869638777,-0.0966357789101716,
-0.571652773847899));
#79680=CARTESIAN_POINT('Ctrl Pts',(-0.114933689027951,-0.104836940258661,
-0.570898453780815));
#79681=CARTESIAN_POINT('Ctrl Pts',(-0.113456041177236,-0.106434312367979,
-0.57074749112664));
#79682=CARTESIAN_POINT('Ctrl Pts',(-0.11097996972815,-0.109000836748831,
-0.570497776178663));
#79683=CARTESIAN_POINT('Ctrl Pts',(-0.110001157464275,-0.109988550440371,
-0.570399855386544));
#79684=CARTESIAN_POINT('Ctrl Pts',(-0.108206392304892,-0.111751715270577,
-0.570221627566613));
#79685=CARTESIAN_POINT('Ctrl Pts',(-0.107395005374523,-0.112531692874178,
-0.570141525683205));
#79686=CARTESIAN_POINT('Ctrl Pts',(-0.105624239608196,-0.114197316590045,
-0.569967671848425));
#79687=CARTESIAN_POINT('Ctrl Pts',(-0.104662037190724,-0.1150798196411,
-0.569873794627664));
#79688=CARTESIAN_POINT('Ctrl Pts',(-0.101932136969279,-0.117521044822269,
-0.569609014083028));
#79689=CARTESIAN_POINT('Ctrl Pts',(-0.100140026492689,-0.119051797543412,
-0.569436981292475));
#79690=CARTESIAN_POINT('Ctrl Pts',(-0.0921100907692925,-0.125601049043539,
-0.568673435472315));
#79691=CARTESIAN_POINT('Ctrl Pts',(-0.0855258502945346,-0.130173675227222,
-0.56806523586275));
#79692=CARTESIAN_POINT('Ctrl Pts',(-0.0709828988432958,-0.138692350175944,
-0.566765240122859));
#79693=CARTESIAN_POINT('Ctrl Pts',(-0.0629778727260717,-0.142505907178222,
-0.566073614822845));
#79694=CARTESIAN_POINT('Ctrl Pts',(-0.0517632843281505,-0.146717930584924,
-0.565163263321706));
#79695=CARTESIAN_POINT('Ctrl Pts',(-0.0488019630281979,-0.147729348496298,
-0.564928232088351));
#79696=CARTESIAN_POINT('Ctrl Pts',(-0.0448177151643822,-0.148957232881636,
-0.56462077811129));
#79697=CARTESIAN_POINT('Ctrl Pts',(-0.0438204265777912,-0.149253660563125,
-0.564544541332005));
#79698=CARTESIAN_POINT('Ctrl Pts',(-0.0422403782342652,-0.149706101111725,
-0.564424971556788));
#79699=CARTESIAN_POINT('Ctrl Pts',(-0.0416595789651382,-0.149868761845605,
-0.56438127755662));
#79700=CARTESIAN_POINT('Ctrl Pts',(-0.0404392606509832,-0.150202886274518,
-0.564290032953742));
#79701=CARTESIAN_POINT('Ctrl Pts',(-0.039799567153663,-0.150373652378502,
-0.564242526025334));
#79702=CARTESIAN_POINT('Ctrl Pts',(-0.0381861888625993,-0.150793326917575,
-0.564123477247869));
#79703=CARTESIAN_POINT('Ctrl Pts',(-0.0372111231790342,-0.151036899184065,
-0.56405223068352));
#79704=CARTESIAN_POINT('Ctrl Pts',(-0.0332416388601625,-0.151987704146258,
-0.563764772207036));
#79705=CARTESIAN_POINT('Ctrl Pts',(-0.0302286892110962,-0.152615524265053,
-0.563552532101712));
#79706=CARTESIAN_POINT('Ctrl Pts',(-0.02160007002832,-0.154147898263196,
-0.562956388272049));
#79707=CARTESIAN_POINT('Ctrl Pts',(-0.0159505497784476,-0.154834514566911,
-0.562579895229941));
#79708=CARTESIAN_POINT('Ctrl Pts',(0.00106119114059613,-0.155960783817813,
-0.561455529620654));
#79709=CARTESIAN_POINT('Ctrl Pts',(0.0124449446903201,-0.155466981141138,
-0.560712833677624));
#79710=CARTESIAN_POINT('Ctrl Pts',(0.0259392871278621,-0.153389093894875,
-0.559772109246303));
#79711=CARTESIAN_POINT('Ctrl Pts',(0.0281975611766819,-0.152990056392549,
-0.559612735041083));
#79712=CARTESIAN_POINT('Ctrl Pts',(0.0317266371894681,-0.152285679263893,
-0.559360163509361));
#79713=CARTESIAN_POINT('Ctrl Pts',(0.033003875630759,-0.152013984965058,
-0.559268025550888));
#79714=CARTESIAN_POINT('Ctrl Pts',(0.0353753058407222,-0.151478239049472,
-0.55909551804472));
#79715=CARTESIAN_POINT('Ctrl Pts',(0.0364703522725195,-0.151218327105364,
-0.559015285303121));
#79716=CARTESIAN_POINT('Ctrl Pts',(0.0389115969426395,-0.150610833003047,
-0.558835081450299));
#79717=CARTESIAN_POINT('Ctrl Pts',(0.0402561341864923,-0.15025704250793,
-0.558734917168882));
#79718=CARTESIAN_POINT('Ctrl Pts',(0.0442841879615979,-0.149139189274522,
-0.558431980549979));
#79719=CARTESIAN_POINT('Ctrl Pts',(0.0469519357936611,-0.148320939061457,
-0.558227494882442));
#79720=CARTESIAN_POINT('Ctrl Pts',(0.0556324181781097,-0.145400815980659,
-0.557548958222977));
#79721=CARTESIAN_POINT('Ctrl Pts',(0.0615376109355467,-0.143001635756755,
-0.557065955972878));
#79722=CARTESIAN_POINT('Ctrl Pts',(0.0769143144703095,-0.135625238282909,
-0.555754570580502));
#79723=CARTESIAN_POINT('Ctrl Pts',(0.0860479915653236,-0.13002217573752,
-0.554915985248314));
#79724=CARTESIAN_POINT('Ctrl Pts',(0.0964558301335115,-0.122057055398578,
-0.553927138374224));
#79725=CARTESIAN_POINT('Ctrl Pts',(0.0983420769699213,-0.120542479916192,
-0.553746551922497));
#79726=CARTESIAN_POINT('Ctrl Pts',(0.100917076410527,-0.11837416872505,
-0.553498915186564));
#79727=CARTESIAN_POINT('Ctrl Pts',(0.101636228897111,-0.117757280999884,
-0.553429630342887));
#79728=CARTESIAN_POINT('Ctrl Pts',(0.102835169580987,-0.116709665321775,
-0.553313975101571));
#79729=CARTESIAN_POINT('Ctrl Pts',(0.103317989862954,-0.116282462637515,
-0.553267360018536));
#79730=CARTESIAN_POINT('Ctrl Pts',(0.104322518439007,-0.115382452340274,
-0.553170312582002));
#79731=CARTESIAN_POINT('Ctrl Pts',(0.104843693628346,-0.114909086324636,
-0.553119922095313));
#79732=CARTESIAN_POINT('Ctrl Pts',(0.106244988726247,-0.113618865714547,
-0.552984268454093));
#79733=CARTESIAN_POINT('Ctrl Pts',(0.107118915540285,-0.112795312141819,
-0.552899485811856));
#79734=CARTESIAN_POINT('Ctrl Pts',(0.112140182493943,-0.107952470386524,
-0.552410658544606));
#79735=CARTESIAN_POINT('Ctrl Pts',(0.116071130535236,-0.103714344768788,
-0.552021071111647));
#79736=CARTESIAN_POINT('Ctrl Pts',(0.127771880500659,-0.0895983175565992,
-0.550801144690868));
#79737=CARTESIAN_POINT('Ctrl Pts',(0.134585420876852,-0.0789953923914177,
-0.549991173429477));
#79738=CARTESIAN_POINT('Ctrl Pts',(0.141445265457289,-0.0648021435883795,
-0.548916354524087));
#79739=CARTESIAN_POINT('Ctrl Pts',(0.142750716424631,-0.0618733503971363,
-0.548695302793198));
#79740=CARTESIAN_POINT('Ctrl Pts',(0.144513363343115,-0.0575655238094397,
-0.548369962007351));
#79741=CARTESIAN_POINT('Ctrl Pts',(0.145043267398054,-0.0562170085453605,
-0.548268093072449));
#79742=CARTESIAN_POINT('Ctrl Pts',(0.145953929252702,-0.0538009041046105,
-0.548085424254409));
#79743=CARTESIAN_POINT('Ctrl Pts',(0.146342006493826,-0.0527361712577901,
-0.548004873608401));
#79744=CARTESIAN_POINT('Ctrl Pts',(0.14713471586338,-0.0504851340585873,
-0.54783441585946));
#79745=CARTESIAN_POINT('Ctrl Pts',(0.147536710531374,-0.049297994374511,
-0.547744428581373));
#79746=CARTESIAN_POINT('Ctrl Pts',(0.148574856803444,-0.0461057405625223,
-0.547502135221473));
#79747=CARTESIAN_POINT('Ctrl Pts',(0.149184732420357,-0.0440924279311382,
-0.54734899106169));
#79748=CARTESIAN_POINT('Ctrl Pts',(0.150447093215428,-0.0395986207361951,
-0.547006260523453));
#79749=CARTESIAN_POINT('Ctrl Pts',(0.151079420568643,-0.0371131503261315,
-0.54681609388495));
#79750=CARTESIAN_POINT('Ctrl Pts',(0.152916292400254,-0.0290653332460022,
-0.546198316229022));
#79751=CARTESIAN_POINT('Ctrl Pts',(0.153877064957146,-0.0234525791267074,
-0.545764181616794));
#79752=CARTESIAN_POINT('Ctrl Pts',(0.155504131332962,-0.00932767940001892,
-0.544668174776928));
#79753=CARTESIAN_POINT('Ctrl Pts',(0.155781643987323,-0.000789154788085012,
-0.544001998455278));
#79754=CARTESIAN_POINT('Ctrl Pts',(0.155181025019761,0.0112834596666922,
-0.543080149951416));
#79755=CARTESIAN_POINT('Ctrl Pts',(0.154882255201368,0.0148309997396616,
-0.542811890607801));
#79756=CARTESIAN_POINT('Ctrl Pts',(0.154333748704033,0.0194441924848779,
-0.542468909787829));
#79757=CARTESIAN_POINT('Ctrl Pts',(0.15419418634321,0.0205215907113379,
-0.542389229236602));
#79758=CARTESIAN_POINT('Ctrl Pts',(0.153949031747173,0.0222701482681936,
-0.542260691081167));
#79759=CARTESIAN_POINT('Ctrl Pts',(0.153850313246199,0.0229422109061236,
-0.542211474762342));
#79760=CARTESIAN_POINT('Ctrl Pts',(0.153645683185368,0.0242745476771696,
-0.542114306414622));
#79761=CARTESIAN_POINT('Ctrl Pts',(0.153539910632097,0.0249348251851772,
-0.542066348810515));
#79762=CARTESIAN_POINT('Ctrl Pts',(0.153259254136351,0.0266172662342378,
-0.541944604137886));
#79763=CARTESIAN_POINT('Ctrl Pts',(0.153078396773061,0.0276384231683491,
-0.541871140802929));
#79764=CARTESIAN_POINT('Ctrl Pts',(0.152265011550628,0.0319777861595062,
-0.541560495253131));
#79765=CARTESIAN_POINT('Ctrl Pts',(0.151534651927442,0.035276987411654,
-0.541328136315055));
#79766=CARTESIAN_POINT('Ctrl Pts',(0.149038396369547,0.0450351849884393,
-0.540645231566677));
#79767=CARTESIAN_POINT('Ctrl Pts',(0.146962418313323,0.0514069224264616,
-0.540204888470714));
#79768=CARTESIAN_POINT('Ctrl Pts',(0.140831904942345,0.0667777361337516,
-0.53911490405296));
#79769=CARTESIAN_POINT('Ctrl Pts',(0.136320700492746,0.0755614194340932,
-0.538465868207829));
#79770=CARTESIAN_POINT('Ctrl Pts',(0.129845872110923,0.0856767779354075,
-0.537639186394091));
#79771=CARTESIAN_POINT('Ctrl Pts',(0.128644645664169,0.0874700814795016,
-0.537489412179961));
#79772=CARTESIAN_POINT('Ctrl Pts',(0.126611729710743,0.0903725171093484,
-0.53724125176283));
#79773=CARTESIAN_POINT('Ctrl Pts',(0.125801811569393,0.0914965897499306,
-0.537143678980386));
#79774=CARTESIAN_POINT('Ctrl Pts',(0.124307101756696,0.0935137049932858,
-0.536965816175157));
#79775=CARTESIAN_POINT('Ctrl Pts',(0.123627421022325,0.0944104296098886,
-0.536885727258208));
#79776=CARTESIAN_POINT('Ctrl Pts',(0.122135746598557,0.0963347130909257,
-0.536711593129439));
#79777=CARTESIAN_POINT('Ctrl Pts',(0.121320389871812,0.0973595416558567,
-0.536617419352683));
#79778=CARTESIAN_POINT('Ctrl Pts',(0.11898933642018,0.100214706676362,-0.536350896770465));
#79779=CARTESIAN_POINT('Ctrl Pts',(0.117444555326744,0.102020708158709,
-0.536177394340382));
#79780=CARTESIAN_POINT('Ctrl Pts',(0.111628066576439,0.108513526864028,
-0.535534890508366));
#79781=CARTESIAN_POINT('Ctrl Pts',(0.107113838418182,0.112971568523782,
-0.535056291621251));
#79782=CARTESIAN_POINT('Ctrl Pts',(0.102342237477092,0.117140381287507,
-0.534570457414543));
#79783=CARTESIAN_POINT('Origin',(0.,0.,-1.10400562256037));
#79784=CARTESIAN_POINT('',(0.102342242837719,0.117140376604078,-0.450689508133418));
#79785=CARTESIAN_POINT('',(0.102342242837722,0.117140376604076,-0.464360489961668));
#79786=CARTESIAN_POINT('',(0.10234224283772,0.117140376604078,-1.10400562256037));
#79787=CARTESIAN_POINT('',(-0.155549952262899,0.00012186471943091,-0.495194377443475));
#79788=CARTESIAN_POINT('Ctrl Pts',(-0.155549952262941,0.000121864665597637,
-0.49519437743963));
#79789=CARTESIAN_POINT('Ctrl Pts',(-0.155558009308424,-0.0101622733503201,
-0.494459817921359));
#79790=CARTESIAN_POINT('Ctrl Pts',(-0.154541823275545,-0.020459514100615,
-0.493725258403087));
#79791=CARTESIAN_POINT('Ctrl Pts',(-0.152519911581845,-0.0305528897334775,
-0.492990698884816));
#79792=CARTESIAN_POINT('Ctrl Pts',(-0.150498488090658,-0.0406438282612177,
-0.492256316730276));
#79793=CARTESIAN_POINT('Ctrl Pts',(-0.14747202429582,-0.0505300918992016,
-0.491521934575736));
#79794=CARTESIAN_POINT('Ctrl Pts',(-0.14350997916094,-0.0600057362360169,
-0.490787552421196));
#79795=CARTESIAN_POINT('Ctrl Pts',(-0.13953818484467,-0.0695046967573508,
-0.490051363213835));
#79796=CARTESIAN_POINT('Ctrl Pts',(-0.134626631384355,-0.0785901876366601,
-0.489315174006475));
#79797=CARTESIAN_POINT('Ctrl Pts',(-0.128891766837023,-0.0870787858300196,
-0.488578984799115));
#79798=CARTESIAN_POINT('Ctrl Pts',(-0.126659152731622,-0.090383443491096,
-0.488292382317918));
#79799=CARTESIAN_POINT('Ctrl Pts',(-0.124302218888701,-0.0935979598096855,
-0.48800577983672));
#79800=CARTESIAN_POINT('Ctrl Pts',(-0.12182947505027,-0.0967128818150698,
-0.487719177355523));
#79801=CARTESIAN_POINT('Ctrl Pts',(-0.115465917869771,-0.104729071760014,
-0.486981611559654));
#79802=CARTESIAN_POINT('Ctrl Pts',(-0.108284142641196,-0.112144290598278,
-0.486244045763785));
#79803=CARTESIAN_POINT('Ctrl Pts',(-0.100421731041853,-0.118790902153985,
-0.485506479967916));
#79804=CARTESIAN_POINT('Ctrl Pts',(-0.0925406291636104,-0.125453313826762,
-0.48476716085371));
#79805=CARTESIAN_POINT('Ctrl Pts',(-0.0839762638384047,-0.131342747989288,
-0.484027841739504));
#79806=CARTESIAN_POINT('Ctrl Pts',(-0.0749051052335867,-0.13632691484056,
-0.483288522625298));
#79807=CARTESIAN_POINT('Ctrl Pts',(-0.0658761163701119,-0.141287911440259,
-0.482552640436536));
#79808=CARTESIAN_POINT('Ctrl Pts',(-0.0563458515628692,-0.145351586900182,
-0.481816758247774));
#79809=CARTESIAN_POINT('Ctrl Pts',(-0.046515015375013,-0.148432327491899,
-0.481080876059012));
#79810=CARTESIAN_POINT('Ctrl Pts',(-0.0366153070533836,-0.15153465090466,
-0.480339838482084));
#79811=CARTESIAN_POINT('Ctrl Pts',(-0.0264117019067965,-0.153639917004201,
-0.479598800905156));
#79812=CARTESIAN_POINT('Ctrl Pts',(-0.0161233600777818,-0.154712118981682,
-0.478857763328227));
#79813=CARTESIAN_POINT('Ctrl Pts',(-0.00583501824876717,-0.155784320959164,
-0.478116725751299));
#79814=CARTESIAN_POINT('Ctrl Pts',(0.00453710823583818,-0.155823489254566,
-0.477375688174371));
#79815=CARTESIAN_POINT('Ctrl Pts',(0.0147737473089751,-0.154846823959843,
-0.476634650597443));
#79816=CARTESIAN_POINT('Ctrl Pts',(0.0249624274516175,-0.1538747343684,
-0.475897084801575));
#79817=CARTESIAN_POINT('Ctrl Pts',(0.035092615732708,-0.151889123318184,
-0.475159519005706));
#79818=CARTESIAN_POINT('Ctrl Pts',(0.0449487908546564,-0.148914098394693,
-0.474421953209837));
#79819=CARTESIAN_POINT('Ctrl Pts',(0.0548283957677845,-0.145932001335019,
-0.473682634095631));
#79820=CARTESIAN_POINT('Ctrl Pts',(0.0644317526577002,-0.141955907193368,
-0.472943314981425));
#79821=CARTESIAN_POINT('Ctrl Pts',(0.073551809557291,-0.137061788295819,
-0.472203995867219));
#79822=CARTESIAN_POINT('Ctrl Pts',(0.0826294693985506,-0.132190421037506,
-0.471468113678456));
#79823=CARTESIAN_POINT('Ctrl Pts',(0.0912274894724173,-0.12640998365361,
-0.470732231489695));
#79824=CARTESIAN_POINT('Ctrl Pts',(0.0991647695623966,-0.119842191976102,
-0.469996349300932));
#79825=CARTESIAN_POINT('Ctrl Pts',(0.107157656053065,-0.113228388156963,
-0.469255311724004));
#79826=CARTESIAN_POINT('Ctrl Pts',(0.114479768525023,-0.10581675053189,
-0.468514274147076));
#79827=CARTESIAN_POINT('Ctrl Pts',(0.120981563548319,-0.0977714875687383,
-0.467773236570147));
#79828=CARTESIAN_POINT('Ctrl Pts',(0.127483358571616,-0.0897262246055862,
-0.467032198993219));
#79829=CARTESIAN_POINT('Ctrl Pts',(0.133164343251696,-0.0810481513728482,
-0.466291161416291));
#79830=CARTESIAN_POINT('Ctrl Pts',(0.137919539375875,-0.0719305439875612,
-0.465550123839363));
#79831=CARTESIAN_POINT('Ctrl Pts',(0.1426524572778,-0.0628556528390921,
-0.464812558043494));
#79832=CARTESIAN_POINT('Ctrl Pts',(0.146503453739732,-0.0532779082140079,
-0.464074992247625));
#79833=CARTESIAN_POINT('Ctrl Pts',(0.149375386541972,-0.043391201820604,
-0.463337426451756));
#79834=CARTESIAN_POINT('Ctrl Pts',(0.152254146413029,-0.0334809930580413,
-0.46259810733755));
#79835=CARTESIAN_POINT('Ctrl Pts',(0.154148781561352,-0.0232612011896585,
-0.461858788223344));
#79836=CARTESIAN_POINT('Ctrl Pts',(0.155010262191423,-0.0129468573540533,
-0.461119469109138));
#79837=CARTESIAN_POINT('Ctrl Pts',(0.155867737995108,-0.00268046254355246,
-0.460383586920376));
#79838=CARTESIAN_POINT('Ctrl Pts',(0.155701562959268,0.00767867793224059,
-0.459647704731614));
#79839=CARTESIAN_POINT('Ctrl Pts',(0.15451520569386,0.0179123898289444,
-0.458911822542852));
#79840=CARTESIAN_POINT('Ctrl Pts',(0.15332053713583,0.0282177962958025,
-0.458170784965923));
#79841=CARTESIAN_POINT('Ctrl Pts',(0.151091432852774,0.0383950649584938,
-0.457429747388995));
#79842=CARTESIAN_POINT('Ctrl Pts',(0.147884185479266,0.0482293498311369,
-0.456688709812067));
#79843=CARTESIAN_POINT('Ctrl Pts',(0.144676938105758,0.0580636347037796,
-0.455947672235139));
#79844=CARTESIAN_POINT('Ctrl Pts',(0.140491962857972,0.0675540785365748,
-0.455206634658211));
#79845=CARTESIAN_POINT('Ctrl Pts',(0.135434200201137,0.0765073847146694,
-0.454465597081283));
#79846=CARTESIAN_POINT('Ctrl Pts',(0.130399918229487,0.0854191251297956,
-0.453727999774537));
#79847=CARTESIAN_POINT('Ctrl Pts',(0.124463551504147,0.0938649610089448,
-0.452990402467791));
#79848=CARTESIAN_POINT('Ctrl Pts',(0.117734838928666,0.101657809352952,
-0.452252805161044));
#79849=CARTESIAN_POINT('Ctrl Pts',(0.112981126538093,0.107163314204765,
-0.451731706151836));
#79850=CARTESIAN_POINT('Ctrl Pts',(0.107832998207033,0.112343258516708,
-0.451210607142627));
#79851=CARTESIAN_POINT('Ctrl Pts',(0.102342242837719,0.117140376604078,
-0.450689508133418));
#79852=CARTESIAN_POINT('Ctrl Pts',(0.10234224283772,0.117140376604078,-0.520692779095311));
#79853=CARTESIAN_POINT('Ctrl Pts',(0.0946302156526187,0.123878157221058,
-0.519955465787922));
#79854=CARTESIAN_POINT('Ctrl Pts',(0.0862227979175108,0.129874812435311,
-0.519218152480532));
#79855=CARTESIAN_POINT('Ctrl Pts',(0.0772864419209033,0.134991141913856,
-0.518480839173142));
#79856=CARTESIAN_POINT('Ctrl Pts',(0.0683602118696518,0.140101673987649,
-0.517744361328693));
#79857=CARTESIAN_POINT('Ctrl Pts',(0.0589069874449303,0.144333325515883,
-0.517007883484243));
#79858=CARTESIAN_POINT('Ctrl Pts',(0.0491225935715261,0.147589882108519,
-0.516271405639794));
#79859=CARTESIAN_POINT('Ctrl Pts',(0.0393465649702998,0.150843654473271,
-0.515535557454954));
#79860=CARTESIAN_POINT('Ctrl Pts',(0.0292408044890006,0.153123682619629,
-0.514799709270114));
#79861=CARTESIAN_POINT('Ctrl Pts',(0.0190183539682938,0.154382980643388,
-0.514063861085274));
#79862=CARTESIAN_POINT('Ctrl Pts',(0.00877063935525566,0.155645390936703,
-0.513326194301611));
#79863=CARTESIAN_POINT('Ctrl Pts',(-0.00159341339709402,0.155881936068079,
-0.512588527517949));
#79864=CARTESIAN_POINT('Ctrl Pts',(-0.0118549561801268,0.155097590290653,
-0.511850860734286));
#79865=CARTESIAN_POINT('Ctrl Pts',(-0.0209555468299898,0.154401982427467,
-0.511196650780085));
#79866=CARTESIAN_POINT('Ctrl Pts',(-0.0299750383140325,0.152904264678107,
-0.510542440825884));
#79867=CARTESIAN_POINT('Ctrl Pts',(-0.0387668291020293,0.150641745413992,
-0.509888230871683));
#79868=CARTESIAN_POINT('Ctrl Pts',(-0.0486788216176196,0.148090948363304,
-0.509150665075814));
#79869=CARTESIAN_POINT('Ctrl Pts',(-0.0583748114869105,0.144548188661075,
-0.508413099279945));
#79870=CARTESIAN_POINT('Ctrl Pts',(-0.0676456836184205,0.14007092484808,
-0.507675533484076));
#79871=CARTESIAN_POINT('Ctrl Pts',(-0.0769385941771473,0.135583017823609,
-0.50693621436987));
#79872=CARTESIAN_POINT('Ctrl Pts',(-0.0858034640196526,0.130156428576783,
-0.506196895255664));
#79873=CARTESIAN_POINT('Ctrl Pts',(-0.0940476405090025,0.123898522245786,
-0.505457576141458));
#79874=CARTESIAN_POINT('Ctrl Pts',(-0.102253491707691,0.117669707489838,
-0.504721693952696));
#79875=CARTESIAN_POINT('Ctrl Pts',(-0.109843662867018,0.110617849060189,
-0.503985811763934));
#79876=CARTESIAN_POINT('Ctrl Pts',(-0.11665827623603,0.102891443209035,
-0.503249929575173));
#79877=CARTESIAN_POINT('Ctrl Pts',(-0.123520630911542,0.095110908284094,
-0.502508891998244));
#79878=CARTESIAN_POINT('Ctrl Pts',(-0.129595880763075,0.0866470414031206,
-0.501767854421316));
#79879=CARTESIAN_POINT('Ctrl Pts',(-0.13476195171955,0.0776853838809952,
-0.501026816844388));
#79880=CARTESIAN_POINT('Ctrl Pts',(-0.139928022676026,0.0687237263588701,
-0.50028577926746));
#79881=CARTESIAN_POINT('Ctrl Pts',(-0.144184555132574,0.0592651602194179,
-0.499544741690532));
#79882=CARTESIAN_POINT('Ctrl Pts',(-0.147458031757348,0.0495169806253255,
-0.498803704113603));
#79883=CARTESIAN_POINT('Ctrl Pts',(-0.151288986780027,0.0381086701778544,
-0.497936466631032));
#79884=CARTESIAN_POINT('Ctrl Pts',(-0.153798378570084,0.0262354219127821,
-0.49706922914846));
#79885=CARTESIAN_POINT('Ctrl Pts',(-0.154901888298272,0.0141847630092929,
-0.496201991665888));
#79886=CARTESIAN_POINT('Ctrl Pts',(-0.15532926531208,0.0095176771784699,
-0.495866120258417));
#79887=CARTESIAN_POINT('Ctrl Pts',(-0.155546268242293,0.0048242037730633,
-0.495530248850946));
#79888=CARTESIAN_POINT('Ctrl Pts',(-0.155549952262899,0.000121864719431378,
-0.495194377443475));
#79889=CARTESIAN_POINT('',(-0.155550041019322,1.41736229090128E-5,-0.508861193595026));
#79890=CARTESIAN_POINT('Ctrl Pts',(0.102342237477092,0.117140381287507,
-0.534570457414543));
#79891=CARTESIAN_POINT('Ctrl Pts',(0.100972985009001,0.11833665843562,-0.53443104305554));
#79892=CARTESIAN_POINT('Ctrl Pts',(0.099582537413719,0.119509120344162,
-0.534291061491653));
#79893=CARTESIAN_POINT('Ctrl Pts',(0.0910650113077797,0.12643931883346,
-0.533443640854567));
#79894=CARTESIAN_POINT('Ctrl Pts',(0.083461465507216,0.131582412293558,
-0.532727509774035));
#79895=CARTESIAN_POINT('Ctrl Pts',(0.0730585353124558,0.137352564776124,
-0.531826903790369));
#79896=CARTESIAN_POINT('Ctrl Pts',(0.0706330556814563,0.138615476567551,
-0.531622187174736));
#79897=CARTESIAN_POINT('Ctrl Pts',(0.0672847028607753,0.140248184179539,
-0.531347823242492));
#79898=CARTESIAN_POINT('Ctrl Pts',(0.066389875766124,0.140673981023601,
-0.531275286370639));
#79899=CARTESIAN_POINT('Ctrl Pts',(0.0649522473807156,0.141341292145939,
-0.53116006848315));
#79900=CARTESIAN_POINT('Ctrl Pts',(0.0644120444808691,0.141588289992462,
-0.531117069380187));
#79901=CARTESIAN_POINT('Ctrl Pts',(0.0632567773252321,0.142108534416606,
-0.531025760612177));
#79902=CARTESIAN_POINT('Ctrl Pts',(0.0626413246593988,0.142380897318929,
-0.530977506401075));
#79903=CARTESIAN_POINT('Ctrl Pts',(0.0610544408627348,0.143070876713611,
-0.530854036524967));
#79904=CARTESIAN_POINT('Ctrl Pts',(0.060080464341022,0.143482606888423,
-0.530779163067255));
#79905=CARTESIAN_POINT('Ctrl Pts',(0.0557840135391806,0.145247428329257,
-0.530452524179679));
#79906=CARTESIAN_POINT('Ctrl Pts',(0.0524192264193203,0.146495395938009,
-0.530206221484216));
#79907=CARTESIAN_POINT('Ctrl Pts',(0.0419033837321235,0.14998681017549,
-0.529456603350951));
#79908=CARTESIAN_POINT('Ctrl Pts',(0.0346310201241065,0.151830972795735,
-0.528965941728836));
#79909=CARTESIAN_POINT('Ctrl Pts',(0.0186234321116583,0.154679700136369,
-0.527894424596587));
#79910=CARTESIAN_POINT('Ctrl Pts',(0.0098798350303917,0.155483135521406,
-0.527313858958294));
#79911=CARTESIAN_POINT('Ctrl Pts',(-0.00106187168404021,0.155561617941926,
-0.52656091235647));
#79912=CARTESIAN_POINT('Ctrl Pts',(-0.00323943187548442,0.155531507547467,
-0.526409831115701));
#79913=CARTESIAN_POINT('Ctrl Pts',(-0.00680575629684839,0.155407268769235,
-0.526159961086687));
#79914=CARTESIAN_POINT('Ctrl Pts',(-0.00819520409637836,0.155340194133129,
-0.526062005613909));
#79915=CARTESIAN_POINT('Ctrl Pts',(-0.0107068963187317,0.155185152766832,
-0.525883741305979));
#79916=CARTESIAN_POINT('Ctrl Pts',(-0.0118294527090561,0.155103620833324,
-0.52580363801748));
#79917=CARTESIAN_POINT('Ctrl Pts',(-0.014251682553711,0.154901244769546,
-0.525629811562684));
#79918=CARTESIAN_POINT('Ctrl Pts',(-0.015550908827485,0.154776209831949,
-0.525535963451272));
#79919=CARTESIAN_POINT('Ctrl Pts',(-0.0191892884190071,0.154379787061373,
-0.52527135364745));
#79920=CARTESIAN_POINT('Ctrl Pts',(-0.0215239862790297,0.154071620818185,
-0.525099464843616));
#79921=CARTESIAN_POINT('Ctrl Pts',(-0.0317467551654107,0.152485393445081,
-0.524337189325797));
#79922=CARTESIAN_POINT('Ctrl Pts',(-0.0395354857256762,0.150653780798415,
-0.52373018215175));
#79923=CARTESIAN_POINT('Ctrl Pts',(-0.0555541012174266,0.145558767542852,
-0.522433716972169));
#79924=CARTESIAN_POINT('Ctrl Pts',(-0.0637175524584717,0.142174865096296,
-0.521744445263524));
#79925=CARTESIAN_POINT('Ctrl Pts',(-0.074362447957927,0.136660379959468,
-0.520833097448303));
#79926=CARTESIAN_POINT('Ctrl Pts',(-0.0771297120980275,0.135117889188147,
-0.520595075639688));
#79927=CARTESIAN_POINT('Ctrl Pts',(-0.0807448497918674,0.132955494285235,
-0.520284390647942));
#79928=CARTESIAN_POINT('Ctrl Pts',(-0.0816361451931318,0.132410098501259,
-0.520207816058779));
#79929=CARTESIAN_POINT('Ctrl Pts',(-0.08303389605275,0.131535316210601,
-0.520087847219453));
#79930=CARTESIAN_POINT('Ctrl Pts',(-0.0835440242877966,0.131211902445967,
-0.520044087966065));
#79931=CARTESIAN_POINT('Ctrl Pts',(-0.0846086541113812,0.130528216796133,
-0.519952836610549));
#79932=CARTESIAN_POINT('Ctrl Pts',(-0.0851627645760028,0.130167366445384,
-0.519905387161339));
#79933=CARTESIAN_POINT('Ctrl Pts',(-0.086549685208956,0.129251522339377,
-0.519786690484115));
#79934=CARTESIAN_POINT('Ctrl Pts',(-0.0873794913445005,0.128691991468806,
-0.519715734858861));
#79935=CARTESIAN_POINT('Ctrl Pts',(-0.0907074415816844,0.12640095307398,
-0.519431162204748));
#79936=CARTESIAN_POINT('Ctrl Pts',(-0.0931601692250964,0.124604280814668,
-0.519221417207531));
#79937=CARTESIAN_POINT('Ctrl Pts',(-0.0999549049263591,0.119314119128767,
-0.518635385214551));
#79938=CARTESIAN_POINT('Ctrl Pts',(-0.104164225798949,0.115657533772781,
-0.518266213084619));
#79939=CARTESIAN_POINT('Ctrl Pts',(-0.116474491421627,0.103745288172068,
-0.517136154309814));
#79940=CARTESIAN_POINT('Ctrl Pts',(-0.123857889293638,0.094808131090732,
-0.516381337922129));
#79941=CARTESIAN_POINT('Ctrl Pts',(-0.131427543632126,0.0832332438251946,
-0.515428168475849));
#79942=CARTESIAN_POINT('Ctrl Pts',(-0.132630050004187,0.0813033887961411,
-0.515270110518713));
#79943=CARTESIAN_POINT('Ctrl Pts',(-0.134453751119969,0.078228418935022,
-0.515019162931181));
#79944=CARTESIAN_POINT('Ctrl Pts',(-0.135103627418985,0.0771006251247367,
-0.514927309788746));
#79945=CARTESIAN_POINT('Ctrl Pts',(-0.136289053530319,0.0749824232971751,
-0.514755059438723));
#79946=CARTESIAN_POINT('Ctrl Pts',(-0.13682815511352,0.0739940927532846,
-0.514674795551276));
#79947=CARTESIAN_POINT('Ctrl Pts',(-0.138011506786804,0.0717675042519225,
-0.514494158071738));
#79948=CARTESIAN_POINT('Ctrl Pts',(-0.138649905627462,0.0705262653712839,
-0.514393586993931));
#79949=CARTESIAN_POINT('Ctrl Pts',(-0.140527208063637,0.0667521978346223,
-0.514088078786667));
#79950=CARTESIAN_POINT('Ctrl Pts',(-0.141713970661791,0.064194242275946,
-0.513881384751377));
#79951=CARTESIAN_POINT('Ctrl Pts',(-0.14565902497044,0.055047766844389,
-0.513143136466566));
#79952=CARTESIAN_POINT('Ctrl Pts',(-0.148032186792093,0.0483037830308538,
-0.512599771579437));
#79953=CARTESIAN_POINT('Ctrl Pts',(-0.152929736687253,0.0305760956604584,
-0.511181624682878));
#79954=CARTESIAN_POINT('Ctrl Pts',(-0.154740495121597,0.0194372652676603,
-0.510298573659076));
#79955=CARTESIAN_POINT('Ctrl Pts',(-0.155411548403831,0.0067255792362609,
-0.509350833115812));
#79956=CARTESIAN_POINT('Ctrl Pts',(-0.155468393194625,0.00524994551898382,
-0.509241768242182));
#79957=CARTESIAN_POINT('Ctrl Pts',(-0.155521244365075,0.00307206358973816,
-0.509082413826389));
#79958=CARTESIAN_POINT('Ctrl Pts',(-0.155533522240653,0.00237034460314847,
-0.509031316513663));
#79959=CARTESIAN_POINT('Ctrl Pts',(-0.155544885369041,0.00131108100834932,
-0.508954580178308));
#79960=CARTESIAN_POINT('Ctrl Pts',(-0.155547487800726,0.00095359563289769,
-0.508928750972098));
#79961=CARTESIAN_POINT('Ctrl Pts',(-0.155549601171384,0.000402122783404505,
-0.5088890140095));
#79962=CARTESIAN_POINT('Ctrl Pts',(-0.155549981691975,0.000208144073060478,
-0.508875057311901));
#79963=CARTESIAN_POINT('Ctrl Pts',(-0.155549999355145,1.41638460410301E-5,
-0.508861120692133));
#79964=CARTESIAN_POINT('Ctrl Pts',(-0.155549999353784,1.41787797109209E-5,
-0.508861121765051));
#79965=CARTESIAN_POINT('Ctrl Pts',(-0.155550034413735,-0.000370450604623472,
-0.50883348784606));
#79966=CARTESIAN_POINT('Ctrl Pts',(-0.155548642861194,-0.000755085092070137,
-0.508805932927192));
#79967=CARTESIAN_POINT('Ctrl Pts',(-0.15554031328278,-0.00189188609293203,
-0.508724717404013));
#79968=CARTESIAN_POINT('Ctrl Pts',(-0.155529346035297,-0.00264402552005807,
-0.508671272805648));
#79969=CARTESIAN_POINT('Ctrl Pts',(-0.155468844606933,-0.00541450384071664,
-0.508475381088768));
#79970=CARTESIAN_POINT('Ctrl Pts',(-0.155385471574864,-0.00743200523510162,
-0.508334625547325));
#79971=CARTESIAN_POINT('Ctrl Pts',(-0.154637454033681,-0.0197252235025581,
-0.507485393419724));
#79972=CARTESIAN_POINT('Ctrl Pts',(-0.152993023103531,-0.0299167630772429,
-0.506816062842887));
#79973=CARTESIAN_POINT('Ctrl Pts',(-0.148459062233549,-0.0470138635843441,
-0.505648838352569));
#79974=CARTESIAN_POINT('Ctrl Pts',(-0.146058844217895,-0.0540110537988211,
-0.505157706628213));
#79975=CARTESIAN_POINT('Ctrl Pts',(-0.142099170703203,-0.0633335686225085,
-0.50446353461855));
#79976=CARTESIAN_POINT('Ctrl Pts',(-0.140961194292705,-0.0658274667872572,
-0.50427379150135));
#79977=CARTESIAN_POINT('Ctrl Pts',(-0.139151676349582,-0.0695307181344438,
-0.503985111314698));
#79978=CARTESIAN_POINT('Ctrl Pts',(-0.138528885218867,-0.0707633912287268,
-0.503887838584097));
#79979=CARTESIAN_POINT('Ctrl Pts',(-0.137369148222479,-0.072984828500458,
-0.503710288796056));
#79980=CARTESIAN_POINT('Ctrl Pts',(-0.136837725112853,-0.0739763809579472,
-0.503630209358879));
#79981=CARTESIAN_POINT('Ctrl Pts',(-0.135662788977779,-0.076112643426853,
-0.503455825248715));
#79982=CARTESIAN_POINT('Ctrl Pts',(-0.135015446170418,-0.0772551351242384,
-0.503361389106862));
#79983=CARTESIAN_POINT('Ctrl Pts',(-0.133180924276198,-0.0803993778312663,
-0.503098136186209));
#79984=CARTESIAN_POINT('Ctrl Pts',(-0.131963212608777,-0.082382813664458,
-0.502928236890759));
#79985=CARTESIAN_POINT('Ctrl Pts',(-0.124772601438793,-0.0935263411314294,
-0.501951018768577));
#79986=CARTESIAN_POINT('Ctrl Pts',(-0.117892342550067,-0.102062195073166,
-0.501110184720737));
#79987=CARTESIAN_POINT('Ctrl Pts',(-0.105975381679225,-0.114019415587182,
-0.499801921796356));
#79988=CARTESIAN_POINT('Ctrl Pts',(-0.101536394896655,-0.117989729688908,
-0.499340669040918));
#79989=CARTESIAN_POINT('Ctrl Pts',(-0.094408515298715,-0.123664139030447,
-0.498648437197397));
#79990=CARTESIAN_POINT('Ctrl Pts',(-0.0918767790759331,-0.125556552478788,
-0.49841111727248));
#79991=CARTESIAN_POINT('Ctrl Pts',(-0.0884585223649684,-0.127952806954091,
-0.498103474783591));
#79992=CARTESIAN_POINT('Ctrl Pts',(-0.0876223977134649,-0.128526832027958,
-0.4980291994366));
#79993=CARTESIAN_POINT('Ctrl Pts',(-0.0862296874233603,-0.129463061560662,
-0.497907161751027));
#79994=CARTESIAN_POINT('Ctrl Pts',(-0.085676301758152,-0.129829945225983,
-0.497859103306455));
#79995=CARTESIAN_POINT('Ctrl Pts',(-0.0846172703227035,-0.130522341558059,
-0.497767977953007));
#79996=CARTESIAN_POINT('Ctrl Pts',(-0.0841120603441055,-0.130848482681996,
-0.497724867699783));
#79997=CARTESIAN_POINT('Ctrl Pts',(-0.0827357067193459,-0.131725729802363,
-0.497608360770412));
#79998=CARTESIAN_POINT('Ctrl Pts',(-0.0818609364035401,-0.132271131773049,
-0.497535325332885));
#79999=CARTESIAN_POINT('Ctrl Pts',(-0.0783785078636803,-0.134394574351762,
-0.497248285123059));
#80000=CARTESIAN_POINT('Ctrl Pts',(-0.0757299472252032,-0.135904636535277,
-0.497038122408536));
#80001=CARTESIAN_POINT('Ctrl Pts',(-0.0641716661516806,-0.142051601800993,
-0.496147809065415));
#80002=CARTESIAN_POINT('Ctrl Pts',(-0.0548683034964049,-0.145897783318279,
-0.495496639247763));
#80003=CARTESIAN_POINT('Ctrl Pts',(-0.0393185507335059,-0.150626687133778,
-0.494421052898173));
#80004=CARTESIAN_POINT('Ctrl Pts',(-0.0332764171580743,-0.152075692279265,
-0.494006310708521));
#80005=CARTESIAN_POINT('Ctrl Pts',(-0.0244223047690646,-0.153646048911707,
-0.493390333417223));
#80006=CARTESIAN_POINT('Ctrl Pts',(-0.0216679392285962,-0.154058612567299,
-0.493197633867709));
#80007=CARTESIAN_POINT('Ctrl Pts',(-0.0175251316291427,-0.154565851287285,
-0.492905370004744));
#80008=CARTESIAN_POINT('Ctrl Pts',(-0.0161439817324513,-0.154716205537186,
-0.492807534477192));
#80009=CARTESIAN_POINT('Ctrl Pts',(-0.0136407136312016,-0.154954832039317,
-0.492629396279327));
#80010=CARTESIAN_POINT('Ctrl Pts',(-0.0125192870006524,-0.155049464277307,
-0.4925492977643));
#80011=CARTESIAN_POINT('Ctrl Pts',(-0.0100938961351406,-0.155227648622655,
-0.492375376192672));
#80012=CARTESIAN_POINT('Ctrl Pts',(-0.00878971719479617,-0.15530695514263,
-0.49228142706628));
#80013=CARTESIAN_POINT('Ctrl Pts',(-0.00519070321734847,-0.155480332747356,
-0.492020907865705));
#80014=CARTESIAN_POINT('Ctrl Pts',(-0.0028946297216905,-0.155540018496285,
-0.491853291530051));
#80015=CARTESIAN_POINT('Ctrl Pts',(0.0107255689918021,-0.155592396912694,
-0.490850098128626));
#80016=CARTESIAN_POINT('Ctrl Pts',(0.0220182511160713,-0.154399279535811,
-0.489978190746555));
#80017=CARTESIAN_POINT('Ctrl Pts',(0.0386583392054416,-0.15077777371226,
-0.488658457201511));
#80018=CARTESIAN_POINT('Ctrl Pts',(0.0441667417124337,-0.149257194507259,
-0.488216301165911));
#80019=CARTESIAN_POINT('Ctrl Pts',(0.0525026422809281,-0.146454045001594,
-0.487548545037632));
#80020=CARTESIAN_POINT('Ctrl Pts',(0.0553963414385408,-0.145384191888921,
-0.487317047741923));
#80021=CARTESIAN_POINT('Ctrl Pts',(0.0591891372278691,-0.143852216441358,
-0.487015661120233));
#80022=CARTESIAN_POINT('Ctrl Pts',(0.0601180949935887,-0.143466473218072,
-0.48694200989087));
#80023=CARTESIAN_POINT('Ctrl Pts',(0.0616523874747325,-0.142811848853248,
-0.486820717962775));
#80024=CARTESIAN_POINT('Ctrl Pts',(0.0622598513655658,-0.142548069163766,
-0.486772788210085));
#80025=CARTESIAN_POINT('Ctrl Pts',(0.06341715585927,-0.142036722021429,
-0.486681677161189));
#80026=CARTESIAN_POINT('Ctrl Pts',(0.0639672691093097,-0.141789825360126,
-0.486638454646653));
#80027=CARTESIAN_POINT('Ctrl Pts',(0.0654617826044792,-0.141108603554031,
-0.486521228380729));
#80028=CARTESIAN_POINT('Ctrl Pts',(0.066403308574594,-0.140667991184,-0.486447593753718));
#80029=CARTESIAN_POINT('Ctrl Pts',(0.0701535193260073,-0.138866933587541,
-0.486154886550108));
#80030=CARTESIAN_POINT('Ctrl Pts',(0.0729256007070044,-0.137431442932353,
-0.485939850573176));
#80031=CARTESIAN_POINT('Ctrl Pts',(0.0833909415714472,-0.131606169821783,
-0.485125963779368));
#80032=CARTESIAN_POINT('Ctrl Pts',(0.0907476807267762,-0.126645634115458,
-0.484548681889078));
#80033=CARTESIAN_POINT('Ctrl Pts',(0.103876513570282,-0.11605861886476,
-0.483435689760726));
#80034=CARTESIAN_POINT('Ctrl Pts',(0.109712144847356,-0.110558385142392,
-0.482902947248217));
#80035=CARTESIAN_POINT('Ctrl Pts',(0.1166835994487,-0.102889726689243,-0.482189222872197));
#80036=CARTESIAN_POINT('Ctrl Pts',(0.118229199977226,-0.101109908029082,
-0.482025447479451));
#80037=CARTESIAN_POINT('Ctrl Pts',(0.12056718469128,-0.0982906978328778,
-0.481768394091764));
#80038=CARTESIAN_POINT('Ctrl Pts',(0.121387959170355,-0.0972752306023971,
-0.481676264259538));
#80039=CARTESIAN_POINT('Ctrl Pts',(0.122892239417772,-0.0953654375535408,
-0.481503764131974));
#80040=CARTESIAN_POINT('Ctrl Pts',(0.123579014082919,-0.0944737865534997,
-0.481423530543508));
#80041=CARTESIAN_POINT('Ctrl Pts',(0.125092488453999,-0.0924640749466919,
-0.481243314523684));
#80042=CARTESIAN_POINT('Ctrl Pts',(0.12591398426824,-0.091342236437221,
-0.481143138800704));
#80043=CARTESIAN_POINT('Ctrl Pts',(0.127981988686494,-0.088437243570197,
-0.480884724783558));
#80044=CARTESIAN_POINT('Ctrl Pts',(0.129206288073323,-0.0866387310763382,
-0.480725671051356));
#80045=CARTESIAN_POINT('Ctrl Pts',(0.135190534387713,-0.0774387271699103,
-0.479916339863465));
#80046=CARTESIAN_POINT('Ctrl Pts',(0.139353300328491,-0.0696695706587878,
-0.479245260513665));
#80047=CARTESIAN_POINT('Ctrl Pts',(0.145794376233024,-0.0547320931331457,
-0.477987681289525));
#80048=CARTESIAN_POINT('Ctrl Pts',(0.148254273165585,-0.0476684220848824,
-0.477405629889092));
#80049=CARTESIAN_POINT('Ctrl Pts',(0.15082799391562,-0.0381130222986628,
-0.476651100529235));
#80050=CARTESIAN_POINT('Ctrl Pts',(0.151404014657583,-0.0357562846715602,
-0.47646762093376));
#80051=CARTESIAN_POINT('Ctrl Pts',(0.152296328759981,-0.0316958744410001,
-0.476156951728635));
#80052=CARTESIAN_POINT('Ctrl Pts',(0.152639711373453,-0.0299986562386409,
-0.47602870633689));
#80053=CARTESIAN_POINT('Ctrl Pts',(0.153102180125304,-0.0274987676104102,
-0.475842499786221));
#80054=CARTESIAN_POINT('Ctrl Pts',(0.153243428496939,-0.0267004022310868,
-0.475783433355032));
#80055=CARTESIAN_POINT('Ctrl Pts',(0.153484116848531,-0.0252751105644787,
-0.475678740258841));
#80056=CARTESIAN_POINT('Ctrl Pts',(0.15358596945583,-0.0246486382811247,
-0.475632986189785));
#80057=CARTESIAN_POINT('Ctrl Pts',(0.153805418384035,-0.0232446561843723,
-0.475531033161508));
#80058=CARTESIAN_POINT('Ctrl Pts',(0.153920957334319,-0.0224668584677605,
-0.475474947448035));
#80059=CARTESIAN_POINT('Ctrl Pts',(0.154253878660928,-0.0201024354085416,
-0.475305560196372));
#80060=CARTESIAN_POINT('Ctrl Pts',(0.154452670520549,-0.0185132406739496,
-0.475193221040861));
#80061=CARTESIAN_POINT('Ctrl Pts',(0.155410549127436,-0.00976008077510311,
-0.474581340573928));
#80062=CARTESIAN_POINT('Ctrl Pts',(0.155695886995841,-0.00255227474429615,
-0.47410250908144));
#80063=CARTESIAN_POINT('Ctrl Pts',(0.155294125701423,0.0108809466628106,
-0.473215299998125));
#80064=CARTESIAN_POINT('Ctrl Pts',(0.154733401815542,0.0170948305963474,
-0.472806936328222));
#80065=CARTESIAN_POINT('Ctrl Pts',(0.153151746601219,0.0275539486532268,
-0.472103326869293));
#80066=CARTESIAN_POINT('Ctrl Pts',(0.152322497727317,0.0318202766477223,
-0.471811685215285));
#80067=CARTESIAN_POINT('Ctrl Pts',(0.150594349094953,0.0390747748456741,
-0.471302720845007));
#80068=CARTESIAN_POINT('Ctrl Pts',(0.149782138188398,0.0420809324082278,
-0.471087887347038));
#80069=CARTESIAN_POINT('Ctrl Pts',(0.148460678986912,0.0464470430144603,
-0.470768915289218));
#80070=CARTESIAN_POINT('Ctrl Pts',(0.148021698981767,0.0478275798202348,
-0.470667025688643));
#80071=CARTESIAN_POINT('Ctrl Pts',(0.147205965746631,0.0502740878637355,
-0.470484508878888));
#80072=CARTESIAN_POINT('Ctrl Pts',(0.146836747216872,0.0513424756543966,
-0.470404132772739));
#80073=CARTESIAN_POINT('Ctrl Pts',(0.146029109669307,0.0535995012085676,
-0.470232855494985));
#80074=CARTESIAN_POINT('Ctrl Pts',(0.145587749733694,0.0547869907292133,
-0.470141862063698));
#80075=CARTESIAN_POINT('Ctrl Pts',(0.144351756042345,0.0579920222648916,
-0.469893805071429));
#80076=CARTESIAN_POINT('Ctrl Pts',(0.143529387203179,0.0599984854298684,
-0.469735832298064));
#80077=CARTESIAN_POINT('Ctrl Pts',(0.137640669489281,0.0735515851616843,
-0.468649795239274));
#80078=CARTESIAN_POINT('Ctrl Pts',(0.131229319903731,0.0844602341709095,
-0.46767498093543));
#80079=CARTESIAN_POINT('Ctrl Pts',(0.119492943675741,0.0998117965549145,
-0.466178528546635));
#80080=CARTESIAN_POINT('Ctrl Pts',(0.115069603996479,0.104880704764188,
-0.465660516783328));
#80081=CARTESIAN_POINT('Ctrl Pts',(0.109198510417998,0.110788414591302,
-0.465039328019619));
#80082=CARTESIAN_POINT('Ctrl Pts',(0.108047499253096,0.111911241269032,
-0.464920424820589));
#80083=CARTESIAN_POINT('Ctrl Pts',(0.106307044207402,0.113557188451459,
-0.464745125340443));
#80084=CARTESIAN_POINT('Ctrl Pts',(0.105730743316155,0.114093964285778,
-0.464687793261765));
#80085=CARTESIAN_POINT('Ctrl Pts',(0.104729214258366,0.115012698505431,
-0.464589418457173));
#80086=CARTESIAN_POINT('Ctrl Pts',(0.104305931785258,0.115396714692346,
-0.46454822598989));
#80087=CARTESIAN_POINT('Ctrl Pts',(0.103370776179674,0.116235769656211,
-0.464458058118187));
#80088=CARTESIAN_POINT('Ctrl Pts',(0.102858006390457,0.116689768536294,
-0.464409157882756));
#80089=CARTESIAN_POINT('Ctrl Pts',(0.102342242837716,0.117140376604081,
-0.464360489961667));
#80090=CARTESIAN_POINT('Origin',(0.,0.,-1.10400562256037));
#80091=CARTESIAN_POINT('',(0.102342242837719,0.117140376604078,-0.380699116973164));
#80092=CARTESIAN_POINT('',(0.102342226162682,0.117140391172586,-0.39458065504025));
#80093=CARTESIAN_POINT('',(0.10234224283772,0.117140376604078,-1.10400562256037));
#80094=CARTESIAN_POINT('',(-0.155549964438899,-0.000105181068850209,-0.425194377435439));
#80095=CARTESIAN_POINT('Ctrl Pts',(-0.155549964438899,-0.000105181068849798,
-0.425194377435439));
#80096=CARTESIAN_POINT('Ctrl Pts',(-0.15554199223784,-0.0118950935007836,
-0.424353019449778));
#80097=CARTESIAN_POINT('Ctrl Pts',(-0.154189456344414,-0.0236317205017142,
-0.423511661464117));
#80098=CARTESIAN_POINT('Ctrl Pts',(-0.151552560981598,-0.0350374622357128,
-0.422670303478456));
#80099=CARTESIAN_POINT('Ctrl Pts',(-0.150029091611429,-0.0416271428202483,
-0.422184207921318));
#80100=CARTESIAN_POINT('Ctrl Pts',(-0.148077844605863,-0.0481067002624013,
-0.421698112364181));
#80101=CARTESIAN_POINT('Ctrl Pts',(-0.145717689281867,-0.0544257065213981,
-0.421212016807043));
#80102=CARTESIAN_POINT('Ctrl Pts',(-0.142136562455347,-0.0640137038031714,
-0.420474451011174));
#80103=CARTESIAN_POINT('Ctrl Pts',(-0.137591758783405,-0.0732823674305032,
-0.419736885215305));
#80104=CARTESIAN_POINT('Ctrl Pts',(-0.132162453570186,-0.0820298016961415,
-0.418999319419436));
#80105=CARTESIAN_POINT('Ctrl Pts',(-0.126720241982456,-0.0907980300888769,
-0.41826000030523));
#80106=CARTESIAN_POINT('Ctrl Pts',(-0.120389682031306,-0.0990416821244272,
-0.417520681191024));
#80107=CARTESIAN_POINT('Ctrl Pts',(-0.11329784291094,-0.106580492078653,
-0.416781362076818));
#80108=CARTESIAN_POINT('Ctrl Pts',(-0.1062389721284,-0.114084255829891,
-0.416045479888056));
#80109=CARTESIAN_POINT('Ctrl Pts',(-0.098426521213838,-0.120889034757036,
-0.415309597699294));
#80110=CARTESIAN_POINT('Ctrl Pts',(-0.0900250076149486,-0.126851489955493,
-0.414573715510532));
#80111=CARTESIAN_POINT('Ctrl Pts',(-0.081564635323124,-0.13285571647474,
-0.413832677933604));
#80112=CARTESIAN_POINT('Ctrl Pts',(-0.0725076815596746,-0.13800521080565,
-0.413091640356676));
#80113=CARTESIAN_POINT('Ctrl Pts',(-0.0630515187879494,-0.142198131065541,
-0.412350602779747));
#80114=CARTESIAN_POINT('Ctrl Pts',(-0.0535953560162242,-0.146391051325432,
-0.411609565202819));
#80115=CARTESIAN_POINT('Ctrl Pts',(-0.043740899244311,-0.149627132860022,
-0.410868527625891));
#80116=CARTESIAN_POINT('Ctrl Pts',(-0.0337020367136042,-0.151855112595378,
-0.410127490048963));
#80117=CARTESIAN_POINT('Ctrl Pts',(-0.023710206524963,-0.154072654185505,
-0.409389924253095));
#80118=CARTESIAN_POINT('Ctrl Pts',(-0.0134614412551567,-0.155308039266046,
-0.408652358457228));
#80119=CARTESIAN_POINT('Ctrl Pts',(-0.00316819151771157,-0.155517732308914,
-0.40791479266136));
#80120=CARTESIAN_POINT('Ctrl Pts',(0.00714952701103393,-0.155727923827525,
-0.407175473547153));
#80121=CARTESIAN_POINT('Ctrl Pts',(0.0175110175694432,-0.154907374263842,
-0.406436154432947));
#80122=CARTESIAN_POINT('Ctrl Pts',(0.027695890656914,-0.153064496669607,
-0.40569683531874));
#80123=CARTESIAN_POINT('Ctrl Pts',(0.0378334165991526,-0.151230186191758,
-0.404960953129979));
#80124=CARTESIAN_POINT('Ctrl Pts',(0.0477950452169169,-0.148383194653096,
-0.404225070941218));
#80125=CARTESIAN_POINT('Ctrl Pts',(0.0573709661843662,-0.14458345250779,
-0.403489188752457));
#80126=CARTESIAN_POINT('Ctrl Pts',(0.0670139734197114,-0.140757090414349,
-0.402748151175528));
#80127=CARTESIAN_POINT('Ctrl Pts',(0.0762649600205053,-0.135964914473338,
-0.402007113598599));
#80128=CARTESIAN_POINT('Ctrl Pts',(0.0849310292404507,-0.130317008760015,
-0.40126607602167));
#80129=CARTESIAN_POINT('Ctrl Pts',(0.0935970984603964,-0.124669103046691,
-0.40052503844474));
#80130=CARTESIAN_POINT('Ctrl Pts',(0.101677530059382,-0.11816609088751,
-0.399784000867811));
#80131=CARTESIAN_POINT('Ctrl Pts',(0.109012855546433,-0.110959451267626,
-0.399042963290882));
#80132=CARTESIAN_POINT('Ctrl Pts',(0.1163138148355,-0.103786574948962,-0.398305397495011));
#80133=CARTESIAN_POINT('Ctrl Pts',(0.122930924860931,-0.0958633672169234,
-0.39756783169914));
#80134=CARTESIAN_POINT('Ctrl Pts',(0.128711981306915,-0.0873443093054628,
-0.396830265903269));
#80135=CARTESIAN_POINT('Ctrl Pts',(0.134506780299418,-0.0788050001560606,
-0.396090946789064));
#80136=CARTESIAN_POINT('Ctrl Pts',(0.13946090297529,-0.0696676889163956,
-0.395351627674858));
#80137=CARTESIAN_POINT('Ctrl Pts',(0.143461392679693,-0.0601218039516679,
-0.394612308560653));
#80138=CARTESIAN_POINT('Ctrl Pts',(0.14744328502258,-0.0506202956225042,
-0.393876426371889));
#80139=CARTESIAN_POINT('Ctrl Pts',(0.150480027741536,-0.0407148628101957,
-0.393140544183125));
#80140=CARTESIAN_POINT('Ctrl Pts',(0.152507634197353,-0.0306141145801488,
-0.392404661994361));
#80141=CARTESIAN_POINT('Ctrl Pts',(0.154549445506174,-0.0204426032868703,
-0.391663624417434));
#80142=CARTESIAN_POINT('Ctrl Pts',(0.155567726303639,-0.010073957880923,
-0.390922586840508));
#80143=CARTESIAN_POINT('Ctrl Pts',(0.155549765518353,0.000270087366504549,
-0.390181549263582));
#80144=CARTESIAN_POINT('Ctrl Pts',(0.155531804733066,0.0106141326139321,
-0.389440511686656));
#80145=CARTESIAN_POINT('Ctrl Pts',(0.154477732960773,0.0209326341847206,
-0.388699474109729));
#80146=CARTESIAN_POINT('Ctrl Pts',(0.152427761566985,0.0310093534869439,
-0.387958436532803));
#80147=CARTESIAN_POINT('Ctrl Pts',(0.150387355153145,0.0410390557340294,
-0.387220856569766));
#80148=CARTESIAN_POINT('Ctrl Pts',(0.147345195883627,0.0509037798324544,
-0.386483276606728));
#80149=CARTESIAN_POINT('Ctrl Pts',(0.143347972080018,0.0603917328824605,
-0.385745696643691));
#80150=CARTESIAN_POINT('Ctrl Pts',(0.139359353640141,0.0698592599340547,
-0.385009704568691));
#80151=CARTESIAN_POINT('Ctrl Pts',(0.134420035713166,0.0789507499674971,
-0.384273712493692));
#80152=CARTESIAN_POINT('Ctrl Pts',(0.128625973318703,0.0874709179545767,
-0.383537720418693));
#80153=CARTESIAN_POINT('Ctrl Pts',(0.122834693202875,0.0959869946012906,
-0.382802081763261));
#80154=CARTESIAN_POINT('Ctrl Pts',(0.116189977295208,0.103931512126628,
-0.382066443107829));
#80155=CARTESIAN_POINT('Ctrl Pts',(0.10883162232711,0.111137214656699,-0.381330804452397));
#80156=CARTESIAN_POINT('Ctrl Pts',(0.106725433975545,0.11319970916797,-0.381120241959319));
#80157=CARTESIAN_POINT('Ctrl Pts',(0.10456102684995,0.115201887598262,-0.380909679466242));
#80158=CARTESIAN_POINT('Ctrl Pts',(0.102342242837719,0.117140376604078,
-0.380699116973164));
#80159=CARTESIAN_POINT('Ctrl Pts',(0.102342242837719,0.117140376604078,
-0.450689508133418));
#80160=CARTESIAN_POINT('Ctrl Pts',(0.0945869527699116,0.123915954781355,
-0.449953493924327));
#80161=CARTESIAN_POINT('Ctrl Pts',(0.0861470817054412,0.129925828488917,
-0.449217479715235));
#80162=CARTESIAN_POINT('Ctrl Pts',(0.0771988637065197,0.135041245337942,
-0.448481465506144));
#80163=CARTESIAN_POINT('Ctrl Pts',(0.0682526309237161,0.140155527300894,
-0.447745614586242));
#80164=CARTESIAN_POINT('Ctrl Pts',(0.058799090187575,0.144375305689882,
-0.447009763666341));
#80165=CARTESIAN_POINT('Ctrl Pts',(0.0490395970987759,0.147617480050263,
-0.44627391274644));
#80166=CARTESIAN_POINT('Ctrl Pts',(0.0392574537660712,0.150867178985883,
-0.445536354032633));
#80167=CARTESIAN_POINT('Ctrl Pts',(0.0291688402668807,0.153134515555881,
-0.444798795318827));
#80168=CARTESIAN_POINT('Ctrl Pts',(0.0189889153761444,0.154386604317984,
-0.44406123660502));
#80169=CARTESIAN_POINT('Ctrl Pts',(0.0158596541469504,0.154771490538738,
-0.443834514511081));
#80170=CARTESIAN_POINT('Ctrl Pts',(0.0127217996521047,0.155060815621456,
-0.443607792417142));
#80171=CARTESIAN_POINT('Ctrl Pts',(0.00958162925438207,0.155254613074239,
-0.443381070323204));
#80172=CARTESIAN_POINT('Ctrl Pts',(-0.000633882777645995,0.155885069374354,
-0.442643504527335));
#80173=CARTESIAN_POINT('Ctrl Pts',(-0.0109498481215258,0.155505299869314,
-0.441905938731466));
#80174=CARTESIAN_POINT('Ctrl Pts',(-0.0211496244755702,0.154105470002016,
-0.441168372935597));
#80175=CARTESIAN_POINT('Ctrl Pts',(-0.0313736474188955,0.152702312502947,
-0.440429053821391));
#80176=CARTESIAN_POINT('Ctrl Pts',(-0.041479989427979,0.150274218729261,
-0.439689734707185));
#80177=CARTESIAN_POINT('Ctrl Pts',(-0.0512522767152041,0.14686390513502,
-0.438950415592979));
#80178=CARTESIAN_POINT('Ctrl Pts',(-0.0609791348742219,0.143469445308576,
-0.438214533404217));
#80179=CARTESIAN_POINT('Ctrl Pts',(-0.0703741556842587,0.13910218191845,
-0.437478651215455));
#80180=CARTESIAN_POINT('Ctrl Pts',(-0.0792394575613944,0.133854065554155,
-0.436742769026693));
#80181=CARTESIAN_POINT('Ctrl Pts',(-0.0881668673045523,0.128569182330418,
-0.436001731449764));
#80182=CARTESIAN_POINT('Ctrl Pts',(-0.0965562831422183,0.122391528630175,
-0.435260693872836));
#80183=CARTESIAN_POINT('Ctrl Pts',(-0.104234359520524,0.115459953210393,
-0.434519656295908));
#80184=CARTESIAN_POINT('Ctrl Pts',(-0.11191243589883,0.108528377790611,
-0.433778618718979));
#80185=CARTESIAN_POINT('Ctrl Pts',(-0.11887855872073,0.100843608776628,
-0.433037581142051));
#80186=CARTESIAN_POINT('Ctrl Pts',(-0.124998863260372,0.0925801635536185,
-0.432296543565123));
#80187=CARTESIAN_POINT('Ctrl Pts',(-0.131118548775831,0.0843175541178476,
-0.431555580938743));
#80188=CARTESIAN_POINT('Ctrl Pts',(-0.136438394268224,0.0754146803388129,
-0.430814618312363));
#80189=CARTESIAN_POINT('Ctrl Pts',(-0.140830805721119,0.0660491230822964,
-0.430073655685982));
#80190=CARTESIAN_POINT('Ctrl Pts',(-0.145212958838233,0.0567054387837563,
-0.429334423554003));
#80191=CARTESIAN_POINT('Ctrl Pts',(-0.14867151697737,0.0469019995313918,
-0.428595191422023));
#80192=CARTESIAN_POINT('Ctrl Pts',(-0.151123982145288,0.0368421568390167,
-0.427855959290043));
#80193=CARTESIAN_POINT('Ctrl Pts',(-0.153574248969686,0.0267913315998867,
-0.427117389791803));
#80194=CARTESIAN_POINT('Ctrl Pts',(-0.155019961917213,0.0164854361025983,
-0.426378820293564));
#80195=CARTESIAN_POINT('Ctrl Pts',(-0.155428695874673,0.00614190513589349,
-0.425640250795324));
#80196=CARTESIAN_POINT('Ctrl Pts',(-0.155510946577613,0.00406044682454401,
-0.425491626343426));
#80197=CARTESIAN_POINT('Ctrl Pts',(-0.15555137271386,0.00197748689463135,
-0.425343001891527));
#80198=CARTESIAN_POINT('Ctrl Pts',(-0.155549964438939,-0.000105181010130192,
-0.425194377439629));
#80199=CARTESIAN_POINT('Ctrl Pts',(0.102342242837716,0.117140376604081,
-0.464360489961667));
#80200=CARTESIAN_POINT('Ctrl Pts',(0.102273383127856,0.117200537390247,
-0.464353992296394));
#80201=CARTESIAN_POINT('Ctrl Pts',(0.10220447005422,0.117260637735246,-0.4643474987721));
#80202=CARTESIAN_POINT('Ctrl Pts',(0.101002868152768,0.118306712630067,
-0.464234433445973));
#80203=CARTESIAN_POINT('Ctrl Pts',(0.0998559583886079,0.119276341474565,
-0.464128972645868));
#80204=CARTESIAN_POINT('Ctrl Pts',(0.0914084520228417,0.126210824756935,
-0.463368331933307));
#80205=CARTESIAN_POINT('Ctrl Pts',(0.0835920180079179,0.131518445458895,
-0.462750010536962));
#80206=CARTESIAN_POINT('Ctrl Pts',(0.0674381492762283,0.140461802163869,
-0.461533810153033));
#80207=CARTESIAN_POINT('Ctrl Pts',(0.0591689174924994,0.144140340351055,
-0.460938180434492));
#80208=CARTESIAN_POINT('Ctrl Pts',(0.0480187542505892,0.147978427119094,
-0.460130162411003));
#80209=CARTESIAN_POINT('Ctrl Pts',(0.0453865098418074,0.148806850643875,
-0.45993918702109));
#80210=CARTESIAN_POINT('Ctrl Pts',(0.0414025381178753,0.149945153824693,
-0.459649012662938));
#80211=CARTESIAN_POINT('Ctrl Pts',(0.0400663387427968,0.150307709713359,
-0.459551504752954));
#80212=CARTESIAN_POINT('Ctrl Pts',(0.0376357935218256,0.150932486575182,
-0.459373709758614));
#80213=CARTESIAN_POINT('Ctrl Pts',(0.0365430915322467,0.151200763219292,
-0.459293623026787));
#80214=CARTESIAN_POINT('Ctrl Pts',(0.0341717262928903,0.151755766435899,
-0.459119435513835));
#80215=CARTESIAN_POINT('Ctrl Pts',(0.0328921665741747,0.152038234364553,
-0.459025205544927));
#80216=CARTESIAN_POINT('Ctrl Pts',(0.029343224387433,0.152774780692246,
-0.458763111187242));
#80217=CARTESIAN_POINT('Ctrl Pts',(0.0270671280667928,0.153194412272351,
-0.458594179714592));
#80218=CARTESIAN_POINT('Ctrl Pts',(0.0138089107062163,0.155334076441763,
-0.45760478160228));
#80219=CARTESIAN_POINT('Ctrl Pts',(0.00267887631684841,0.155923374265372,
-0.456749511995822));
#80220=CARTESIAN_POINT('Ctrl Pts',(-0.0142447024928887,0.155006311867815,
-0.455436053330004));
#80221=CARTESIAN_POINT('Ctrl Pts',(-0.0200506514537917,0.154362711522413,
-0.454983830980701));
#80222=CARTESIAN_POINT('Ctrl Pts',(-0.0288880445425049,0.152875914483139,
-0.454303147399978));
#80223=CARTESIAN_POINT('Ctrl Pts',(-0.0319530889213901,0.152264794739188,
-0.454068555978212));
#80224=CARTESIAN_POINT('Ctrl Pts',(-0.0359822441043171,0.151334402043461,
-0.453763842364232));
#80225=CARTESIAN_POINT('Ctrl Pts',(-0.0369644019649006,0.151097505817334,
-0.453689857362875));
#80226=CARTESIAN_POINT('Ctrl Pts',(-0.0385873217286234,0.150689285796646,
-0.453568166781194));
#80227=CARTESIAN_POINT('Ctrl Pts',(-0.0392294072950517,0.150523406534299,
-0.453520168378703));
#80228=CARTESIAN_POINT('Ctrl Pts',(-0.0404523919771729,0.150199097777176,
-0.453429050557898));
#80229=CARTESIAN_POINT('Ctrl Pts',(-0.0410334616694395,0.150041394442107,
-0.453385888778444));
#80230=CARTESIAN_POINT('Ctrl Pts',(-0.042610685521492,0.149603485142612,
-0.453269050917933));
#80231=CARTESIAN_POINT('Ctrl Pts',(-0.0436050051765083,0.14931670021704,
-0.45319573969795));
#80232=CARTESIAN_POINT('Ctrl Pts',(-0.0475482651125873,0.148136621786212,
-0.452906107010234));
#80233=CARTESIAN_POINT('Ctrl Pts',(-0.0504734535386896,0.147165654402174,
-0.452693715955252));
#80234=CARTESIAN_POINT('Ctrl Pts',(-0.0617153359925256,0.143059401321248,
-0.451880076352907));
#80235=CARTESIAN_POINT('Ctrl Pts',(-0.0697866059163284,0.139300503670522,
-0.451300806194502));
#80236=CARTESIAN_POINT('Ctrl Pts',(-0.0844501399166961,0.130875334844449,
-0.450184824916392));
#80237=CARTESIAN_POINT('Ctrl Pts',(-0.0910866090001889,0.126346298564955,
-0.449651112211696));
#80238=CARTESIAN_POINT('Ctrl Pts',(-0.0991837315935736,0.119849717939578,
-0.448936213283125));
#80239=CARTESIAN_POINT('Ctrl Pts',(-0.100989815815044,0.118331836767116,
-0.448772304710144));
#80240=CARTESIAN_POINT('Ctrl Pts',(-0.103741101150282,0.115910708216065,
-0.44851508852352));
#80241=CARTESIAN_POINT('Ctrl Pts',(-0.104710660537534,0.115035584634023,
-0.448422931494508));
#80242=CARTESIAN_POINT('Ctrl Pts',(-0.106494951341316,0.113383836859246,
-0.448250406662965));
#80243=CARTESIAN_POINT('Ctrl Pts',(-0.107312501171839,0.112610372936681,
-0.448170175899296));
#80244=CARTESIAN_POINT('Ctrl Pts',(-0.109120812231424,0.110861998572991,
-0.447990000553222));
#80245=CARTESIAN_POINT('Ctrl Pts',(-0.110107032500817,0.109882553447126,
-0.447889863085197));
#80246=CARTESIAN_POINT('Ctrl Pts',(-0.112601669766067,0.107337745938541,
-0.447631618782498));
#80247=CARTESIAN_POINT('Ctrl Pts',(-0.114090592093974,0.105753787907573,
-0.447472698339076));
#80248=CARTESIAN_POINT('Ctrl Pts',(-0.121453755798805,0.097584124337845,
-0.446661682269395));
#80249=CARTESIAN_POINT('Ctrl Pts',(-0.126792271660576,0.0905392176756994,
-0.445988649653727));
#80250=CARTESIAN_POINT('Ctrl Pts',(-0.135485092709898,0.07677984111134,
-0.444730370860713));
#80251=CARTESIAN_POINT('Ctrl Pts',(-0.139008039593366,0.0702006063947223,
-0.444149640067028));
#80252=CARTESIAN_POINT('Ctrl Pts',(-0.143033222847984,0.061181452160883,
-0.443396609619197));
#80253=CARTESIAN_POINT('Ctrl Pts',(-0.14396889553151,0.0589460038775934,
-0.443213343113782));
#80254=CARTESIAN_POINT('Ctrl Pts',(-0.145482480732827,0.0550785168834813,
-0.442902993349576));
#80255=CARTESIAN_POINT('Ctrl Pts',(-0.146086069110067,0.0534570508601559,
-0.44277485697675));
#80256=CARTESIAN_POINT('Ctrl Pts',(-0.146932540071791,0.0510616100265278,
-0.442588777164272));
#80257=CARTESIAN_POINT('Ctrl Pts',(-0.147196599843968,0.0502953320134109,
-0.442529730500426));
#80258=CARTESIAN_POINT('Ctrl Pts',(-0.14765675025871,0.0489253455026532,
-0.442425057813741));
#80259=CARTESIAN_POINT('Ctrl Pts',(-0.147855149226051,0.0483224608308629,
-0.442379304609632));
#80260=CARTESIAN_POINT('Ctrl Pts',(-0.148291151917845,0.0469697285999913,
-0.442277335645265));
#80261=CARTESIAN_POINT('Ctrl Pts',(-0.148526764896833,0.0462192743552451,
-0.44222123333554));
#80262=CARTESIAN_POINT('Ctrl Pts',(-0.149225133434975,0.0439343889128088,
-0.442051742500243));
#80263=CARTESIAN_POINT('Ctrl Pts',(-0.149669894145649,0.0423945077254265,
-0.441939318076861));
#80264=CARTESIAN_POINT('Ctrl Pts',(-0.152011041710859,0.0337922473756497,
-0.441319826793158));
#80265=CARTESIAN_POINT('Ctrl Pts',(-0.153431612341769,0.0266090104343941,
-0.440834124095532));
#80266=CARTESIAN_POINT('Ctrl Pts',(-0.155141457102581,0.0129719579906293,
-0.439927036330913));
#80267=CARTESIAN_POINT('Ctrl Pts',(-0.155545019498552,0.0065489010164554,
-0.439505840719987));
#80268=CARTESIAN_POINT('Ctrl Pts',(-0.155554687920093,-0.00604830111625869,
-0.438666773939041));
#80269=CARTESIAN_POINT('Ctrl Pts',(-0.155192595328809,-0.0122101478716149,
-0.438250224472298));
#80270=CARTESIAN_POINT('Ctrl Pts',(-0.154245906872207,-0.0201861980903193,
-0.437693067194438));
#80271=CARTESIAN_POINT('Ctrl Pts',(-0.153992741246545,-0.0220344618013044,
-0.437562714821551));
#80272=CARTESIAN_POINT('Ctrl Pts',(-0.153521630372683,-0.0250671192107265,
-0.437346543927467));
#80273=CARTESIAN_POINT('Ctrl Pts',(-0.153323056712552,-0.0262543632955327,
-0.437261336221811));
#80274=CARTESIAN_POINT('Ctrl Pts',(-0.152907496161228,-0.0285731949652815,
-0.437093717823636));
#80275=CARTESIAN_POINT('Ctrl Pts',(-0.152691675561865,-0.0297049143416587,
-0.437011349035311));
#80276=CARTESIAN_POINT('Ctrl Pts',(-0.152146413066709,-0.0324010368771696,
-0.43681372331183));
#80277=CARTESIAN_POINT('Ctrl Pts',(-0.151805391623711,-0.0339629345239154,
-0.436698106679225));
#80278=CARTESIAN_POINT('Ctrl Pts',(-0.150508872076115,-0.0394907939181744,
-0.436284738665284));
#80279=CARTESIAN_POINT('Ctrl Pts',(-0.149421590564192,-0.0434237960688197,
-0.435982888599719));
#80280=CARTESIAN_POINT('Ctrl Pts',(-0.146200630768544,-0.053512430439989,
-0.435187868835745));
#80281=CARTESIAN_POINT('Ctrl Pts',(-0.143832785339941,-0.0595845520368354,
-0.434688508265065));
#80282=CARTESIAN_POINT('Ctrl Pts',(-0.136826691907896,-0.0746785114488359,
-0.433401553096011));
#80283=CARTESIAN_POINT('Ctrl Pts',(-0.131673966068072,-0.0834291387637996,
-0.432609997655158));
#80284=CARTESIAN_POINT('Ctrl Pts',(-0.124851345500854,-0.0927903661990848,
-0.431748100419001));
#80285=CARTESIAN_POINT('Ctrl Pts',(-0.123979763315437,-0.0939517387796647,
-0.431640918226325));
#80286=CARTESIAN_POINT('Ctrl Pts',(-0.122623809719798,-0.095706793057841,
-0.431478759439734));
#80287=CARTESIAN_POINT('Ctrl Pts',(-0.122151130530738,-0.0963093470219964,
-0.431423052111199));
#80288=CARTESIAN_POINT('Ctrl Pts',(-0.121277780371052,-0.0974058877887452,
-0.431321648888495));
#80289=CARTESIAN_POINT('Ctrl Pts',(-0.120878516117451,-0.0979009262303392,
-0.431275864187193));
#80290=CARTESIAN_POINT('Ctrl Pts',(-0.119947627560858,-0.0990407361073701,
-0.431170418168864));
#80291=CARTESIAN_POINT('Ctrl Pts',(-0.119413829548268,-0.0996836905545983,
-0.431110911452802));
#80292=CARTESIAN_POINT('Ctrl Pts',(-0.117668387066577,-0.101751916325438,
-0.430919290288429));
#80293=CARTESIAN_POINT('Ctrl Pts',(-0.116436154482214,-0.103159703961293,
-0.430788542640987));
#80294=CARTESIAN_POINT('Ctrl Pts',(-0.11336641697481,-0.106541678731171,
-0.430472658602986));
#80295=CARTESIAN_POINT('Ctrl Pts',(-0.111502353107589,-0.108491017162094,
-0.430289040084084));
#80296=CARTESIAN_POINT('Ctrl Pts',(-0.102961046808947,-0.116970225698991,
-0.429477907951531));
#80297=CARTESIAN_POINT('Ctrl Pts',(-0.0957543248465152,-0.122939578218008,
-0.4288715835954));
#80298=CARTESIAN_POINT('Ctrl Pts',(-0.0820289690876509,-0.13236500040725,
-0.427768400687438));
#80299=CARTESIAN_POINT('Ctrl Pts',(-0.075719136167067,-0.13607291230543,
-0.42727796413229));
#80300=CARTESIAN_POINT('Ctrl Pts',(-0.0674299815768194,-0.140188391398987,
-0.426636830968148));
#80301=CARTESIAN_POINT('Ctrl Pts',(-0.0656714199494314,-0.141020748534759,
-0.426501022953783));
#80302=CARTESIAN_POINT('Ctrl Pts',(-0.0627851718758298,-0.142321164525712,
-0.426278197111946));
#80303=CARTESIAN_POINT('Ctrl Pts',(-0.061666736694328,-0.142809331323208,
-0.426191868511892));
#80304=CARTESIAN_POINT('Ctrl Pts',(-0.0594889580944578,-0.143729520219288,
-0.426023742695757));
#80305=CARTESIAN_POINT('Ctrl Pts',(-0.058430361601978,-0.14416311536826,
-0.425942005044496));
#80306=CARTESIAN_POINT('Ctrl Pts',(-0.0559271320274577,-0.145156323844406,
-0.425748639461388));
#80307=CARTESIAN_POINT('Ctrl Pts',(-0.0544787547995319,-0.145706099404677,
-0.425636692351353));
#80308=CARTESIAN_POINT('Ctrl Pts',(-0.0495107717165426,-0.147507420714917,
-0.425252350959622));
#80309=CARTESIAN_POINT('Ctrl Pts',(-0.045954659809813,-0.148653693519369,
-0.424976590046232));
#80310=CARTESIAN_POINT('Ctrl Pts',(-0.03690491349467,-0.151215023822785,
-0.424272773075451));
#80311=CARTESIAN_POINT('Ctrl Pts',(-0.0313689887452169,-0.152459605212025,
-0.423840241952703));
#80312=CARTESIAN_POINT('Ctrl Pts',(-0.0174172111038909,-0.154804133058094,
-0.422749811353617));
#80313=CARTESIAN_POINT('Ctrl Pts',(-0.00895560974873443,-0.155523240595038,
-0.422087640583578));
#80314=CARTESIAN_POINT('Ctrl Pts',(0.00315134924843414,-0.155560407106869,
-0.421163818662137));
#80315=CARTESIAN_POINT('Ctrl Pts',(0.00677983169964172,-0.155444555774993,
-0.420890131226195));
#80316=CARTESIAN_POINT('Ctrl Pts',(0.0114915123117164,-0.155128790577476,
-0.420541444965241));
#80317=CARTESIAN_POINT('Ctrl Pts',(0.0125810207736793,-0.155044234389489,
-0.420461286123524));
#80318=CARTESIAN_POINT('Ctrl Pts',(0.0143475853713237,-0.15488838740217,
-0.420332171300241));
#80319=CARTESIAN_POINT('Ctrl Pts',(0.0150252003981042,-0.154824123310057,
-0.420282850866333));
#80320=CARTESIAN_POINT('Ctrl Pts',(0.0163664661775842,-0.154688030640773,
-0.420185661353746));
#80321=CARTESIAN_POINT('Ctrl Pts',(0.0170301157202365,-0.154616374400829,
-0.420137785079173));
#80322=CARTESIAN_POINT('Ctrl Pts',(0.0187179169767573,-0.154423138459113,
-0.420016519502882));
#80323=CARTESIAN_POINT('Ctrl Pts',(0.0197413814980716,-0.15429563867892,
-0.419943448843378));
#80324=CARTESIAN_POINT('Ctrl Pts',(0.0240559714763751,-0.153714506495937,
-0.419637075019275));
#80325=CARTESIAN_POINT('Ctrl Pts',(0.0273336454300653,-0.153165645457995,
-0.419408431574137));
#80326=CARTESIAN_POINT('Ctrl Pts',(0.0369608400545467,-0.151234584568491,
-0.418742316226919));
#80327=CARTESIAN_POINT('Ctrl Pts',(0.0432443585596993,-0.149559154453393,
-0.418314471503221));
#80328=CARTESIAN_POINT('Ctrl Pts',(0.0590104423181322,-0.144278152126124,
-0.417219228716014));
#80329=CARTESIAN_POINT('Ctrl Pts',(0.0682774551253329,-0.140130566603647,
-0.416552929954819));
#80330=CARTESIAN_POINT('Ctrl Pts',(0.0789448092232963,-0.134045340375308,
-0.415707536708337));
#80331=CARTESIAN_POINT('Ctrl Pts',(0.080792149342832,-0.132940076803219,
-0.415558148656184));
#80332=CARTESIAN_POINT('Ctrl Pts',(0.0837883610557263,-0.131061923947238,
-0.415310493492284));
#80333=CARTESIAN_POINT('Ctrl Pts',(0.0849509410998604,-0.130311376115607,
-0.415213033963486));
#80334=CARTESIAN_POINT('Ctrl Pts',(0.0870403383383378,-0.128922643001383,
-0.415035289493543));
#80335=CARTESIAN_POINT('Ctrl Pts',(0.0879705482491184,-0.128289714694196,
-0.414955204343035));
#80336=CARTESIAN_POINT('Ctrl Pts',(0.0899695493219107,-0.126897601253898,
-0.414780976780436));
#80337=CARTESIAN_POINT('Ctrl Pts',(0.0910357652332837,-0.126134889160652,
-0.414686704714272));
#80338=CARTESIAN_POINT('Ctrl Pts',(0.0940125791763811,-0.123948036147847,
-0.414419603700523));
#80339=CARTESIAN_POINT('Ctrl Pts',(0.0959001988389162,-0.122493393351473,
-0.414245613055288));
#80340=CARTESIAN_POINT('Ctrl Pts',(0.104141878542834,-0.115834881100149,
-0.41346460617345));
#80341=CARTESIAN_POINT('Ctrl Pts',(0.110110429949034,-0.110176702456328,
-0.412839979123223));
#80342=CARTESIAN_POINT('Ctrl Pts',(0.121804284386646,-0.0971874513485076,
-0.411490932749007));
#80343=CARTESIAN_POINT('Ctrl Pts',(0.127377024367968,-0.0897596194853495,
-0.410766481811189));
#80344=CARTESIAN_POINT('Ctrl Pts',(0.133626246672558,-0.0796656117833917,
-0.409868924107657));
#80345=CARTESIAN_POINT('Ctrl Pts',(0.134941269304232,-0.0774173063837144,
-0.409674157451417));
#80346=CARTESIAN_POINT('Ctrl Pts',(0.136669366128138,-0.0742848156534651,
-0.409410795660582));
#80347=CARTESIAN_POINT('Ctrl Pts',(0.137131435116893,-0.0734283263261997,
-0.409339589299091));
#80348=CARTESIAN_POINT('Ctrl Pts',(0.137888375438125,-0.0719931944092857,
-0.409221675717405));
#80349=CARTESIAN_POINT('Ctrl Pts',(0.13818771070766,-0.0714169503242614,
-0.409174702458611));
#80350=CARTESIAN_POINT('Ctrl Pts',(0.138800005163743,-0.0702199705311602,
-0.409077921025874));
#80351=CARTESIAN_POINT('Ctrl Pts',(0.139112426231255,-0.0695989842828882,
-0.409028145195357));
#80352=CARTESIAN_POINT('Ctrl Pts',(0.13993486665706,-0.0679365892857792,
-0.408895991464965));
#80353=CARTESIAN_POINT('Ctrl Pts',(0.14043743392055,-0.0668915124230873,
-0.40881405257143));
#80354=CARTESIAN_POINT('Ctrl Pts',(0.143025587441762,-0.0613517310240737,
-0.408385173481009));
#80355=CARTESIAN_POINT('Ctrl Pts',(0.144907436430801,-0.0567644205456595,
-0.408048821671189));
#80356=CARTESIAN_POINT('Ctrl Pts',(0.148781770544489,-0.0458640519402042,
-0.407275160728713));
#80357=CARTESIAN_POINT('Ctrl Pts',(0.150596840885279,-0.0394984105807963,
-0.406842326235232));
#80358=CARTESIAN_POINT('Ctrl Pts',(0.153872789005679,-0.0244256797164644,
-0.405824766218257));
#80359=CARTESIAN_POINT('Ctrl Pts',(0.155008993320746,-0.0156726452948194,
-0.405238624081585));
#80360=CARTESIAN_POINT('Ctrl Pts',(0.155486962600614,-0.00486291610375301,
-0.404489776173616));
#80361=CARTESIAN_POINT('Ctrl Pts',(0.155536818973617,-0.0028532078328083,
-0.404349561852821));
#80362=CARTESIAN_POINT('Ctrl Pts',(0.155554402840785,0.000390639397702419,
-0.404121348660314));
#80363=CARTESIAN_POINT('Ctrl Pts',(0.155546410520769,0.00162445670713242,
-0.404034104909804));
#80364=CARTESIAN_POINT('Ctrl Pts',(0.155502817372158,0.00399665008138526,
-0.403865451645369));
#80365=CARTESIAN_POINT('Ctrl Pts',(0.155469389821721,0.005134990243521,
-0.403784115134633));
#80366=CARTESIAN_POINT('Ctrl Pts',(0.155362365034471,0.00778676847194762,
-0.40359364518516));
#80367=CARTESIAN_POINT('Ctrl Pts',(0.155279148357151,0.00929967837408699,
-0.40348421995326));
#80368=CARTESIAN_POINT('Ctrl Pts',(0.154929577813954,0.0143171410907361,
-0.40311867601386));
#80369=CARTESIAN_POINT('Ctrl Pts',(0.154566572808116,0.017813634039671,
-0.402859623878621));
#80370=CARTESIAN_POINT('Ctrl Pts',(0.15337715702905,0.0264201262367326,
-0.402210856217068));
#80371=CARTESIAN_POINT('Ctrl Pts',(0.152413572980783,0.0315066504079926,
-0.401817543260454));
#80372=CARTESIAN_POINT('Ctrl Pts',(0.148794420336471,0.0464842311849151,
-0.400633233020501));
#80373=CARTESIAN_POINT('Ctrl Pts',(0.145414353709923,0.0561714395871313,
-0.399830857396631));
#80374=CARTESIAN_POINT('Ctrl Pts',(0.139905571106592,0.0680469579368619,
-0.398838574306083));
#80375=CARTESIAN_POINT('Ctrl Pts',(0.138632683588476,0.0706040997296308,
-0.398624512466365));
#80376=CARTESIAN_POINT('Ctrl Pts',(0.136816662605184,0.0740136283129232,
-0.398339879864655));
#80377=CARTESIAN_POINT('Ctrl Pts',(0.136334679761057,0.0748977408188562,
-0.398266146777899));
#80378=CARTESIAN_POINT('Ctrl Pts',(0.135553360973311,0.0762983950045594,
-0.398149526203277));
#80379=CARTESIAN_POINT('Ctrl Pts',(0.135259588628421,0.076817982711238,
-0.398106306925722));
#80380=CARTESIAN_POINT('Ctrl Pts',(0.134630163198465,0.0779164254625724,
-0.3980150491823));
#80381=CARTESIAN_POINT('Ctrl Pts',(0.134293750849438,0.0784948324457345,
-0.397967062234209));
#80382=CARTESIAN_POINT('Ctrl Pts',(0.13342544065371,0.0799658292976259,
-0.397845145390837));
#80383=CARTESIAN_POINT('Ctrl Pts',(0.132888301077491,0.0808553131223326,
-0.39777154106279));
#80384=CARTESIAN_POINT('Ctrl Pts',(0.130556589902209,0.0846305307915819,
-0.397459343169993));
#80385=CARTESIAN_POINT('Ctrl Pts',(0.12867648790279,0.087462651802643,-0.397225633072002));
#80386=CARTESIAN_POINT('Ctrl Pts',(0.12277937583617,0.0957435321447507,
-0.396536526870984));
#80387=CARTESIAN_POINT('Ctrl Pts',(0.118497975758745,0.100994265393113,
-0.39609155030182));
#80388=CARTESIAN_POINT('Ctrl Pts',(0.110232646575901,0.109878865735452,
-0.395292274098939));
#80389=CARTESIAN_POINT('Ctrl Pts',(0.10637872970927,0.113613812895561,-0.394939070889565));
#80390=CARTESIAN_POINT('Ctrl Pts',(0.102342226162682,0.117140391172586,
-0.39458065504025));
#80391=CARTESIAN_POINT('Origin',(0.,0.,-1.10400562256037));
#80392=CARTESIAN_POINT('',(0.102342242837719,0.117140376604078,-0.310696206146068));
#80393=CARTESIAN_POINT('',(0.102342232991206,0.117140385206698,-0.324608715049314));
#80394=CARTESIAN_POINT('',(0.10234224283772,0.117140376604078,-1.10400562256037));
#80395=CARTESIAN_POINT('',(-0.155549994568677,-4.11057744446486E-5,-0.355194377443546));
#80396=CARTESIAN_POINT('Ctrl Pts',(-0.155549994568662,-4.11058288203373E-5,
-0.355194377439629));
#80397=CARTESIAN_POINT('Ctrl Pts',(-0.155549396009725,-0.00230613349326641,
-0.355031203712607));
#80398=CARTESIAN_POINT('Ctrl Pts',(-0.155499326836065,-0.00457044143846376,
-0.354868029985585));
#80399=CARTESIAN_POINT('Ctrl Pts',(-0.155399866787252,-0.00683256192830994,
-0.354704856258563));
#80400=CARTESIAN_POINT('Ctrl Pts',(-0.154950294840852,-0.0170576314285913,
-0.353967290462704));
#80401=CARTESIAN_POINT('Ctrl Pts',(-0.153485536234328,-0.0272761366067171,
-0.353229724666845));
#80402=CARTESIAN_POINT('Ctrl Pts',(-0.151018641087833,-0.0372716050631629,
-0.352492158870986));
#80403=CARTESIAN_POINT('Ctrl Pts',(-0.148545881715323,-0.0472908344347134,
-0.351752839756777));
#80404=CARTESIAN_POINT('Ctrl Pts',(-0.145066294261912,-0.0570850296203176,
-0.351013520642569));
#80405=CARTESIAN_POINT('Ctrl Pts',(-0.140645158956177,-0.0664435231018924,
-0.35027420152836));
#80406=CARTESIAN_POINT('Ctrl Pts',(-0.136244576497222,-0.0757585110878595,
-0.349538319339607));
#80407=CARTESIAN_POINT('Ctrl Pts',(-0.130911576344366,-0.0846409946880161,
-0.348802437150854));
#80408=CARTESIAN_POINT('Ctrl Pts',(-0.124758450002192,-0.0929038839502992,
-0.348066554962102));
#80409=CARTESIAN_POINT('Ctrl Pts',(-0.1185622165495,-0.101224660741753,
-0.347325517385165));
#80410=CARTESIAN_POINT('Ctrl Pts',(-0.111534877784764,-0.108916358423386,
-0.346584479808228));
#80411=CARTESIAN_POINT('Ctrl Pts',(-0.103832776624706,-0.115821228617227,
-0.345843442231292));
#80412=CARTESIAN_POINT('Ctrl Pts',(-0.0961306754646478,-0.122726098811068,
-0.345102404654355));
#80413=CARTESIAN_POINT('Ctrl Pts',(-0.0877546006943488,-0.128843607569754,
-0.344361367077418));
#80414=CARTESIAN_POINT('Ctrl Pts',(-0.0788922047367165,-0.134059026297299,
-0.343620329500482));
#80415=CARTESIAN_POINT('Ctrl Pts',(-0.0700713293439948,-0.139250010646957,
-0.342882763704648));
#80416=CARTESIAN_POINT('Ctrl Pts',(-0.0607031405623345,-0.143585954003829,
-0.342145197908815));
#80417=CARTESIAN_POINT('Ctrl Pts',(-0.0509763064828735,-0.146959922010609,
-0.341407632112981));
#80418=CARTESIAN_POINT('Ctrl Pts',(-0.0412263500771315,-0.150341910508792,
-0.340668312998766));
#80419=CARTESIAN_POINT('Ctrl Pts',(-0.0311168689297538,-0.152756901008259,
-0.339928993884551));
#80420=CARTESIAN_POINT('Ctrl Pts',(-0.0208601042734006,-0.154144927096881,
-0.339189674770336));
#80421=CARTESIAN_POINT('Ctrl Pts',(-0.0106510209703367,-0.155526500569642,
-0.33845379258161));
#80422=CARTESIAN_POINT('Ctrl Pts',(-0.00029694429549402,-0.155890508456486,
-0.337717910392884));
#80423=CARTESIAN_POINT('Ctrl Pts',(0.00998405975226561,-0.155229253205906,
-0.336982028204158));
#80424=CARTESIAN_POINT('Ctrl Pts',(0.0203370896869163,-0.154563365382897,
-0.336240990627199));
#80425=CARTESIAN_POINT('Ctrl Pts',(0.0306150705144891,-0.152857840989834,
-0.335499953050239));
#80426=CARTESIAN_POINT('Ctrl Pts',(0.0406005577015138,-0.150157907598388,
-0.33475891547328));
#80427=CARTESIAN_POINT('Ctrl Pts',(0.0505860448885384,-0.147457974206942,
-0.334017877896321));
#80428=CARTESIAN_POINT('Ctrl Pts',(0.060278161065648,-0.143764002633356,
-0.333276840319362));
#80429=CARTESIAN_POINT('Ctrl Pts',(0.0694784940677451,-0.139170907024702,
-0.332535802742402));
#80430=CARTESIAN_POINT('Ctrl Pts',(0.0786357232622493,-0.134599330192524,
-0.331798236946424));
#80431=CARTESIAN_POINT('Ctrl Pts',(0.087373843924104,-0.129103093918329,
-0.331060671150446));
#80432=CARTESIAN_POINT('Ctrl Pts',(0.0955004280601591,-0.122782208565925,
-0.330323105354468));
#80433=CARTESIAN_POINT('Ctrl Pts',(0.103646330456298,-0.116446297403765,
-0.329583786240289));
#80434=CARTESIAN_POINT('Ctrl Pts',(0.111176962586784,-0.109282264469586,
-0.32884446712611));
#80435=CARTESIAN_POINT('Ctrl Pts',(0.117926453096682,-0.101435467958875,
-0.328105148011931));
#80436=CARTESIAN_POINT('Ctrl Pts',(0.124644566770364,-0.0936251494087723,
-0.327369265823062));
#80437=CARTESIAN_POINT('Ctrl Pts',(0.130588174796864,-0.0851391062085926,
-0.326633383634192));
#80438=CARTESIAN_POINT('Ctrl Pts',(0.135632073353664,-0.076156044919535,
-0.325897501445322));
#80439=CARTESIAN_POINT('Ctrl Pts',(0.140711308074736,-0.0671100507768938,
-0.325156463868489));
#80440=CARTESIAN_POINT('Ctrl Pts',(0.144877701622766,-0.0575608692355155,
-0.324415426291655));
#80441=CARTESIAN_POINT('Ctrl Pts',(0.148050778424439,-0.0477155059484613,
-0.323674388714822));
#80442=CARTESIAN_POINT('Ctrl Pts',(0.151223855226112,-0.0378701426614064,
-0.322933351137988));
#80443=CARTESIAN_POINT('Ctrl Pts',(0.153403448524948,-0.0277295354314074,
-0.322192313561155));
#80444=CARTESIAN_POINT('Ctrl Pts',(0.154561120375391,-0.0175117836985256,
-0.321451275984322));
#80445=CARTESIAN_POINT('Ctrl Pts',(0.155713378648865,-0.0073418128505561,
-0.320713703693404));
#80446=CARTESIAN_POINT('Ctrl Pts',(0.155861855353249,0.00298016479531421,
-0.319976131402487));
#80447=CARTESIAN_POINT('Ctrl Pts',(0.154985645239039,0.0132382880252213,
-0.31923855911157));
#80448=CARTESIAN_POINT('Ctrl Pts',(0.154110671345499,0.0234819383521538,
-0.318502027441043));
#80449=CARTESIAN_POINT('Ctrl Pts',(0.152213864886687,0.0336609894596978,
-0.317765495770516));
#80450=CARTESIAN_POINT('Ctrl Pts',(0.149326363322342,0.0435596110740663,
-0.31702896409999));
#80451=CARTESIAN_POINT('Ctrl Pts',(0.146441745391506,0.0534483473268699,
-0.316293167974486));
#80452=CARTESIAN_POINT('Ctrl Pts',(0.142568636922808,0.0630563155655001,
-0.315557371848983));
#80453=CARTESIAN_POINT('Ctrl Pts',(0.137788530039798,0.0721811851487048,
-0.31482157572348));
#80454=CARTESIAN_POINT('Ctrl Pts',(0.132997950743386,0.0813260457925393,
-0.314084167591929));
#80455=CARTESIAN_POINT('Ctrl Pts',(0.127296846994873,0.0899848734962369,
-0.313346759460377));
#80456=CARTESIAN_POINT('Ctrl Pts',(0.120812856293013,0.0979798767825501,
-0.312609351328826));
#80457=CARTESIAN_POINT('Ctrl Pts',(0.115205461488811,0.104894004508611,
-0.311971636267907));
#80458=CARTESIAN_POINT('Ctrl Pts',(0.109013547816566,0.11131184562285,-0.311333921206987));
#80459=CARTESIAN_POINT('Ctrl Pts',(0.102342242837719,0.117140376604078,
-0.310696206146068));
#80460=CARTESIAN_POINT('Ctrl Pts',(0.102342242837719,0.117140376604078,
-0.380699116973164));
#80461=CARTESIAN_POINT('Ctrl Pts',(0.0945698035973211,0.123930937529717,
-0.379961512873473));
#80462=CARTESIAN_POINT('Ctrl Pts',(0.0861280069020955,0.129936518309589,
-0.379223908773781));
#80463=CARTESIAN_POINT('Ctrl Pts',(0.0772013106887236,0.1350398464452,-0.378486304674089));
#80464=CARTESIAN_POINT('Ctrl Pts',(0.0706967556260747,0.138758453874802,
-0.377948839707633));
#80465=CARTESIAN_POINT('Ctrl Pts',(0.0639354807636149,0.141998879591595,
-0.377411374741178));
#80466=CARTESIAN_POINT('Ctrl Pts',(0.0569959733123979,0.144731688051278,
-0.376873909774722));
#80467=CARTESIAN_POINT('Ctrl Pts',(0.0474728533778924,0.148481934434403,
-0.376136343978859));
#80468=CARTESIAN_POINT('Ctrl Pts',(0.0375426173799939,0.151302178905618,
-0.375398778182996));
#80469=CARTESIAN_POINT('Ctrl Pts',(0.0274083143440573,0.153116252582204,
-0.374661212387134));
#80470=CARTESIAN_POINT('Ctrl Pts',(0.0172499203598626,0.154934638618005,
-0.373921893272926));
#80471=CARTESIAN_POINT('Ctrl Pts',(0.00688737479814154,0.15574175549937,
-0.373182574158718));
#80472=CARTESIAN_POINT('Ctrl Pts',(-0.0034603217118658,0.155511506563503,
-0.372443255044511));
#80473=CARTESIAN_POINT('Ctrl Pts',(-0.013759914147707,0.155282328002272,
-0.371707372855755));
#80474=CARTESIAN_POINT('Ctrl Pts',(-0.024043862791822,0.154025424734984,
-0.370971490666999));
#80475=CARTESIAN_POINT('Ctrl Pts',(-0.0340955737290129,0.151767237413381,
-0.370235608478243));
#80476=CARTESIAN_POINT('Ctrl Pts',(-0.0442177041878638,0.149493229852616,
-0.36949457090131));
#80477=CARTESIAN_POINT('Ctrl Pts',(-0.0541034007564343,0.146204049606232,
-0.368753533324376));
#80478=CARTESIAN_POINT('Ctrl Pts',(-0.0635449458789444,0.141978316489674,
-0.368012495747443));
#80479=CARTESIAN_POINT('Ctrl Pts',(-0.0729864910014544,0.137752583373116,
-0.367271458170509));
#80480=CARTESIAN_POINT('Ctrl Pts',(-0.0819830759570848,0.132590800628203,
-0.366530420593576));
#80481=CARTESIAN_POINT('Ctrl Pts',(-0.0903535391157341,0.126617694139727,
-0.365789383016643));
#80482=CARTESIAN_POINT('Ctrl Pts',(-0.0986278299880834,0.120713215551097,
-0.365056859577655));
#80483=CARTESIAN_POINT('Ctrl Pts',(-0.106353689299282,0.113970697276645,
-0.364324336138668));
#80484=CARTESIAN_POINT('Ctrl Pts',(-0.113357974871389,0.106516534083012,
-0.363591812699681));
#80485=CARTESIAN_POINT('Ctrl Pts',(-0.120352862561989,0.0990723723865641,
-0.362860272111609));
#80486=CARTESIAN_POINT('Ctrl Pts',(-0.126627387258907,0.090919072982288,
-0.362128731523536));
#80487=CARTESIAN_POINT('Ctrl Pts',(-0.132043043414792,0.0822218777805478,
-0.361397190935464));
#80488=CARTESIAN_POINT('Ctrl Pts',(-0.137453576521634,0.0735329098658196,
-0.360666342362948));
#80489=CARTESIAN_POINT('Ctrl Pts',(-0.14200634180813,0.0643018565896784,
-0.359935493790432));
#80490=CARTESIAN_POINT('Ctrl Pts',(-0.145606530111015,0.0547223984217612,
-0.359204645217917));
#80491=CARTESIAN_POINT('Ctrl Pts',(-0.149215067776358,0.0451207240913367,
-0.358472101700825));
#80492=CARTESIAN_POINT('Ctrl Pts',(-0.151866301606515,0.0351699238834797,
-0.357739558183735));
#80493=CARTESIAN_POINT('Ctrl Pts',(-0.153514574585645,0.0250814251945219,
-0.357007014666644));
#80494=CARTESIAN_POINT('Ctrl Pts',(-0.154874093797856,0.0167602866673107,
-0.356402802258944));
#80495=CARTESIAN_POINT('Ctrl Pts',(-0.155552210956479,0.00834601538551534,
-0.355798589851245));
#80496=CARTESIAN_POINT('Ctrl Pts',(-0.155549994568677,-4.11057744457694E-5,
-0.355194377443546));
#80497=CARTESIAN_POINT('',(-0.155549931546106,-0.000109021168048467,-0.369108945921202));
#80498=CARTESIAN_POINT('Ctrl Pts',(0.102342226162682,0.117140391172586,
-0.39458065504025));
#80499=CARTESIAN_POINT('Ctrl Pts',(0.0990436577238993,0.120022256546226,
-0.394287763136437));
#80500=CARTESIAN_POINT('Ctrl Pts',(0.0956231589673669,0.122764977425907,
-0.393991420093704));
#80501=CARTESIAN_POINT('Ctrl Pts',(0.0903485245596155,0.126639696980803,
-0.393540936964394));
#80502=CARTESIAN_POINT('Ctrl Pts',(0.0885812435961712,0.12788209903274,
-0.393391038034195));
#80503=CARTESIAN_POINT('Ctrl Pts',(0.0856385464428394,0.129860551344907,
-0.393142714453109));
#80504=CARTESIAN_POINT('Ctrl Pts',(0.0844781070580761,0.130618423819413,
-0.393045105112036));
#80505=CARTESIAN_POINT('Ctrl Pts',(0.0823574844704538,0.131963303171459,
-0.392867204059805));
#80506=CARTESIAN_POINT('Ctrl Pts',(0.0814007533674989,0.132555595364566,
-0.39278711387893));
#80507=CARTESIAN_POINT('Ctrl Pts',(0.0793171639663523,0.133814438430755,
-0.392613009675623));
#80508=CARTESIAN_POINT('Ctrl Pts',(0.078188155400012,0.134477241918941,
-0.392518867438061));
#80509=CARTESIAN_POINT('Ctrl Pts',(0.07498842592508,0.136301781505302,-0.392252530350849));
#80510=CARTESIAN_POINT('Ctrl Pts',(0.0728993597881388,0.137430425535494,
-0.392079184460036));
#80511=CARTESIAN_POINT('Ctrl Pts',(0.0635335214936542,0.142216800621858,
-0.391303966956571));
#80512=CARTESIAN_POINT('Ctrl Pts',(0.0560029286093983,0.145347038301092,
-0.390684794156728));
#80513=CARTESIAN_POINT('Ctrl Pts',(0.0395855453188601,0.15070536664108,
-0.389352105625249));
#80514=CARTESIAN_POINT('Ctrl Pts',(0.0306754390533624,0.152768287796585,
-0.388638622687398));
#80515=CARTESIAN_POINT('Ctrl Pts',(0.0188869811684354,0.154424054806561,
-0.387737018241808));
#80516=CARTESIAN_POINT('Ctrl Pts',(0.0161282484375128,0.154736513865307,
-0.387529097745903));
#80517=CARTESIAN_POINT('Ctrl Pts',(0.012369643410878,0.155060592593653,
-0.38725120623545));
#80518=CARTESIAN_POINT('Ctrl Pts',(0.0113760217546522,0.155136654989613,
-0.387178253388668));
#80519=CARTESIAN_POINT('Ctrl Pts',(0.00978805789541216,0.155242875568239,
-0.387062548268217));
#80520=CARTESIAN_POINT('Ctrl Pts',(0.00919417575328183,0.155279179725827,
-0.387019473160543));
#80521=CARTESIAN_POINT('Ctrl Pts',(0.00792951129614141,0.155349207917511,
-0.386928185776871));
#80522=CARTESIAN_POINT('Ctrl Pts',(0.00725868685187888,0.155381997211835,
-0.386880027570973));
#80523=CARTESIAN_POINT('Ctrl Pts',(0.00553778242150198,0.155454944210573,
-0.386757112616538));
#80524=CARTESIAN_POINT('Ctrl Pts',(0.00448744754675826,0.155488808882294,
-0.38668269210849));
#80525=CARTESIAN_POINT('Ctrl Pts',(-8.07190659825778E-5,0.155589765267076,
-0.386361306897857));
#80526=CARTESIAN_POINT('Ctrl Pts',(-0.00360020104933071,0.155548142426236,
-0.386119590138954));
#80527=CARTESIAN_POINT('Ctrl Pts',(-0.0143271742175793,0.15505692897941,
-0.385392607819279));
#80528=CARTESIAN_POINT('Ctrl Pts',(-0.0215075612017889,0.154225024524725,
-0.384919135256757));
#80529=CARTESIAN_POINT('Ctrl Pts',(-0.0375912449433175,0.15121602819075,
-0.383841136058655));
#80530=CARTESIAN_POINT('Ctrl Pts',(-0.0464111308382953,0.148745987082825,
-0.383236715655148));
#80531=CARTESIAN_POINT('Ctrl Pts',(-0.0569893384070287,0.144750515467279,
-0.382458484074722));
#80532=CARTESIAN_POINT('Ctrl Pts',(-0.0589998242090271,0.14394275384838,
-0.382308152321243));
#80533=CARTESIAN_POINT('Ctrl Pts',(-0.0622693977844241,0.142549116734279,
-0.382059262538946));
#80534=CARTESIAN_POINT('Ctrl Pts',(-0.0635387135022984,0.141987887682433,
-0.38196152639137));
#80535=CARTESIAN_POINT('Ctrl Pts',(-0.0658233426026664,0.140940967878594,
-0.381783492496763));
#80536=CARTESIAN_POINT('Ctrl Pts',(-0.0668412282902948,0.14046109403529,
-0.381703397751886));
#80537=CARTESIAN_POINT('Ctrl Pts',(-0.0690305245835815,0.139399782213281,
-0.381529396467118));
#80538=CARTESIAN_POINT('Ctrl Pts',(-0.0701999806319685,0.138814535017395,
-0.381435362918814));
#80539=CARTESIAN_POINT('Ctrl Pts',(-0.0734651460869936,0.137128690553749,
-0.381169664662358));
#80540=CARTESIAN_POINT('Ctrl Pts',(-0.0755432311339703,0.135994943136918,
-0.380996857790056));
#80541=CARTESIAN_POINT('Ctrl Pts',(-0.0846034272654175,0.130780200743782,
-0.38022645054959));
#80542=CARTESIAN_POINT('Ctrl Pts',(-0.0912859822725921,0.126206314224676,
-0.379611803845602));
#80543=CARTESIAN_POINT('Ctrl Pts',(-0.104600923792216,0.115480243469031,
-0.378292636901898));
#80544=CARTESIAN_POINT('Ctrl Pts',(-0.11111530560378,0.109226538509883,
-0.377588205168478));
#80545=CARTESIAN_POINT('Ctrl Pts',(-0.118974670922404,0.100246478885924,
-0.376683087222946));
#80546=CARTESIAN_POINT('Ctrl Pts',(-0.120835654242549,0.0979952867029918,
-0.376464083483152));
#80547=CARTESIAN_POINT('Ctrl Pts',(-0.123256753588523,0.0948926001915009,
-0.3761740456901));
#80548=CARTESIAN_POINT('Ctrl Pts',(-0.123873391639172,0.0940862150702452,
-0.376099700640623));
#80549=CARTESIAN_POINT('Ctrl Pts',(-0.124840921635155,0.0927949612724498,
-0.375982360741999));
#80550=CARTESIAN_POINT('Ctrl Pts',(-0.125196972401435,0.092314022154407,
-0.375939027030337));
#80551=CARTESIAN_POINT('Ctrl Pts',(-0.125944168409434,0.0912924650202418,
-0.375847783525183));
#80552=CARTESIAN_POINT('Ctrl Pts',(-0.126334628020549,0.0907513610036011,
-0.375799923285292));
#80553=CARTESIAN_POINT('Ctrl Pts',(-0.127319037323205,0.0893684873260986,
-0.375678752510074));
#80554=CARTESIAN_POINT('Ctrl Pts',(-0.127908142124847,0.0885232801066856,
-0.375605759611428));
#80555=CARTESIAN_POINT('Ctrl Pts',(-0.13035514298136,0.0849370568688732,
-0.375300222864133));
#80556=CARTESIAN_POINT('Ctrl Pts',(-0.132133810621604,0.0821427223688853,
-0.375072307040431));
#80557=CARTESIAN_POINT('Ctrl Pts',(-0.139060122653014,0.0704533237310836,
-0.37415043720196));
#80558=CARTESIAN_POINT('Ctrl Pts',(-0.143409704206191,0.0611152806725299,
-0.373485179801227));
#80559=CARTESIAN_POINT('Ctrl Pts',(-0.149188600306762,0.0446149124210833,
-0.372326264867267));
#80560=CARTESIAN_POINT('Ctrl Pts',(-0.151094752297982,0.0376574724873536,
-0.371842494210479));
#80561=CARTESIAN_POINT('Ctrl Pts',(-0.152891690232485,0.0286995658878011,
-0.371209412667761));
#80562=CARTESIAN_POINT('Ctrl Pts',(-0.153236290544166,0.0267987446228151,
-0.371074544120154));
#80563=CARTESIAN_POINT('Ctrl Pts',(-0.1537402154161,0.0236903111726044,
-0.370852865714455));
#80564=CARTESIAN_POINT('Ctrl Pts',(-0.153920918368918,0.0224863384572335,
-0.370766731333539));
#80565=CARTESIAN_POINT('Ctrl Pts',(-0.154235002444943,0.0202121132415971,
-0.370603454356239));
#80566=CARTESIAN_POINT('Ctrl Pts',(-0.154371421961385,0.0191423476949558,
-0.37052641230921));
#80567=CARTESIAN_POINT('Ctrl Pts',(-0.154626313842322,0.0169632011293798,
-0.370368952586842));
#80568=CARTESIAN_POINT('Ctrl Pts',(-0.154743995850993,0.0158537930265916,
-0.370288514897042));
#80569=CARTESIAN_POINT('Ctrl Pts',(-0.155045129489924,0.0126909564207269,
-0.370058366089622));
#80570=CARTESIAN_POINT('Ctrl Pts',(-0.155199699647872,0.0106350850549925,
-0.369907773453013));
#80571=CARTESIAN_POINT('Ctrl Pts',(-0.155473109177032,0.00568405776425027,
-0.369542574006086));
#80572=CARTESIAN_POINT('Ctrl Pts',(-0.155551995357722,0.00278758824431477,
-0.369326834733086));
#80573=CARTESIAN_POINT('Ctrl Pts',(-0.155549961666794,-0.000109203749030585,
-0.369108984688673));
#80574=CARTESIAN_POINT('Ctrl Pts',(-0.155549961792102,-0.00010902511433882,
-0.369108998122695));
#80575=CARTESIAN_POINT('Ctrl Pts',(-0.155542653148416,-0.0105365238885239,
-0.368324809893432));
#80576=CARTESIAN_POINT('Ctrl Pts',(-0.15448680998581,-0.0209362629403968,
-0.367513221839129));
#80577=CARTESIAN_POINT('Ctrl Pts',(-0.151223083365885,-0.0369033025256532,
-0.366253479600695));
#80578=CARTESIAN_POINT('Ctrl Pts',(-0.149722407424921,-0.0425850820425572,
-0.365803003141355));
#80579=CARTESIAN_POINT('Ctrl Pts',(-0.147434623044069,-0.0496097853025308,
-0.365252855596421));
#80580=CARTESIAN_POINT('Ctrl Pts',(-0.146944304424871,-0.0510438117500759,
-0.365140926057862));
#80581=CARTESIAN_POINT('Ctrl Pts',(-0.146173516486474,-0.0531949029040052,
-0.364973830280732));
#80582=CARTESIAN_POINT('Ctrl Pts',(-0.145908570677525,-0.0539173783381018,
-0.364917846756262));
#80583=CARTESIAN_POINT('Ctrl Pts',(-0.145414988546055,-0.055233030569196,
-0.364816189164675));
#80584=CARTESIAN_POINT('Ctrl Pts',(-0.145188069653475,-0.0558267948138428,
-0.364770423047617));
#80585=CARTESIAN_POINT('Ctrl Pts',(-0.144661198834578,-0.0571804810871024,
-0.364666328478205));
#80586=CARTESIAN_POINT('Ctrl Pts',(-0.144358892602902,-0.0579394517623867,
-0.364608138578518));
#80587=CARTESIAN_POINT('Ctrl Pts',(-0.14336612934982,-0.0603758713943324,
-0.364421787290871));
#80588=CARTESIAN_POINT('Ctrl Pts',(-0.142652276322684,-0.0620437078753656,
-0.36429490905641));
#80589=CARTESIAN_POINT('Ctrl Pts',(-0.137233938959937,-0.0741147869673015,
-0.36337894392607));
#80590=CARTESIAN_POINT('Ctrl Pts',(-0.131425327857237,-0.0839857652447746,
-0.362640696120224));
#80591=CARTESIAN_POINT('Ctrl Pts',(-0.121383113407584,-0.0974196486601801,
-0.361531852553697));
#80592=CARTESIAN_POINT('Ctrl Pts',(-0.117959703263889,-0.101537924356356,
-0.361175471631034));
#80593=CARTESIAN_POINT('Ctrl Pts',(-0.112656087883774,-0.10728704729976,
-0.360644251882682));
#80594=CARTESIAN_POINT('Ctrl Pts',(-0.11093818388441,-0.109062472791636,
-0.36047508461122));
#80595=CARTESIAN_POINT('Ctrl Pts',(-0.107749454920902,-0.112204653810063,
-0.360165417271889));
#80596=CARTESIAN_POINT('Ctrl Pts',(-0.10629304237743,-0.113585289009196,
-0.360025524307564));
#80597=CARTESIAN_POINT('Ctrl Pts',(-0.10475027792264,-0.114992123175167,
-0.359878721077568));
#80598=CARTESIAN_POINT('Ctrl Pts',(-0.104690127592689,-0.115046887405898,
-0.359872999568864));
#80599=CARTESIAN_POINT('Ctrl Pts',(-0.104571434833511,-0.115154781780456,
-0.35986171371752));
#80600=CARTESIAN_POINT('Ctrl Pts',(-0.104512894798335,-0.115207914532271,
-0.359856149483805));
#80601=CARTESIAN_POINT('Ctrl Pts',(-0.104396606719464,-0.115313299625932,
-0.359845100284993));
#80602=CARTESIAN_POINT('Ctrl Pts',(-0.104338859887233,-0.115365553275455,
-0.359839615375602));
#80603=CARTESIAN_POINT('Ctrl Pts',(-0.104223327877295,-0.115469937572198,
-0.359828645790369));
#80604=CARTESIAN_POINT('Ctrl Pts',(-0.10416554277042,-0.115522068264251,
-0.359823161118577));
#80605=CARTESIAN_POINT('Ctrl Pts',(-0.104049041172718,-0.115627011410977,
-0.359812107249289));
#80606=CARTESIAN_POINT('Ctrl Pts',(-0.103990323539663,-0.115679822557228,
-0.359806538000588));
#80607=CARTESIAN_POINT('Ctrl Pts',(-0.103870938541682,-0.115787034103212,
-0.359795218576086));
#80608=CARTESIAN_POINT('Ctrl Pts',(-0.103810268603674,-0.11584143158791,
-0.359789468283536));
#80609=CARTESIAN_POINT('Ctrl Pts',(-0.103685746681135,-0.11595290323976,
-0.359777670377251));
#80610=CARTESIAN_POINT('Ctrl Pts',(-0.103621890260409,-0.116009972387555,
-0.359771622561006));
#80611=CARTESIAN_POINT('Ctrl Pts',(-0.103489413391929,-0.116128171696093,
-0.359759080469007));
#80612=CARTESIAN_POINT('Ctrl Pts',(-0.103420785852836,-0.116189293823484,
-0.359752585868001));
#80613=CARTESIAN_POINT('Ctrl Pts',(-0.103276611891727,-0.11631747134407,
-0.359738947381961));
#80614=CARTESIAN_POINT('Ctrl Pts',(-0.103201054265141,-0.116384514013635,
-0.359731802980783));
#80615=CARTESIAN_POINT('Ctrl Pts',(-0.103082980207387,-0.116489076341719,
-0.359720643304648));
#80616=CARTESIAN_POINT('Ctrl Pts',(-0.103040508365672,-0.116526646528217,
-0.359716630099068));
#80617=CARTESIAN_POINT('Ctrl Pts',(-0.102887193138994,-0.116662118354606,
-0.359702146741765));
#80618=CARTESIAN_POINT('Ctrl Pts',(-0.102776230987178,-0.116759884869776,
-0.359691671072001));
#80619=CARTESIAN_POINT('Ctrl Pts',(-0.101872250324765,-0.117554076923857,
-0.359606382287122));
#80620=CARTESIAN_POINT('Ctrl Pts',(-0.101072320041888,-0.118242557521096,
-0.35953124684217));
#80621=CARTESIAN_POINT('Ctrl Pts',(-0.0992683042712271,-0.119763547879234,
-0.359362503688229));
#80622=CARTESIAN_POINT('Ctrl Pts',(-0.0982606396411751,-0.120591666958241,
-0.35926872546181));
#80623=CARTESIAN_POINT('Ctrl Pts',(-0.0954584838310542,-0.122836094655481,
-0.359009163135727));
#80624=CARTESIAN_POINT('Ctrl Pts',(-0.0936430651259912,-0.124225615786324,
-0.358842345334207));
#80625=CARTESIAN_POINT('Ctrl Pts',(-0.0825803194243243,-0.132312726648769,
-0.357833172999869));
#80626=CARTESIAN_POINT('Ctrl Pts',(-0.0726506007022807,-0.138014361313446,
-0.356953777414982));
#80627=CARTESIAN_POINT('Ctrl Pts',(-0.0570041682774519,-0.144838952004175,
-0.355630933133603));
#80628=CARTESIAN_POINT('Ctrl Pts',(-0.0516997333702246,-0.146816013035286,
-0.355193016087507));
#80629=CARTESIAN_POINT('Ctrl Pts',(-0.0433711088026882,-0.149412704096979,
-0.354530721261272));
#80630=CARTESIAN_POINT('Ctrl Pts',(-0.0404164722410028,-0.150238880127184,
-0.354300543782726));
#80631=CARTESIAN_POINT('Ctrl Pts',(-0.0364647364669028,-0.151218825785667,
-0.354000578153947));
#80632=CARTESIAN_POINT('Ctrl Pts',(-0.0354880160944418,-0.151451018923379,
-0.353927070777786));
#80633=CARTESIAN_POINT('Ctrl Pts',(-0.0338637287992436,-0.151820579674609,
-0.353805950541589));
#80634=CARTESIAN_POINT('Ctrl Pts',(-0.0332174232508073,-0.151963296206719,
-0.353758050249479));
#80635=CARTESIAN_POINT('Ctrl Pts',(-0.0319802285685722,-0.152228221795555,
-0.353666941481153));
#80636=CARTESIAN_POINT('Ctrl Pts',(-0.0313895104195222,-0.15235112470573,
-0.353623692283379));
#80637=CARTESIAN_POINT('Ctrl Pts',(-0.029777191571018,-0.15267680274454,
-0.353506295921824));
#80638=CARTESIAN_POINT('Ctrl Pts',(-0.0287542224859087,-0.152872764346402,
-0.353432519753503));
#80639=CARTESIAN_POINT('Ctrl Pts',(-0.0246413713855004,-0.153617882264129,
-0.353138455034306));
#80640=CARTESIAN_POINT('Ctrl Pts',(-0.0215369327324756,-0.154083791293826,
-0.352922250454496));
#80641=CARTESIAN_POINT('Ctrl Pts',(-0.00963984795243291,-0.155502630997381,
-0.352108250244894));
#80642=CARTESIAN_POINT('Ctrl Pts',(-0.000785440330262356,-0.155799239028749,
-0.35153184413112));
#80643=CARTESIAN_POINT('Ctrl Pts',(0.0160374348858264,-0.154927806413076,
-0.350420169597972));
#80644=CARTESIAN_POINT('Ctrl Pts',(0.0239833473702748,-0.153898023917492,
-0.349887855353378));
#80645=CARTESIAN_POINT('Ctrl Pts',(0.0341206325625117,-0.151779895178607,
-0.349174649464466));
#80646=CARTESIAN_POINT('Ctrl Pts',(0.0364156590466672,-0.151245670729985,
-0.349010932925888));
#80647=CARTESIAN_POINT('Ctrl Pts',(0.0399620276865986,-0.150334770387596,
-0.34875395148283));
#80648=CARTESIAN_POINT('Ctrl Pts',(0.0412223140658205,-0.149994091493247,
-0.348661833671514));
#80649=CARTESIAN_POINT('Ctrl Pts',(0.0435608363179875,-0.149330247297556,
-0.348489344454473));
#80650=CARTESIAN_POINT('Ctrl Pts',(0.044640148570971,-0.149011161436979,
-0.348409109608831));
#80651=CARTESIAN_POINT('Ctrl Pts',(0.047045129668025,-0.148271683854432,
-0.348228875568988));
#80652=CARTESIAN_POINT('Ctrl Pts',(0.0483687993967947,-0.147845173988204,
-0.348128682903362));
#80653=CARTESIAN_POINT('Ctrl Pts',(0.05174884891782,-0.146705812922677,
-0.347870193709787));
#80654=CARTESIAN_POINT('Ctrl Pts',(0.0537962463238277,-0.145967468676788,
-0.347711080932915));
#80655=CARTESIAN_POINT('Ctrl Pts',(0.0640313780522109,-0.142031835015903,
-0.346902426588634));
#80656=CARTESIAN_POINT('Ctrl Pts',(0.0719519185206624,-0.138188043754406,
-0.346232137904868));
#80657=CARTESIAN_POINT('Ctrl Pts',(0.0859306156531535,-0.129875442579227,
-0.344974849207563));
#80658=CARTESIAN_POINT('Ctrl Pts',(0.092073040237872,-0.12559563029979,
-0.34439227034945));
#80659=CARTESIAN_POINT('Ctrl Pts',(0.0997699866967528,-0.119363483845766,
-0.343637142450146));
#80660=CARTESIAN_POINT('Ctrl Pts',(0.101620112134122,-0.117792383723186,
-0.343453577881046));
#80661=CARTESIAN_POINT('Ctrl Pts',(0.104726399546585,-0.115026881370939,
-0.343142781308017));
#80662=CARTESIAN_POINT('Ctrl Pts',(0.106000731012999,-0.113853624795944,
-0.343014492457252));
#80663=CARTESIAN_POINT('Ctrl Pts',(0.10784252430731,-0.112100177971014,
-0.342828235387536));
#80664=CARTESIAN_POINT('Ctrl Pts',(0.108425418402785,-0.111536490315506,
-0.34276916107942));
#80665=CARTESIAN_POINT('Ctrl Pts',(0.109456684545443,-0.110523479636222,
-0.34266445984756));
#80666=CARTESIAN_POINT('Ctrl Pts',(0.109906745022687,-0.110075940991269,
-0.342618705431));
#80667=CARTESIAN_POINT('Ctrl Pts',(0.110908166404592,-0.109067865296914,
-0.342516758740405));
#80668=CARTESIAN_POINT('Ctrl Pts',(0.111458031290368,-0.108505888997843,
-0.342460679630619));
#80669=CARTESIAN_POINT('Ctrl Pts',(0.113114534367614,-0.106787019441468,
-0.342291333584569));
#80670=CARTESIAN_POINT('Ctrl Pts',(0.114207636129837,-0.105617147165904,
-0.342179028347387));
#80671=CARTESIAN_POINT('Ctrl Pts',(0.12009771164027,-0.0991149995571928,
-0.341569373443823));
#80672=CARTESIAN_POINT('Ctrl Pts',(0.124540094552274,-0.0934720997648663,
-0.341092545368906));
#80673=CARTESIAN_POINT('Ctrl Pts',(0.132051587551712,-0.0824395851387343,
-0.340211365473669));
#80674=CARTESIAN_POINT('Ctrl Pts',(0.135218759772714,-0.0771348982962128,
-0.339806971979551));
#80675=CARTESIAN_POINT('Ctrl Pts',(0.140088132991576,-0.067752906633184,
-0.339104154631879));
#80676=CARTESIAN_POINT('Ctrl Pts',(0.141947379860386,-0.0637658085816957,
-0.338809087848357));
#80677=CARTESIAN_POINT('Ctrl Pts',(0.144840508881559,-0.0568057317678934,
-0.338294816194288));
#80678=CARTESIAN_POINT('Ctrl Pts',(0.145957712059494,-0.0538702904695179,
-0.338078175521387));
#80679=CARTESIAN_POINT('Ctrl Pts',(0.147460838479355,-0.0495299469889708,
-0.337757032366953));
#80680=CARTESIAN_POINT('Ctrl Pts',(0.147917137293856,-0.0481501274878945,
-0.337654824280176));
#80681=CARTESIAN_POINT('Ctrl Pts',(0.148694010371156,-0.0456855851358198,
-0.337471954782896));
#80682=CARTESIAN_POINT('Ctrl Pts',(0.149022217171528,-0.0446033639563307,
-0.337391548169827));
#80683=CARTESIAN_POINT('Ctrl Pts',(0.14969226569751,-0.0423039746789782,
-0.337220435732902));
#80684=CARTESIAN_POINT('Ctrl Pts',(0.150031125278164,-0.0410860311691848,
-0.337129639994901));
#80685=CARTESIAN_POINT('Ctrl Pts',(0.150907518066628,-0.0377805498923967,
-0.336882717647996));
#80686=CARTESIAN_POINT('Ctrl Pts',(0.151416546195022,-0.0356858184531165,
-0.336725696019932));
#80687=CARTESIAN_POINT('Ctrl Pts',(0.154623214881198,-0.0211826545236121,
-0.335634251274153));
#80688=CARTESIAN_POINT('Ctrl Pts',(0.15583553642611,-0.00849719880153343,
-0.334652288712062));
#80689=CARTESIAN_POINT('Ctrl Pts',(0.15531397539444,0.0108523768537028,
-0.33315343211067));
#80690=CARTESIAN_POINT('Ctrl Pts',(0.154706565903961,0.0174957403968025,
-0.33263991250157));
#80691=CARTESIAN_POINT('Ctrl Pts',(0.153426806796225,0.025662887203259,
-0.332023414601149));
#80692=CARTESIAN_POINT('Ctrl Pts',(0.153154362516311,0.027241706852262,
-0.331904950436275));
#80693=CARTESIAN_POINT('Ctrl Pts',(0.152711876709184,0.0295889109378865,
-0.331730165861789));
#80694=CARTESIAN_POINT('Ctrl Pts',(0.152560329467402,0.0303606140017147,
-0.331672917317838));
#80695=CARTESIAN_POINT('Ctrl Pts',(0.152288559736134,0.0316910658216855,
-0.331574630145222));
#80696=CARTESIAN_POINT('Ctrl Pts',(0.152171104159477,0.0322503359465934,
-0.331533442670949));
#80697=CARTESIAN_POINT('Ctrl Pts',(0.151886605889724,0.0335688202852624,
-0.331436644139672));
#80698=CARTESIAN_POINT('Ctrl Pts',(0.151716951205872,0.0343274457151024,
-0.331381180143353));
#80699=CARTESIAN_POINT('Ctrl Pts',(0.151190835544041,0.036599895343702,
-0.331215646391797));
#80700=CARTESIAN_POINT('Ctrl Pts',(0.150817339662266,0.0381097314066112,
-0.331106476125294));
#80701=CARTESIAN_POINT('Ctrl Pts',(0.147475092643408,0.0508008930098569,
-0.330193714210232));
#80702=CARTESIAN_POINT('Ctrl Pts',(0.143289710270429,0.0616260588405502,
-0.329445335627954));
#80703=CARTESIAN_POINT('Ctrl Pts',(0.135398109976251,0.0767687806790433,
-0.328317183312199));
#80704=CARTESIAN_POINT('Ctrl Pts',(0.132597455023029,0.0815107476335337,
-0.327951115804574));
#80705=CARTESIAN_POINT('Ctrl Pts',(0.127524281588751,0.0891446919271814,
-0.327329011072885));
#80706=CARTESIAN_POINT('Ctrl Pts',(0.125390025838851,0.0921225077589712,
-0.327077364656587));
#80707=CARTESIAN_POINT('Ctrl Pts',(0.122213151198575,0.0962398785543149,
-0.326714442097121));
#80708=CARTESIAN_POINT('Ctrl Pts',(0.121255518858464,0.097443662698613,
-0.326606430612682));
#80709=CARTESIAN_POINT('Ctrl Pts',(0.119555932733026,0.0995162608485024,
-0.326416976070397));
#80710=CARTESIAN_POINT('Ctrl Pts',(0.118821955032776,0.100391484206639,
-0.326335855864047));
#80711=CARTESIAN_POINT('Ctrl Pts',(0.117281325562466,0.102188025277145,
-0.326166956704383));
#80712=CARTESIAN_POINT('Ctrl Pts',(0.116473302885723,0.103108056876523,
-0.326079125046549));
#80713=CARTESIAN_POINT('Ctrl Pts',(0.114340211832302,0.105479767645434,
-0.325849126929599));
#80714=CARTESIAN_POINT('Ctrl Pts',(0.112998379782944,0.106915999448697,
-0.325706266327592));
#80715=CARTESIAN_POINT('Ctrl Pts',(0.108654866342163,0.11139196732859,-0.32524927132002));
#80716=CARTESIAN_POINT('Ctrl Pts',(0.105556299437616,0.114332346488649,
-0.324931146127184));
#80717=CARTESIAN_POINT('Ctrl Pts',(0.102342232991206,0.117140385206698,
-0.324608715049314));
#80718=CARTESIAN_POINT('Origin',(0.,0.,-1.10400562256037));
#80719=CARTESIAN_POINT('',(0.102342242837721,0.117140376604077,-0.240688435831897));
#80720=CARTESIAN_POINT('',(0.102342242833752,0.117140376607545,-0.254368055082067));
#80721=CARTESIAN_POINT('',(0.10234224283772,0.117140376604078,-1.10400562256037));
#80722=CARTESIAN_POINT('',(-0.155549938814025,0.00013796721713873,-0.285194377443525));
#80723=CARTESIAN_POINT('Ctrl Pts',(-0.155549938814074,0.000137967162685264,
-0.285194377439629));
#80724=CARTESIAN_POINT('Ctrl Pts',(-0.155558981668482,-0.010057324401557,
-0.284464910207374));
#80725=CARTESIAN_POINT('Ctrl Pts',(-0.154561332613283,-0.0202748323328174,
-0.283735442975119));
#80726=CARTESIAN_POINT('Ctrl Pts',(-0.152570315678244,-0.0303001860364103,
-0.283005975742864));
#80727=CARTESIAN_POINT('Ctrl Pts',(-0.150580816435515,-0.0403178977144842,
-0.282277064561534));
#80728=CARTESIAN_POINT('Ctrl Pts',(-0.147599629776064,-0.0501428167204543,
-0.281548153380204));
#80729=CARTESIAN_POINT('Ctrl Pts',(-0.143691318078789,-0.0595701906055402,
-0.280819242198874));
#80730=CARTESIAN_POINT('Ctrl Pts',(-0.139773730282771,-0.0690199396893853,
-0.280088600998903));
#80731=CARTESIAN_POINT('Ctrl Pts',(-0.134925019610267,-0.0780693952167697,
-0.279357959798932));
#80732=CARTESIAN_POINT('Ctrl Pts',(-0.129257441688844,-0.0865350580288423,
-0.27862731859896));
#80733=CARTESIAN_POINT('Ctrl Pts',(-0.125342359471028,-0.0923830174917879,
-0.278122602049974));
#80734=CARTESIAN_POINT('Ctrl Pts',(-0.12103754189237,-0.0979528910724632,
-0.277617885500988));
#80735=CARTESIAN_POINT('Ctrl Pts',(-0.116391161322095,-0.103193507867957,
-0.277113168952002));
#80736=CARTESIAN_POINT('Ctrl Pts',(-0.109601189038108,-0.110851865218201,
-0.276375603157067));
#80737=CARTESIAN_POINT('Ctrl Pts',(-0.102026882713366,-0.117865655153864,
-0.275638037362132));
#80738=CARTESIAN_POINT('Ctrl Pts',(-0.0938147346389066,-0.124074969533067,
-0.274900471567197));
#80739=CARTESIAN_POINT('Ctrl Pts',(-0.0855830648899174,-0.130299044510017,
-0.274161152452757));
#80740=CARTESIAN_POINT('Ctrl Pts',(-0.0767111678007134,-0.13571413733421,
-0.273421833338317));
#80741=CARTESIAN_POINT('Ctrl Pts',(-0.0673824449105403,-0.14019774826251,
-0.272682514223878));
#80742=CARTESIAN_POINT('Ctrl Pts',(-0.05809708913432,-0.144660515901933,
-0.271946632036085));
#80743=CARTESIAN_POINT('Ctrl Pts',(-0.0483599847136722,-0.148200036035695,
-0.271210749848292));
#80744=CARTESIAN_POINT('Ctrl Pts',(-0.0383761940370499,-0.150741733541945,
-0.2704748676605));
#80745=CARTESIAN_POINT('Ctrl Pts',(-0.0283224596450145,-0.153301237487933,
-0.269733830082737));
#80746=CARTESIAN_POINT('Ctrl Pts',(-0.0180194862842248,-0.154848636445333,
-0.268992792504974));
#80747=CARTESIAN_POINT('Ctrl Pts',(-0.00768806758017188,-0.155359892240188,
-0.268251754927211));
#80748=CARTESIAN_POINT('Ctrl Pts',(0.0026433511238818,-0.155871148035042,
-0.267510717349448));
#80749=CARTESIAN_POINT('Ctrl Pts',(0.0130022662074183,-0.155346342822456,
-0.266769679771685));
#80750=CARTESIAN_POINT('Ctrl Pts',(0.023170665058325,-0.153814572719086,
-0.266028642193922));
#80751=CARTESIAN_POINT('Ctrl Pts',(0.0332914247445106,-0.152289978991203,
-0.265291076392959));
#80752=CARTESIAN_POINT('Ctrl Pts',(0.0432986755703804,-0.149756542950667,
-0.264553510591997));
#80753=CARTESIAN_POINT('Ctrl Pts',(0.0529785256937023,-0.146250054069466,
-0.263815944791035));
#80754=CARTESIAN_POINT('Ctrl Pts',(0.0626813863702148,-0.142735229702913,
-0.263076625678102));
#80755=CARTESIAN_POINT('Ctrl Pts',(0.0720543656097244,-0.138242897588601,
-0.262337306565169));
#80756=CARTESIAN_POINT('Ctrl Pts',(0.0808948481806159,-0.132860174762173,
-0.261597987452237));
#80757=CARTESIAN_POINT('Ctrl Pts',(0.0896942334457746,-0.127502474936909,
-0.260862105258429));
#80758=CARTESIAN_POINT('Ctrl Pts',(0.0979652636911245,-0.121263126769864,
-0.26012622306462));
#80759=CARTESIAN_POINT('Ctrl Pts',(0.105533724046101,-0.114273512193165,
-0.259390340870812));
#80760=CARTESIAN_POINT('Ctrl Pts',(0.11315520685431,-0.107234930390026,
-0.258649303298317));
#80761=CARTESIAN_POINT('Ctrl Pts',(0.120063530842511,-0.0994361637182063,
-0.257908265725822));
#80762=CARTESIAN_POINT('Ctrl Pts',(0.126118301512676,-0.0910493081992267,
-0.257167228153327));
#80763=CARTESIAN_POINT('Ctrl Pts',(0.132173072182841,-0.0826624526802466,
-0.256426190580832));
#80764=CARTESIAN_POINT('Ctrl Pts',(0.137373841683401,-0.07368834897487,
-0.255685153008337));
#80765=CARTESIAN_POINT('Ctrl Pts',(0.141626295177241,-0.0643256948222792,
-0.254944115435842));
#80766=CARTESIAN_POINT('Ctrl Pts',(0.145858825795763,-0.0550069049921559,
-0.254206549647149));
#80767=CARTESIAN_POINT('Ctrl Pts',(0.149183400078978,-0.0452339540653752,
-0.253468983858457));
#80768=CARTESIAN_POINT('Ctrl Pts',(0.151513561061112,-0.0352057284341728,
-0.252731418069765));
#80769=CARTESIAN_POINT('Ctrl Pts',(0.153849261257435,-0.0251536638965008,
-0.251992098953765));
#80770=CARTESIAN_POINT('Ctrl Pts',(0.155185460769777,-0.0148459793914166,
-0.251252779837765));
#80771=CARTESIAN_POINT('Ctrl Pts',(0.15548489321086,-0.00450005368940009,
-0.250513460721764));
#80772=CARTESIAN_POINT('Ctrl Pts',(0.155782933655481,0.0057977760483914,
-0.249777578539952));
#80773=CARTESIAN_POINT('Ctrl Pts',(0.155053794881369,0.0161325600513416,
-0.24904169635814));
#80774=CARTESIAN_POINT('Ctrl Pts',(0.153312802145975,0.0262866353523834,
-0.248305814176328));
#80775=CARTESIAN_POINT('Ctrl Pts',(0.151559612463294,0.0365118474931549,
-0.247564776593234));
#80776=CARTESIAN_POINT('Ctrl Pts',(0.148780483665354,0.0465528707681876,
-0.246823739010139));
#80777=CARTESIAN_POINT('Ctrl Pts',(0.14504330595665,0.0561982374916302,
-0.246082701427045));
#80778=CARTESIAN_POINT('Ctrl Pts',(0.141306128247946,0.0658436042150729,
-0.24534166384395));
#80779=CARTESIAN_POINT('Ctrl Pts',(0.136611362837868,0.0750924809795906,
-0.244600626260856));
#80780=CARTESIAN_POINT('Ctrl Pts',(0.131074304207541,0.083757562503389,
-0.243859588677762));
#80781=CARTESIAN_POINT('Ctrl Pts',(0.12556327654748,0.0923819075108227,
-0.243122034880659));
#80782=CARTESIAN_POINT('Ctrl Pts',(0.119176932545119,0.100492053151117,
-0.242384481083557));
#80783=CARTESIAN_POINT('Ctrl Pts',(0.112034997693936,0.107907190639548,
-0.241646927286454));
#80784=CARTESIAN_POINT('Ctrl Pts',(0.108941219517684,0.11111931606685,-0.241327430134935));
#80785=CARTESIAN_POINT('Ctrl Pts',(0.105706230923814,0.11420135510192,-0.241007932983416));
#80786=CARTESIAN_POINT('Ctrl Pts',(0.102342242837721,0.117140376604077,
-0.240688435831897));
#80787=CARTESIAN_POINT('Ctrl Pts',(0.102342242837719,0.117140376604078,
-0.310696206146068));
#80788=CARTESIAN_POINT('Ctrl Pts',(0.101193397674604,0.118144090217394,
-0.310586387172793));
#80789=CARTESIAN_POINT('Ctrl Pts',(0.10003037851299,0.119130383226153,-0.310476568199517));
#80790=CARTESIAN_POINT('Ctrl Pts',(0.0988537724225576,0.120098851692384,
-0.310366749226242));
#80791=CARTESIAN_POINT('Ctrl Pts',(0.0909514548046981,0.126603276142732,
-0.309629183430565));
#80792=CARTESIAN_POINT('Ctrl Pts',(0.0823750481708025,0.132348588583837,
-0.308891617634889));
#80793=CARTESIAN_POINT('Ctrl Pts',(0.0732942129935362,0.137199711521775,
-0.308154051839212));
#80794=CARTESIAN_POINT('Ctrl Pts',(0.0641917911359939,0.142062366398989,
-0.307414732724958));
#80795=CARTESIAN_POINT('Ctrl Pts',(0.0545832879531424,0.146026008005004,
-0.306675413610704));
#80796=CARTESIAN_POINT('Ctrl Pts',(0.0446689805157271,0.148998270727165,
-0.305936094496449));
#80797=CARTESIAN_POINT('Ctrl Pts',(0.034800762428978,0.151956716078851,
-0.305200212307883));
#80798=CARTESIAN_POINT('Ctrl Pts',(0.0246304694614635,0.153932708599576,
-0.304464330119317));
#80799=CARTESIAN_POINT('Ctrl Pts',(0.0143722920902381,0.154884601300687,
-0.303728447930751));
#80800=CARTESIAN_POINT('Ctrl Pts',(0.00404224874535361,0.155843162700663,
-0.302987410353653));
#80801=CARTESIAN_POINT('Ctrl Pts',(-0.00637597069568843,0.155763118524284,
-0.302246372776555));
#80802=CARTESIAN_POINT('Ctrl Pts',(-0.0166605270868574,0.154655194989331,
-0.301505335199457));
#80803=CARTESIAN_POINT('Ctrl Pts',(-0.0269450834780264,0.153547271454379,
-0.300764297622359));
#80804=CARTESIAN_POINT('Ctrl Pts',(-0.0370950523170257,0.151411697858038,
-0.30002326004526));
#80805=CARTESIAN_POINT('Ctrl Pts',(-0.0468996365405047,0.1483112490419,
-0.299282222468162));
#80806=CARTESIAN_POINT('Ctrl Pts',(-0.0566582860298873,0.145225325909738,
-0.298544656671538));
#80807=CARTESIAN_POINT('Ctrl Pts',(-0.066147320962248,0.141160651001074,
-0.297807090874913));
#80808=CARTESIAN_POINT('Ctrl Pts',(-0.0751610594652361,0.136185967118728,
-0.297069525078289));
#80809=CARTESIAN_POINT('Ctrl Pts',(-0.08419622513386,0.131199457579858,
-0.296330205964271));
#80810=CARTESIAN_POINT('Ctrl Pts',(-0.0927529485620364,0.125298926055274,
-0.295590886850254));
#80811=CARTESIAN_POINT('Ctrl Pts',(-0.100644699324042,0.118602053093415,
-0.294851567736237));
#80812=CARTESIAN_POINT('Ctrl Pts',(-0.108499763151951,0.111936312353595,
-0.294115685546729));
#80813=CARTESIAN_POINT('Ctrl Pts',(-0.115695310022657,0.104482218782449,
-0.29337980335722));
#80814=CARTESIAN_POINT('Ctrl Pts',(-0.122079772151376,0.0963967412907104,
-0.292643921167712));
#80815=CARTESIAN_POINT('Ctrl Pts',(-0.128508962053125,0.0882546191835279,
-0.29190288359144));
#80816=CARTESIAN_POINT('Ctrl Pts',(-0.134115059660229,0.0794729694098018,
-0.291161846015168));
#80817=CARTESIAN_POINT('Ctrl Pts',(-0.138786259034236,0.0702436958259034,
-0.290420808438897));
#80818=CARTESIAN_POINT('Ctrl Pts',(-0.143457458408242,0.0610144222420051,
-0.289679770862625));
#80819=CARTESIAN_POINT('Ctrl Pts',(-0.147193448430352,0.0513384251183174,
-0.288938733286353));
#80820=CARTESIAN_POINT('Ctrl Pts',(-0.149932090804099,0.0414266900332545,
-0.288197695710081));
#80821=CARTESIAN_POINT('Ctrl Pts',(-0.153348034962215,0.0290636542878144,
-0.287273389928547));
#80822=CARTESIAN_POINT('Ctrl Pts',(-0.155235267497647,0.0162607764979687,
-0.286349084147013));
#80823=CARTESIAN_POINT('Ctrl Pts',(-0.155513782640199,0.00335647269272036,
-0.285424778365478));
#80824=CARTESIAN_POINT('Ctrl Pts',(-0.155536924385028,0.0022842577204016,
-0.28534797805816));
#80825=CARTESIAN_POINT('Ctrl Pts',(-0.15554898675718,0.00121135542526031,
-0.285271177750843));
#80826=CARTESIAN_POINT('Ctrl Pts',(-0.155549938814025,0.00013796721713873,
-0.285194377443525));
#80827=CARTESIAN_POINT('Ctrl Pts',(0.102342232991206,0.117140385206698,
-0.324608715049314));
#80828=CARTESIAN_POINT('Ctrl Pts',(0.0995774578652578,0.119555890837902,
-0.324331356308046));
#80829=CARTESIAN_POINT('Ctrl Pts',(0.0967272170089489,0.121873470857469,
-0.324050827145225));
#80830=CARTESIAN_POINT('Ctrl Pts',(0.0881603394717722,0.128349042152045,
-0.323224633791954));
#80831=CARTESIAN_POINT('Ctrl Pts',(0.082240427910377,0.132220387384085,
-0.322674244551114));
#80832=CARTESIAN_POINT('Ctrl Pts',(0.071360191489484,0.138321297100539,
-0.321713079532888));
#80833=CARTESIAN_POINT('Ctrl Pts',(0.0665070957496949,0.140719143160135,
-0.321300593597109));
#80834=CARTESIAN_POINT('Ctrl Pts',(0.0604511146818696,0.143327830066916,
-0.320812693485542));
#80835=CARTESIAN_POINT('Ctrl Pts',(0.0593584397561002,0.143783796003625,
-0.320725697203665));
#80836=CARTESIAN_POINT('Ctrl Pts',(0.0576112097965569,0.144489589795576,
-0.320588343478885));
#80837=CARTESIAN_POINT('Ctrl Pts',(0.0569600158959998,0.144747537782999,
-0.320537536129179));
#80838=CARTESIAN_POINT('Ctrl Pts',(0.055704460043638,0.145235097513607,
-0.320440342721329));
#80839=CARTESIAN_POINT('Ctrl Pts',(0.0551003781941231,0.145465352440342,
-0.320393922408553));
#80840=CARTESIAN_POINT('Ctrl Pts',(0.0537421817022358,0.145973374991262,
-0.32029028344851));
#80841=CARTESIAN_POINT('Ctrl Pts',(0.0529873029674625,0.1462490823832,-0.320233182970691));
#80842=CARTESIAN_POINT('Ctrl Pts',(0.0503171665215763,0.147200918594917,
-0.320032857854654));
#80843=CARTESIAN_POINT('Ctrl Pts',(0.0483907426641921,0.147845408125118,
-0.319891306619007));
#80844=CARTESIAN_POINT('Ctrl Pts',(0.037146669369087,0.151363792084599,
-0.319079222922563));
#80845=CARTESIAN_POINT('Ctrl Pts',(0.0275869269328072,0.153394520744539,
-0.318443514261546));
#80846=CARTESIAN_POINT('Ctrl Pts',(0.00996605592697227,0.155435699051433,
-0.317273987897849));
#80847=CARTESIAN_POINT('Ctrl Pts',(0.00197493010693328,0.15574228330505,
-0.316744404252176));
#80848=CARTESIAN_POINT('Ctrl Pts',(-0.00868910705218733,0.155330367386536,
-0.316012520815531));
#80849=CARTESIAN_POINT('Ctrl Pts',(-0.0113710324962245,0.155157087395567,
-0.31582640497958));
#80850=CARTESIAN_POINT('Ctrl Pts',(-0.0154122327222227,0.154790648241365,
-0.31554212674005));
#80851=CARTESIAN_POINT('Ctrl Pts',(-0.0167757348444684,0.154648815735772,
-0.315445551206598));
#80852=CARTESIAN_POINT('Ctrl Pts',(-0.0191455544922464,0.154370596764007,
-0.315276462152372));
#80853=CARTESIAN_POINT('Ctrl Pts',(-0.0201527566995663,0.154242340849208,
-0.315204206953287));
#80854=CARTESIAN_POINT('Ctrl Pts',(-0.0224269743602169,0.153930089316516,
-0.315040136548382));
#80855=CARTESIAN_POINT('Ctrl Pts',(-0.0236931044695245,0.153740294639807,
-0.314948144186946));
#80856=CARTESIAN_POINT('Ctrl Pts',(-0.0271037225009013,0.153185907214702,
-0.314698513826376));
#80857=CARTESIAN_POINT('Ctrl Pts',(-0.0292430693355967,0.152791936817779,
-0.314539968537613));
#80858=CARTESIAN_POINT('Ctrl Pts',(-0.0434940865710232,0.149857295025282,
-0.313470124199063));
#80859=CARTESIAN_POINT('Ctrl Pts',(-0.0552715078738923,0.145924252600084,
-0.312514075675306));
#80860=CARTESIAN_POINT('Ctrl Pts',(-0.0726673527218893,0.13770422422792,
-0.311023801793443));
#80861=CARTESIAN_POINT('Ctrl Pts',(-0.0786780474767305,0.1343606366774,
-0.310493805978386));
#80862=CARTESIAN_POINT('Ctrl Pts',(-0.0858115077254709,0.129749073358664,
-0.309860125724757));
#80863=CARTESIAN_POINT('Ctrl Pts',(-0.0871607618905411,0.128846571659886,
-0.309740067524514));
#80864=CARTESIAN_POINT('Ctrl Pts',(-0.089145772785032,0.127473363930259,
-0.309563414446321));
#80865=CARTESIAN_POINT('Ctrl Pts',(-0.0897924172014102,0.127018696271568,
-0.309505863481106));
#80866=CARTESIAN_POINT('Ctrl Pts',(-0.090900706063731,0.126226744147712,
-0.309407258180593));
#80867=CARTESIAN_POINT('Ctrl Pts',(-0.0913639874433515,0.12589182313022,
-0.30936605175881));
#80868=CARTESIAN_POINT('Ctrl Pts',(-0.092449840084606,0.125097673794527,
-0.309269497766083));
#80869=CARTESIAN_POINT('Ctrl Pts',(-0.0930708453419837,0.124636345964435,
-0.309214294074079));
#80870=CARTESIAN_POINT('Ctrl Pts',(-0.0949145776288989,0.123245222629986,
-0.309050358604073));
#80871=CARTESIAN_POINT('Ctrl Pts',(-0.0961270438172292,0.122301896376435,
-0.308942500840184));
#80872=CARTESIAN_POINT('Ctrl Pts',(-0.104559697708476,0.115538203302102,
-0.308190389339393));
#80873=CARTESIAN_POINT('Ctrl Pts',(-0.111261626617918,0.109099517511102,
-0.307581627383203));
#80874=CARTESIAN_POINT('Ctrl Pts',(-0.124178709282525,0.0942531972055352,
-0.306285432700813));
#80875=CARTESIAN_POINT('Ctrl Pts',(-0.130201534157377,0.0857411244615418,
-0.305599675402478));
#80876=CARTESIAN_POINT('Ctrl Pts',(-0.136335538792383,0.0749171971863099,
-0.304739042475821));
#80877=CARTESIAN_POINT('Ctrl Pts',(-0.137306451000273,0.073122523324995,
-0.304596777117482));
#80878=CARTESIAN_POINT('Ctrl Pts',(-0.138810265976411,0.0702071969106137,
-0.30436605391616));
#80879=CARTESIAN_POINT('Ctrl Pts',(-0.139365570234347,0.0690983220680937,
-0.304278382663857));
#80880=CARTESIAN_POINT('Ctrl Pts',(-0.140404384719368,0.0669604629035755,
-0.304109455066016));
#80881=CARTESIAN_POINT('Ctrl Pts',(-0.140889990564759,0.0659325812769539,
-0.304028277768552));
#80882=CARTESIAN_POINT('Ctrl Pts',(-0.141979783254097,0.0635587915278226,
-0.303840854867683));
#80883=CARTESIAN_POINT('Ctrl Pts',(-0.142576167346247,0.0622094451136279,
-0.303734351537556));
#80884=CARTESIAN_POINT('Ctrl Pts',(-0.144470081348812,0.0577540359266274,
-0.303382682284045));
#80885=CARTESIAN_POINT('Ctrl Pts',(-0.145685909611661,0.0546145183717806,
-0.30313484369636));
#80886=CARTESIAN_POINT('Ctrl Pts',(-0.150542807238968,0.0407534885815632,
-0.302039767954119));
#80887=CARTESIAN_POINT('Ctrl Pts',(-0.153108529579124,0.0296932287765719,
-0.301160347188309));
#80888=CARTESIAN_POINT('Ctrl Pts',(-0.15518460883441,0.0123180975927828,
-0.299806634002793));
#80889=CARTESIAN_POINT('Ctrl Pts',(-0.155551542164629,0.00614258291340502,
-0.299331611971668));
#80890=CARTESIAN_POINT('Ctrl Pts',(-0.155549607151914,-0.00158917287991982,
-0.298755512407639));
#80891=CARTESIAN_POINT('Ctrl Pts',(-0.155526044074766,-0.00313940290399828,
-0.298640952897414));
#80892=CARTESIAN_POINT('Ctrl Pts',(-0.155455903163095,-0.00546510875804829,
-0.298470757023469));
#80893=CARTESIAN_POINT('Ctrl Pts',(-0.155426689375158,-0.00624095670408139,
-0.298414259485607));
#80894=CARTESIAN_POINT('Ctrl Pts',(-0.155365886810345,-0.00758751276029682,
-0.298316724405288));
#80895=CARTESIAN_POINT('Ctrl Pts',(-0.155336960708364,-0.00815829635502679,
-0.298275546326686));
#80896=CARTESIAN_POINT('Ctrl Pts',(-0.155260699360192,-0.00951513483507425,
-0.298178048271776));
#80897=CARTESIAN_POINT('Ctrl Pts',(-0.155210540536866,-0.0103010064552261,
-0.298121883632185));
#80898=CARTESIAN_POINT('Ctrl Pts',(-0.155039855924804,-0.0126897229362202,
-0.297952003431668));
#80899=CARTESIAN_POINT('Ctrl Pts',(-0.154900448596701,-0.014291170111211,
-0.29783925844996));
#80900=CARTESIAN_POINT('Ctrl Pts',(-0.154050247483862,-0.0225702676408501,
-0.297260989561896));
#80901=CARTESIAN_POINT('Ctrl Pts',(-0.152932323938379,-0.029199679994003,
-0.296813291170937));
#80902=CARTESIAN_POINT('Ctrl Pts',(-0.148491034362419,-0.0480140174521139,
-0.295535466929416));
#80903=CARTESIAN_POINT('Ctrl Pts',(-0.14411061745827,-0.0598918201436837,
-0.294715751762492));
#80904=CARTESIAN_POINT('Ctrl Pts',(-0.137353600519461,-0.0730375795244298,
-0.293695187238585));
#80905=CARTESIAN_POINT('Ctrl Pts',(-0.136322691964313,-0.0749441289201565,
-0.293544292359504));
#80906=CARTESIAN_POINT('Ctrl Pts',(-0.134626723801917,-0.077929789500584,
-0.29330300189276));
#80907=CARTESIAN_POINT('Ctrl Pts',(-0.133987704337724,-0.0790234254538095,
-0.293213530962021));
#80908=CARTESIAN_POINT('Ctrl Pts',(-0.132753243559565,-0.081078089996767,
-0.29304329492563));
#80909=CARTESIAN_POINT('Ctrl Pts',(-0.132160539180629,-0.0820406735305506,
-0.292962633102756));
#80910=CARTESIAN_POINT('Ctrl Pts',(-0.130784268687581,-0.084222189254922,
-0.292777691705462));
#80911=CARTESIAN_POINT('Ctrl Pts',(-0.129994066217153,-0.0854367870712042,
-0.292673172805494));
#80912=CARTESIAN_POINT('Ctrl Pts',(-0.12745166189055,-0.0892277055727707,
-0.292341921080406));
#80913=CARTESIAN_POINT('Ctrl Pts',(-0.125639061034569,-0.091762374399115,
-0.292112964695512));
#80914=CARTESIAN_POINT('Ctrl Pts',(-0.121116916493584,-0.097700602095763,
-0.291557922715467));
#80915=CARTESIAN_POINT('Ctrl Pts',(-0.118338422613799,-0.101048141916091,
-0.291229481986223));
#80916=CARTESIAN_POINT('Ctrl Pts',(-0.111247974901332,-0.108896691394552,
-0.290421482821475));
#80917=CARTESIAN_POINT('Ctrl Pts',(-0.106798718969604,-0.113263530635705,
-0.28993854592397));
#80918=CARTESIAN_POINT('Ctrl Pts',(-0.0966667491466219,-0.122078690107172,
-0.288898026968516));
#80919=CARTESIAN_POINT('Ctrl Pts',(-0.0909112997371471,-0.126423188949271,
-0.288341710379856));
#80920=CARTESIAN_POINT('Ctrl Pts',(-0.0835330513956159,-0.131227268664951,
-0.287685127246972));
#80921=CARTESIAN_POINT('Ctrl Pts',(-0.0821776383292283,-0.132080289980819,
-0.287566712739405));
#80922=CARTESIAN_POINT('Ctrl Pts',(-0.0801373742888518,-0.133320748503863,
-0.287391986417021));
#80923=CARTESIAN_POINT('Ctrl Pts',(-0.0794624155207532,-0.133724138921695,
-0.28733474733288));
#80924=CARTESIAN_POINT('Ctrl Pts',(-0.0782371391933199,-0.134443874520561,
-0.287231893103517));
#80925=CARTESIAN_POINT('Ctrl Pts',(-0.0776879175883482,-0.13476198589118,
-0.28718617134235));
#80926=CARTESIAN_POINT('Ctrl Pts',(-0.0764326942394409,-0.135478791919709,
-0.287082534534691));
#80927=CARTESIAN_POINT('Ctrl Pts',(-0.0757255044505087,-0.135875339416135,
-0.287024753405496));
#80928=CARTESIAN_POINT('Ctrl Pts',(-0.073498390652203,-0.137101375362434,
-0.286844578444149));
#80929=CARTESIAN_POINT('Ctrl Pts',(-0.0719676365458002,-0.137911060075139,
-0.286723334284815));
#80930=CARTESIAN_POINT('Ctrl Pts',(-0.0682606318143345,-0.139793323386092,
-0.286435113261444));
#80931=CARTESIAN_POINT('Ctrl Pts',(-0.0660721427909364,-0.140840904593983,
-0.286269326981563));
#80932=CARTESIAN_POINT('Ctrl Pts',(-0.0570478087702293,-0.14490397422584,
-0.285599738520941));
#80933=CARTESIAN_POINT('Ctrl Pts',(-0.0500231310482297,-0.147476491644343,
-0.285110432888552));
#80934=CARTESIAN_POINT('Ctrl Pts',(-0.0343819299477129,-0.151957568813729,
-0.284038200592309));
#80935=CARTESIAN_POINT('Ctrl Pts',(-0.0257341202640613,-0.153658548126121,
-0.283455536359174));
#80936=CARTESIAN_POINT('Ctrl Pts',(-0.0148274964742767,-0.154856961367827,
-0.282700477575218));
#80937=CARTESIAN_POINT('Ctrl Pts',(-0.01266085682664,-0.155049137545369,
-0.282549573702179));
#80938=CARTESIAN_POINT('Ctrl Pts',(-0.00910386767394617,-0.155289584281115,
-0.28229993562745));
#80939=CARTESIAN_POINT('Ctrl Pts',(-0.00771559456445765,-0.155364747520493,
-0.28220203202903));
#80940=CARTESIAN_POINT('Ctrl Pts',(-0.00520200674194078,-0.155467064983784,
-0.282023822291512));
#80941=CARTESIAN_POINT('Ctrl Pts',(-0.00407703817784952,-0.155500632820194,
-0.281943721097383));
#80942=CARTESIAN_POINT('Ctrl Pts',(-0.0016462645624265,-0.155546769269533,
-0.281769853652271));
#80943=CARTESIAN_POINT('Ctrl Pts',(-0.000340476043106266,-0.155555107603514,
-0.28167596197086));
#80944=CARTESIAN_POINT('Ctrl Pts',(0.00332283652720539,-0.155532375392482,
-0.281411096590015));
#80945=CARTESIAN_POINT('Ctrl Pts',(0.00567968293065076,-0.155464147375873,
-0.28123899225281));
#80946=CARTESIAN_POINT('Ctrl Pts',(0.0160363573838207,-0.154928523796453,
-0.280474814526348));
#80947=CARTESIAN_POINT('Ctrl Pts',(0.0239935958899593,-0.153896991398887,
-0.279866021609797));
#80948=CARTESIAN_POINT('Ctrl Pts',(0.0405129523280155,-0.15044302565002,
-0.278564267130008));
#80949=CARTESIAN_POINT('Ctrl Pts',(0.049020061628579,-0.147889969579086,
-0.277871468719104));
#80950=CARTESIAN_POINT('Ctrl Pts',(0.0601541550801836,-0.143481518347877,
-0.276961609693985));
#80951=CARTESIAN_POINT('Ctrl Pts',(0.0630101143312593,-0.14225047333252,
-0.276728063734208));
#80952=CARTESIAN_POINT('Ctrl Pts',(0.066768016638625,-0.140495238597484,
-0.276422216591579));
#80953=CARTESIAN_POINT('Ctrl Pts',(0.0677041737846811,-0.140046510567872,
-0.276346149323808));
#80954=CARTESIAN_POINT('Ctrl Pts',(0.0691766534402561,-0.139322490511125,
-0.276226779705948));
#80955=CARTESIAN_POINT('Ctrl Pts',(0.069715967472237,-0.139053405769155,
-0.27618311835309));
#80956=CARTESIAN_POINT('Ctrl Pts',(0.07084480534099,-0.138481966247615,
-0.27609187642972));
#80957=CARTESIAN_POINT('Ctrl Pts',(0.0714339857500194,-0.138178967748704,
-0.276044340049154));
#80958=CARTESIAN_POINT('Ctrl Pts',(0.0729138774641495,-0.137405906871741,
-0.275925111684539));
#80959=CARTESIAN_POINT('Ctrl Pts',(0.073802013731886,-0.136930930328859,
-0.275853716865926));
#80960=CARTESIAN_POINT('Ctrl Pts',(0.0774012105278814,-0.134960882246662,
-0.275564774646624));
#80961=CARTESIAN_POINT('Ctrl Pts',(0.0800721628053102,-0.133393549532656,
-0.275351250883022));
#80962=CARTESIAN_POINT('Ctrl Pts',(0.0875618131086776,-0.128692471420388,
-0.274749853935152));
#80963=CARTESIAN_POINT('Ctrl Pts',(0.0922562062560516,-0.125369953687317,
-0.274369547563549));
#80964=CARTESIAN_POINT('Ctrl Pts',(0.105574175569846,-0.114789910879557,
-0.273247978516741));
#80965=CARTESIAN_POINT('Ctrl Pts',(0.113604320642675,-0.10684874957738,
-0.272511461397408));
#80966=CARTESIAN_POINT('Ctrl Pts',(0.122158618889659,-0.0963243175115933,
-0.271577118846981));
#80967=CARTESIAN_POINT('Ctrl Pts',(0.123570746881867,-0.0945059357202949,
-0.271417131269575));
#80968=CARTESIAN_POINT('Ctrl Pts',(0.125720932240138,-0.0916065494053033,
-0.27116380311641));
#80969=CARTESIAN_POINT('Ctrl Pts',(0.126486621492542,-0.0905463809065521,
-0.27107153264621));
#80970=CARTESIAN_POINT('Ctrl Pts',(0.127886149705519,-0.0885562056881211,
-0.270898904482829));
#80971=CARTESIAN_POINT('Ctrl Pts',(0.12852344300986,-0.0876287243311157,
-0.270818685211601));
#80972=CARTESIAN_POINT('Ctrl Pts',(0.129924074026566,-0.0855421734960147,
-0.270638678097841));
#80973=CARTESIAN_POINT('Ctrl Pts',(0.130682067086161,-0.0843796513964934,
-0.270538699051406));
#80974=CARTESIAN_POINT('Ctrl Pts',(0.132909728695237,-0.0808610961356502,
-0.270236928755979));
#80975=CARTESIAN_POINT('Ctrl Pts',(0.134331895257323,-0.0784758112442404,
-0.270033443760925));
#80976=CARTESIAN_POINT('Ctrl Pts',(0.138601560385234,-0.0708582085333875,
-0.269386563920474));
#80977=CARTESIAN_POINT('Ctrl Pts',(0.141212578133769,-0.065500161864576,
-0.268935605584176));
#80978=CARTESIAN_POINT('Ctrl Pts',(0.14428338561334,-0.0581560703844953,
-0.268324542680345));
#80979=CARTESIAN_POINT('Ctrl Pts',(0.145021115880139,-0.0562912028906115,
-0.268169990125387));
#80980=CARTESIAN_POINT('Ctrl Pts',(0.149213374758756,-0.0450639062517173,
-0.26724399780844));
#80981=CARTESIAN_POINT('Ctrl Pts',(0.15179661786613,-0.035400515145278,
-0.266463598253098));
#80982=CARTESIAN_POINT('Ctrl Pts',(0.153738558825832,-0.0237411520744586,
-0.265578875701345));
#80983=CARTESIAN_POINT('Ctrl Pts',(0.154008600880754,-0.0219211861052032,
-0.265442434793654));
#80984=CARTESIAN_POINT('Ctrl Pts',(0.154352431084631,-0.0192822260481019,
-0.265247379978161));
#80985=CARTESIAN_POINT('Ctrl Pts',(0.15445210589775,-0.0184668429123928,
-0.265187495217724));
#80986=CARTESIAN_POINT('Ctrl Pts',(0.154617484667173,-0.0170188245750852,
-0.265081870649495));
#80987=CARTESIAN_POINT('Ctrl Pts',(0.15468577438873,-0.0163865252033171,
-0.265035994837533));
#80988=CARTESIAN_POINT('Ctrl Pts',(0.154827760440746,-0.014991789578896,
-0.264935349332066));
#80989=CARTESIAN_POINT('Ctrl Pts',(0.154899705816366,-0.0142292080456393,
-0.264880675224894));
#80990=CARTESIAN_POINT('Ctrl Pts',(0.155095657690461,-0.0119742217889823,
-0.264719965119066));
#80991=CARTESIAN_POINT('Ctrl Pts',(0.155203753663212,-0.0104804723997598,
-0.264614752809675));
#80992=CARTESIAN_POINT('Ctrl Pts',(0.155620548156694,-0.0032771565080258,
-0.264112366097192));
#80993=CARTESIAN_POINT('Ctrl Pts',(0.155635884889912,0.00244554408657134,
-0.263728214927522));
#80994=CARTESIAN_POINT('Ctrl Pts',(0.15462532416037,0.0216907172833835,
-0.262448752975366));
#80995=CARTESIAN_POINT('Ctrl Pts',(0.152149161910106,0.0350726613191967,
-0.261574306215701));
#80996=CARTESIAN_POINT('Ctrl Pts',(0.147269646702286,0.050126018370757,
-0.260483685098901));
#80997=CARTESIAN_POINT('Ctrl Pts',(0.146521673775424,0.0522720265913844,
-0.260325709870193));
#80998=CARTESIAN_POINT('Ctrl Pts',(0.14527186664726,0.0556199675975706,
-0.260074864363362));
#80999=CARTESIAN_POINT('Ctrl Pts',(0.144801470889826,0.0568333518285932,
-0.259983029142518));
#81000=CARTESIAN_POINT('Ctrl Pts',(0.143895840188974,0.0590851685460495,
-0.259810794872113));
#81001=CARTESIAN_POINT('Ctrl Pts',(0.14346444475922,0.0601250607830885,
-0.259730528922739));
#81002=CARTESIAN_POINT('Ctrl Pts',(0.142472874223701,0.0624438288473355,
-0.25954986365613));
#81003=CARTESIAN_POINT('Ctrl Pts',(0.141906698627159,0.0637200149156635,
-0.259449266577453));
#81004=CARTESIAN_POINT('Ctrl Pts',(0.140144667671015,0.0675517201084837,
-0.259143593520673));
#81005=CARTESIAN_POINT('Ctrl Pts',(0.138896449057761,0.0700823608466168,
-0.258936757824729));
#81006=CARTESIAN_POINT('Ctrl Pts',(0.134228034344481,0.078931951923188,
-0.258195197389933));
#81007=CARTESIAN_POINT('Ctrl Pts',(0.130440122460054,0.0850456811818212,
-0.257648494844447));
#81008=CARTESIAN_POINT('Ctrl Pts',(0.121127845779657,0.0979823111246914,
-0.256419249406507));
#81009=CARTESIAN_POINT('Ctrl Pts',(0.115420774050056,0.104644819969919,
-0.255735028883777));
#81010=CARTESIAN_POINT('Ctrl Pts',(0.106967115260322,0.11297574982386,-0.254832118582925));
#81011=CARTESIAN_POINT('Ctrl Pts',(0.104685744149188,0.115092925611983,
-0.254598006970998));
#81012=CARTESIAN_POINT('Ctrl Pts',(0.102342242833752,0.117140376607545,
-0.254368055082067));
#81013=CARTESIAN_POINT('Origin',(0.,0.,-1.10400562256037));
#81014=CARTESIAN_POINT('',(0.10234224283772,0.117140376604078,-0.170697633677947));
#81015=CARTESIAN_POINT('',(0.102342242826532,0.117140376613853,-0.184536881298507));
#81016=CARTESIAN_POINT('',(0.10234224283772,0.117140376604078,-1.10400562256037));
#81017=CARTESIAN_POINT('',(-0.155549984535534,-6.93613367895633E-5,-0.215194377432725));
#81018=CARTESIAN_POINT('Ctrl Pts',(-0.155549984535534,-6.93613367884616E-5,
-0.215194377432725));
#81019=CARTESIAN_POINT('Ctrl Pts',(-0.155544924241764,-0.0114175944321142,
-0.214385432002025));
#81020=CARTESIAN_POINT('Ctrl Pts',(-0.154293756121922,-0.0227244664062756,
-0.213576486571325));
#81021=CARTESIAN_POINT('Ctrl Pts',(-0.151848298219052,-0.0337327263644348,
-0.212767541140625));
#81022=CARTESIAN_POINT('Ctrl Pts',(-0.149670179599569,-0.0435375551267021,
-0.212047030228257));
#81023=CARTESIAN_POINT('Ctrl Pts',(-0.146545503580168,-0.053105400351191,
-0.211326519315889));
#81024=CARTESIAN_POINT('Ctrl Pts',(-0.14254312808969,-0.0622676411501693,
-0.210606008403521));
#81025=CARTESIAN_POINT('Ctrl Pts',(-0.138446014228048,-0.071646757095313,
-0.209868442612018));
#81026=CARTESIAN_POINT('Ctrl Pts',(-0.133404010521729,-0.0806546181908517,
-0.209130876820515));
#81027=CARTESIAN_POINT('Ctrl Pts',(-0.127507151897742,-0.0890939319758985,
-0.208393311029012));
#81028=CARTESIAN_POINT('Ctrl Pts',(-0.121596275402187,-0.0975533074962367,
-0.207653991913714));
#81029=CARTESIAN_POINT('Ctrl Pts',(-0.114826884814375,-0.105440584507109,
-0.206914672798417));
#81030=CARTESIAN_POINT('Ctrl Pts',(-0.107335662132136,-0.112582672444101,
-0.206175353683119));
#81031=CARTESIAN_POINT('Ctrl Pts',(-0.0998792645099848,-0.119691558372276,
-0.205439471501111));
#81032=CARTESIAN_POINT('Ctrl Pts',(-0.0917084040091688,-0.126061522420267,
-0.204703589319102));
#81033=CARTESIAN_POINT('Ctrl Pts',(-0.0829951478406017,-0.131558382229779,
-0.203967707137094));
#81034=CARTESIAN_POINT('Ctrl Pts',(-0.0742208488565232,-0.137093751615132,
-0.203226669555152));
#81035=CARTESIAN_POINT('Ctrl Pts',(-0.0648973211481259,-0.141743217842826,
-0.20248563197321));
#81036=CARTESIAN_POINT('Ctrl Pts',(-0.0552271822349882,-0.145415820468006,
-0.201744594391268));
#81037=CARTESIAN_POINT('Ctrl Pts',(-0.04555704332185,-0.149088423093186,
-0.201003556809326));
#81038=CARTESIAN_POINT('Ctrl Pts',(-0.0355412212476219,-0.151783947600411,
-0.200262519227384));
#81039=CARTESIAN_POINT('Ctrl Pts',(-0.0253960749986721,-0.153462835483585,
-0.199521481645442));
#81040=CARTESIAN_POINT('Ctrl Pts',(-0.0152984561802915,-0.155133858203917,
-0.198783915636147));
#81041=CARTESIAN_POINT('Ctrl Pts',(-0.00499768058454571,-0.155810207328269,
-0.198046349626853));
#81042=CARTESIAN_POINT('Ctrl Pts',(0.00529174832921784,-0.155459962368515,
-0.197308783617558));
#81043=CARTESIAN_POINT('Ctrl Pts',(0.0156056332226933,-0.155108884944327,
-0.196569464556709));
#81044=CARTESIAN_POINT('Ctrl Pts',(0.0259071855506799,-0.15372621134018,
-0.195830145495859));
#81045=CARTESIAN_POINT('Ctrl Pts',(0.0359767993225822,-0.151332324407255,
-0.195090826435009));
#81046=CARTESIAN_POINT('Ctrl Pts',(0.0459996053868997,-0.148949565245671,
-0.19435494403332));
#81047=CARTESIAN_POINT('Ctrl Pts',(0.0557917163008593,-0.145565185573833,
-0.193619061631631));
#81048=CARTESIAN_POINT('Ctrl Pts',(0.0651468902848729,-0.141250434286804,
-0.192883179229942));
#81049=CARTESIAN_POINT('Ctrl Pts',(0.0745675989473153,-0.136905457390013,
-0.192142141839512));
#81050=CARTESIAN_POINT('Ctrl Pts',(0.0835443572856849,-0.131617409202288,
-0.191401104449082));
#81051=CARTESIAN_POINT('Ctrl Pts',(0.0918905391417884,-0.125506698292288,
-0.190660067058652));
#81052=CARTESIAN_POINT('Ctrl Pts',(0.100236720997892,-0.119395987382288,
-0.189919029668222));
#81053=CARTESIAN_POINT('Ctrl Pts',(0.107951641088085,-0.112463275310278,
-0.189177992277792));
#81054=CARTESIAN_POINT('Ctrl Pts',(0.114884302548217,-0.104868486820444,
-0.188436954887361));
#81055=CARTESIAN_POINT('Ctrl Pts',(0.121784482046381,-0.097309282591043,
-0.187699389518243));
#81056=CARTESIAN_POINT('Ctrl Pts',(0.127961030407077,-0.0890380370869365,
-0.186961824149124));
#81057=CARTESIAN_POINT('Ctrl Pts',(0.133270367378195,-0.0802172779323822,
-0.186224258780005));
#81058=CARTESIAN_POINT('Ctrl Pts',(0.138592329386306,-0.0713755439534292,
-0.185484939559112));
#81059=CARTESIAN_POINT('Ctrl Pts',(0.143042345846606,-0.0619823981288728,
-0.184745620338218));
#81060=CARTESIAN_POINT('Ctrl Pts',(0.14651792591867,-0.0522331301425736,
-0.184006301117324));
#81061=CARTESIAN_POINT('Ctrl Pts',(0.14997734635418,-0.0425291911730338,
-0.183270419345621));
#81062=CARTESIAN_POINT('Ctrl Pts',(0.152471055355108,-0.0324733116894837,
-0.182534537573919));
#81063=CARTESIAN_POINT('Ctrl Pts',(0.153946502728169,-0.0222772708778693,
-0.181798655802216));
#81064=CARTESIAN_POINT('Ctrl Pts',(0.155432288260647,-0.0120097884836756,
-0.181057617856727));
#81065=CARTESIAN_POINT('Ctrl Pts',(0.155885338135254,-0.00160111105110903,
-0.180316579911238));
#81066=CARTESIAN_POINT('Ctrl Pts',(0.155305015513463,0.00872666352984315,
-0.179575541965749));
#81067=CARTESIAN_POINT('Ctrl Pts',(0.154724692891672,0.0190544381107961,
-0.178834504020259));
#81068=CARTESIAN_POINT('Ctrl Pts',(0.153111179475993,0.0293003748119713,
-0.17809346607477));
#81069=CARTESIAN_POINT('Ctrl Pts',(0.150516384009077,0.039250740691509,
-0.177352428129281));
#81070=CARTESIAN_POINT('Ctrl Pts',(0.147933773686665,0.0491543797104302,
-0.176614870093697));
#81071=CARTESIAN_POINT('Ctrl Pts',(0.144359921071405,0.0588388340894559,
-0.175877312058113));
#81072=CARTESIAN_POINT('Ctrl Pts',(0.139852954270346,0.0680951810472411,
-0.17513975402253));
#81073=CARTESIAN_POINT('Ctrl Pts',(0.135328906002627,0.0773866096883254,
-0.174399400631766));
#81074=CARTESIAN_POINT('Ctrl Pts',(0.129864919948991,0.0862457725237679,
-0.173659047241002));
#81075=CARTESIAN_POINT('Ctrl Pts',(0.12356946561236,0.0944795727566328,
-0.172918693850239));
#81076=CARTESIAN_POINT('Ctrl Pts',(0.117274011275729,0.102713372989497,
-0.172178340459475));
#81077=CARTESIAN_POINT('Ctrl Pts',(0.110147633291769,0.110321027132533,
-0.171437987068711));
#81078=CARTESIAN_POINT('Ctrl Pts',(0.10234224283772,0.117140376604078,-0.170697633677947));
#81079=CARTESIAN_POINT('Ctrl Pts',(0.102342242837721,0.117140376604077,
-0.240688435831897));
#81080=CARTESIAN_POINT('Ctrl Pts',(0.0945907992358971,0.123912594232521,
-0.239952236984707));
#81081=CARTESIAN_POINT('Ctrl Pts',(0.0861522819330473,0.129922626667033,
-0.239216038137517));
#81082=CARTESIAN_POINT('Ctrl Pts',(0.077201467392696,0.135039756858543,
-0.238479839290327));
#81083=CARTESIAN_POINT('Ctrl Pts',(0.0682553086659258,0.140154225347687,
-0.237744023380866));
#81084=CARTESIAN_POINT('Ctrl Pts',(0.0587981892741572,0.144376258801276,
-0.237008207471405));
#81085=CARTESIAN_POINT('Ctrl Pts',(0.0490306936084764,0.147620437556159,
-0.236272391561943));
#81086=CARTESIAN_POINT('Ctrl Pts',(0.039239939646621,0.150872341328067,
-0.235534823532498));
#81087=CARTESIAN_POINT('Ctrl Pts',(0.0291382295232789,0.153141489378281,
-0.234797255503053));
#81088=CARTESIAN_POINT('Ctrl Pts',(0.0189409422343509,0.154392497250595,
-0.234059687473607));
#81089=CARTESIAN_POINT('Ctrl Pts',(0.0130207218573329,0.15511879259637,
-0.233631478955632));
#81090=CARTESIAN_POINT('Ctrl Pts',(0.00706846490628639,0.155502887085559,
-0.233203270437657));
#81091=CARTESIAN_POINT('Ctrl Pts',(0.00112651773548907,0.155545920736584,
-0.232775061919681));
#81092=CARTESIAN_POINT('Ctrl Pts',(-0.00910816235334534,0.155620043854584,
-0.232037496090364));
#81093=CARTESIAN_POINT('Ctrl Pts',(-0.019388222831283,0.154679973770776,
-0.231299930261046));
#81094=CARTESIAN_POINT('Ctrl Pts',(-0.0294968071169101,0.15272766897294,
-0.230562364431728));
#81095=CARTESIAN_POINT('Ctrl Pts',(-0.0396294206387574,0.150770723328093,
-0.229823045325885));
#81096=CARTESIAN_POINT('Ctrl Pts',(-0.0495888031548398,0.147796755498571,
-0.229083726220041));
#81097=CARTESIAN_POINT('Ctrl Pts',(-0.0591612233517547,0.143860182648027,
-0.228344407114197));
#81098=CARTESIAN_POINT('Ctrl Pts',(-0.068689144095095,0.139941909802832,
-0.227608524892187));
#81099=CARTESIAN_POINT('Ctrl Pts',(-0.0778328285156711,0.135070313602817,
-0.226872642670177));
#81100=CARTESIAN_POINT('Ctrl Pts',(-0.0863996868963797,0.129347967143699,
-0.226136760448167));
#81101=CARTESIAN_POINT('Ctrl Pts',(-0.0950265616007538,0.123585531986723,
-0.225395722900406));
#81102=CARTESIAN_POINT('Ctrl Pts',(-0.103067699695561,0.116960896736977,
-0.224654685352646));
#81103=CARTESIAN_POINT('Ctrl Pts',(-0.110357561019662,0.10962212927047,
-0.223913647804885));
#81104=CARTESIAN_POINT('Ctrl Pts',(-0.117647422343763,0.102283361803962,
-0.223172610257124));
#81105=CARTESIAN_POINT('Ctrl Pts',(-0.124185433295616,0.0942312225561094,
-0.222431572709363));
#81106=CARTESIAN_POINT('Ctrl Pts',(-0.129847415376793,0.0856472487588859,
-0.221690535161602));
#81107=CARTESIAN_POINT('Ctrl Pts',(-0.135586640544162,0.0769461688637659,
-0.220939388075105));
#81108=CARTESIAN_POINT('Ctrl Pts',(-0.140467434326455,0.0676358586772041,
-0.220188240988607));
#81109=CARTESIAN_POINT('Ctrl Pts',(-0.144370123305893,0.0579056991723721,
-0.21943709390211));
#81110=CARTESIAN_POINT('Ctrl Pts',(-0.148263561630633,0.0481986033413841,
-0.218687727280918));
#81111=CARTESIAN_POINT('Ctrl Pts',(-0.151183090597988,0.0380744094506218,
-0.217938360659726));
#81112=CARTESIAN_POINT('Ctrl Pts',(-0.15305544994819,0.0277458418714797,
-0.217188994038534));
#81113=CARTESIAN_POINT('Ctrl Pts',(-0.154716692448818,0.0185818662536416,
-0.216524121838899));
#81114=CARTESIAN_POINT('Ctrl Pts',(-0.155554143584908,0.00925775084187499,
-0.215859249639264));
#81115=CARTESIAN_POINT('Ctrl Pts',(-0.155549984535578,-6.93612399397573E-5,
-0.215194377439629));
#81116=CARTESIAN_POINT('',(-0.155549939620994,0.000137054387354205,-0.229033329119584));
#81117=CARTESIAN_POINT('Ctrl Pts',(0.102342242833752,0.117140376607545,
-0.254368055082067));
#81118=CARTESIAN_POINT('Ctrl Pts',(0.102237155459024,0.117232188482618,
-0.254357743570756));
#81119=CARTESIAN_POINT('Ctrl Pts',(0.102131943151496,0.117323860156174,
-0.254347440447633));
#81120=CARTESIAN_POINT('Ctrl Pts',(0.101230699495509,0.118106984331783,
-0.254259361857058));
#81121=CARTESIAN_POINT('Ctrl Pts',(0.100427751951031,0.118790492334365,
-0.254182072473187));
#81122=CARTESIAN_POINT('Ctrl Pts',(0.0991525990076992,0.119853792747519,
-0.254061258475514));
#81123=CARTESIAN_POINT('Ctrl Pts',(0.098685037457719,0.120239065787949,
-0.254017360350847));
#81124=CARTESIAN_POINT('Ctrl Pts',(0.09770379834357,0.12103803228153,-0.253926088736467));
#81125=CARTESIAN_POINT('Ctrl Pts',(0.0971897210145893,0.121451206760199,
-0.253878755764946));
#81126=CARTESIAN_POINT('Ctrl Pts',(0.0958957476446415,0.122477722284622,
-0.253760779619929));
#81127=CARTESIAN_POINT('Ctrl Pts',(0.0951125639313814,0.12308690909447,
-0.253690420536054));
#81128=CARTESIAN_POINT('Ctrl Pts',(0.0919662299546577,0.125486269452311,
-0.253411660576555));
#81129=CARTESIAN_POINT('Ctrl Pts',(0.0895577780559352,0.127216345240533,
-0.253206934893019));
#81130=CARTESIAN_POINT('Ctrl Pts',(0.0826721827140387,0.131869967987762,
-0.252640863873219));
#81131=CARTESIAN_POINT('Ctrl Pts',(0.078091516219679,0.134633211558832,
-0.252286067737515));
#81132=CARTESIAN_POINT('Ctrl Pts',(0.0628318062082967,0.142797077335476,
-0.251143612545098));
#81133=CARTESIAN_POINT('Ctrl Pts',(0.0516720087248723,0.147203298417664,
-0.250364046703397));
#81134=CARTESIAN_POINT('Ctrl Pts',(0.0379652838529928,0.150862204128483,
-0.249385698727708));
#81135=CARTESIAN_POINT('Ctrl Pts',(0.0358004580935539,0.151390533900714,
-0.2492307252812));
#81136=CARTESIAN_POINT('Ctrl Pts',(0.0323638731944192,0.152151407938639,
-0.248983584670104));
#81137=CARTESIAN_POINT('Ctrl Pts',(0.0310992300763334,0.15241492359857,
-0.24889240123796));
#81138=CARTESIAN_POINT('Ctrl Pts',(0.028736195244139,0.152876679222919,
-0.248721505364394));
#81139=CARTESIAN_POINT('Ctrl Pts',(0.0276386608629597,0.153078908653628,
-0.248641925078218));
#81140=CARTESIAN_POINT('Ctrl Pts',(0.0251557270309056,0.153508836596325,
-0.248461379400763));
#81141=CARTESIAN_POINT('Ctrl Pts',(0.023769246937255,0.153729620363511,
-0.248360203079257));
#81142=CARTESIAN_POINT('Ctrl Pts',(0.0195461659202881,0.154343611202967,
-0.248050842254632));
#81143=CARTESIAN_POINT('Ctrl Pts',(0.0167016696748106,0.154677261298513,
-0.247840834539995));
#81144=CARTESIAN_POINT('Ctrl Pts',(0.00606029667304388,0.155628518483842,
-0.247048609468335));
#81145=CARTESIAN_POINT('Ctrl Pts',(-0.00176950607963955,0.155736317986571,
-0.246451824251603));
#81146=CARTESIAN_POINT('Ctrl Pts',(-0.0195188630475428,0.154641871805015,
-0.245077820488252));
#81147=CARTESIAN_POINT('Ctrl Pts',(-0.0293830388359485,0.153074341744745,
-0.244298571100877));
#81148=CARTESIAN_POINT('Ctrl Pts',(-0.0408252246802439,0.150108438451841,
-0.243413628989057));
#81149=CARTESIAN_POINT('Ctrl Pts',(-0.0426121913330136,0.149610976221383,
-0.243276049838723));
#81150=CARTESIAN_POINT('Ctrl Pts',(-0.0451796869573198,0.148846489365071,
-0.243079684867336));
#81151=CARTESIAN_POINT('Ctrl Pts',(-0.0459675843097169,0.148605056386415,
-0.24301960537448));
#81152=CARTESIAN_POINT('Ctrl Pts',(-0.0473603025091855,0.148166153214888,
-0.242913770474043));
#81153=CARTESIAN_POINT('Ctrl Pts',(-0.0479658806957881,0.14797121866722,
-0.242867876934328));
#81154=CARTESIAN_POINT('Ctrl Pts',(-0.0492960128460711,0.147534027269328,
-0.242767354683724));
#81155=CARTESIAN_POINT('Ctrl Pts',(-0.0500199972454502,0.147290142323381,
-0.242712819787466));
#81156=CARTESIAN_POINT('Ctrl Pts',(-0.0521482624463817,0.146555701857846,
-0.242552951865193));
#81157=CARTESIAN_POINT('Ctrl Pts',(-0.0535473843819025,0.146050310071637,
-0.242448429625248));
#81158=CARTESIAN_POINT('Ctrl Pts',(-0.0646625466860618,0.141854072276852,
-0.241621031911769));
#81159=CARTESIAN_POINT('Ctrl Pts',(-0.0739950524959171,0.137217410717385,
-0.240943368765056));
#81160=CARTESIAN_POINT('Ctrl Pts',(-0.0908053356306465,0.126647928935881,
-0.239634617721139));
#81161=CARTESIAN_POINT('Ctrl Pts',(-0.0983372909981724,0.120892724275524,
-0.239007317317134));
#81162=CARTESIAN_POINT('Ctrl Pts',(-0.106763368528717,0.113143016164262,
-0.238214769340962));
#81163=CARTESIAN_POINT('Ctrl Pts',(-0.108201373991743,0.111768604766045,
-0.238075993724116));
#81164=CARTESIAN_POINT('Ctrl Pts',(-0.110484879049356,0.109500709862623,
-0.23784954042197));
#81165=CARTESIAN_POINT('Ctrl Pts',(-0.111346857856541,0.108624081350539,
-0.237762596087138));
#81166=CARTESIAN_POINT('Ctrl Pts',(-0.112988180000601,0.106914798452867,
-0.237594124907835));
#81167=CARTESIAN_POINT('Ctrl Pts',(-0.113768937480959,0.106083607054832,
-0.237512666749974));
#81168=CARTESIAN_POINT('Ctrl Pts',(-0.114602093295998,0.105176855859264,
-0.237424277959772));
#81169=CARTESIAN_POINT('Ctrl Pts',(-0.114663660870459,0.105109731576027,
-0.237417737558879));
#81170=CARTESIAN_POINT('Ctrl Pts',(-0.114781783749357,0.104980720362508,
-0.237405172379322));
#81171=CARTESIAN_POINT('Ctrl Pts',(-0.114838348066653,0.104918841691026,
-0.237399147982927));
#81172=CARTESIAN_POINT('Ctrl Pts',(-0.114947899103571,0.104798803341607,
-0.237387465783282));
#81173=CARTESIAN_POINT('Ctrl Pts',(-0.115000891789213,0.104740649118675,
-0.237381808233095));
#81174=CARTESIAN_POINT('Ctrl Pts',(-0.115104396697849,0.104626889489676,
-0.237370745090582));
#81175=CARTESIAN_POINT('Ctrl Pts',(-0.115154912813204,0.10457128763866,
-0.237365339663611));
#81176=CARTESIAN_POINT('Ctrl Pts',(-0.115254344789724,0.104461685875046,
-0.237354688200212));
#81177=CARTESIAN_POINT('Ctrl Pts',(-0.115303263032921,0.104407688139778,
-0.237349442265415));
#81178=CARTESIAN_POINT('Ctrl Pts',(-0.115400240900896,0.104300489165329,
-0.237339031225641));
#81179=CARTESIAN_POINT('Ctrl Pts',(-0.115448301721761,0.104247289027779,
-0.237333866172464));
#81180=CARTESIAN_POINT('Ctrl Pts',(-0.115544221827175,0.104140964154906,
-0.237323546735965));
#81181=CARTESIAN_POINT('Ctrl Pts',(-0.115592081296024,0.104087839608585,
-0.237318392362079));
#81182=CARTESIAN_POINT('Ctrl Pts',(-0.115688211050713,0.103980986438307,
-0.237308028344029));
#81183=CARTESIAN_POINT('Ctrl Pts',(-0.115736480577164,0.103927257157961,
-0.237302818669999));
#81184=CARTESIAN_POINT('Ctrl Pts',(-0.117098131177028,0.10240946549878,
-0.237155698925889));
#81185=CARTESIAN_POINT('Ctrl Pts',(-0.118383605708921,0.100920722324515,
-0.237012642916754));
#81186=CARTESIAN_POINT('Ctrl Pts',(-0.124009026173209,0.0941503677472277,
-0.236367264788718));
#81187=CARTESIAN_POINT('Ctrl Pts',(-0.12802564726391,0.0886111735369072,
-0.235852578010242));
#81188=CARTESIAN_POINT('Ctrl Pts',(-0.136232845254982,0.0755646620245248,
-0.234671654804108));
#81189=CARTESIAN_POINT('Ctrl Pts',(-0.14019241443196,0.0679373527464534,
-0.234001868060932));
#81190=CARTESIAN_POINT('Ctrl Pts',(-0.145400353804564,0.0554862429682903,
-0.232963939940484));
#81191=CARTESIAN_POINT('Ctrl Pts',(-0.147081964161305,0.0508614987340524,
-0.23258986046351));
#81192=CARTESIAN_POINT('Ctrl Pts',(-0.148894400814737,0.0450296775245204,
-0.232137950298299));
#81193=CARTESIAN_POINT('Ctrl Pts',(-0.149234053959582,0.0438909081540693,
-0.232050627790585));
#81194=CARTESIAN_POINT('Ctrl Pts',(-0.149753378550969,0.0420739822696501,
-0.231912881457015));
#81195=CARTESIAN_POINT('Ctrl Pts',(-0.149941562166702,0.0413983376266898,
-0.231862003485077));
#81196=CARTESIAN_POINT('Ctrl Pts',(-0.150296267755695,0.0400906663571473,
-0.231764226763451));
#81197=CARTESIAN_POINT('Ctrl Pts',(-0.150463385272501,0.0394588309787067,
-0.231717298211734));
#81198=CARTESIAN_POINT('Ctrl Pts',(-0.150866375972795,0.0378954156587527,
-0.231601915238833));
#81199=CARTESIAN_POINT('Ctrl Pts',(-0.151097613494102,0.0369626466520453,
-0.231533718070885));
#81200=CARTESIAN_POINT('Ctrl Pts',(-0.15157997871462,0.0349366646199434,
-0.231386862628883));
#81201=CARTESIAN_POINT('Ctrl Pts',(-0.151827958302424,0.033842750092484,
-0.231308365104121));
#81202=CARTESIAN_POINT('Ctrl Pts',(-0.154371560420178,0.0220309853340326,
-0.230468374167616));
#81203=CARTESIAN_POINT('Ctrl Pts',(-0.155540279718414,0.011100565239248,
-0.229756731682557));
#81204=CARTESIAN_POINT('Ctrl Pts',(-0.155549939620994,0.000137054387354205,
-0.229033329119584));
#81205=CARTESIAN_POINT('Ctrl Pts',(-0.155549939882158,0.000136757657850698,
-0.229033309540554));
#81206=CARTESIAN_POINT('Ctrl Pts',(-0.155557403485862,-0.0083524423307012,
-0.228473168697887));
#81207=CARTESIAN_POINT('Ctrl Pts',(-0.154869933188093,-0.0168271466045379,
-0.227908318305866));
#81208=CARTESIAN_POINT('Ctrl Pts',(-0.153243276817333,-0.0267340190266168,
-0.22721470303172));
#81209=CARTESIAN_POINT('Ctrl Pts',(-0.15296901012999,-0.0282611272572615,
-0.227106867729416));
#81210=CARTESIAN_POINT('Ctrl Pts',(-0.152453204345113,-0.0309051481942851,
-0.226918411679549));
#81211=CARTESIAN_POINT('Ctrl Pts',(-0.152222112306578,-0.0320239926151563,
-0.226838116476382));
#81212=CARTESIAN_POINT('Ctrl Pts',(-0.151733107294955,-0.0342665390317804,
-0.2266760134888));
#81213=CARTESIAN_POINT('Ctrl Pts',(-0.151474984114997,-0.0353901201575002,
-0.226594203765093));
#81214=CARTESIAN_POINT('Ctrl Pts',(-0.150955709809273,-0.0375406282955948,
-0.226436434284313));
#81215=CARTESIAN_POINT('Ctrl Pts',(-0.150696506976857,-0.0385679631268124,
-0.226360540991574));
#81216=CARTESIAN_POINT('Ctrl Pts',(-0.149985613206859,-0.0412689133903112,
-0.226159582701926));
#81217=CARTESIAN_POINT('Ctrl Pts',(-0.149516417080251,-0.0429377218322032,
-0.226033962908637));
#81218=CARTESIAN_POINT('Ctrl Pts',(-0.147647967485752,-0.0491809071161105,
-0.225558315230642));
#81219=CARTESIAN_POINT('Ctrl Pts',(-0.146065979461878,-0.0536973441504225,
-0.225202529143145));
#81220=CARTESIAN_POINT('Ctrl Pts',(-0.139888913410187,-0.0690279396012791,
-0.223953633819794));
#81221=CARTESIAN_POINT('Ctrl Pts',(-0.134279465761447,-0.079389786415519,
-0.223032841083095));
#81222=CARTESIAN_POINT('Ctrl Pts',(-0.125612159491976,-0.0918093520851595,
-0.221871110024715));
#81223=CARTESIAN_POINT('Ctrl Pts',(-0.123574478575888,-0.0945342439882163,
-0.221612471314857));
#81224=CARTESIAN_POINT('Ctrl Pts',(-0.120347638588512,-0.0985665013289709,
-0.22122626320443));
#81225=CARTESIAN_POINT('Ctrl Pts',(-0.119222955075185,-0.09992395591849,
-0.221095619837041));
#81226=CARTESIAN_POINT('Ctrl Pts',(-0.117538262149019,-0.10188837115776,
-0.220905977802767));
#81227=CARTESIAN_POINT('Ctrl Pts',(-0.116996153766251,-0.102510405967401,
-0.220845839183806));
#81228=CARTESIAN_POINT('Ctrl Pts',(-0.116031795710695,-0.103599329503717,
-0.220740449489436));
#81229=CARTESIAN_POINT('Ctrl Pts',(-0.115611629324614,-0.104068006141586,
-0.220695054914599));
#81230=CARTESIAN_POINT('Ctrl Pts',(-0.114670355893549,-0.10510521719659,
-0.220594519134982));
#81231=CARTESIAN_POINT('Ctrl Pts',(-0.114147853103979,-0.105672441541926,
-0.220539482272171));
#81232=CARTESIAN_POINT('Ctrl Pts',(-0.112580394799073,-0.107348867415279,
-0.220376566581818));
#81233=CARTESIAN_POINT('Ctrl Pts',(-0.111523299424275,-0.108446663233632,
-0.220269545700896));
#81234=CARTESIAN_POINT('Ctrl Pts',(-0.102194224272893,-0.117854217550899,
-0.219347532677652));
#81235=CARTESIAN_POINT('Ctrl Pts',(-0.0930221980872955,-0.125220719277211,
-0.218589637170017));
#81236=CARTESIAN_POINT('Ctrl Pts',(-0.0785111661517927,-0.134392610567397,
-0.217455164562992));
#81237=CARTESIAN_POINT('Ctrl Pts',(-0.0737652996666542,-0.137054919197883,
-0.217093281842978));
#81238=CARTESIAN_POINT('Ctrl Pts',(-0.0656320267208734,-0.141072478193257,
-0.21647742071298));
#81239=CARTESIAN_POINT('Ctrl Pts',(-0.0623188670872072,-0.142567045411504,
-0.216227710838994));
#81240=CARTESIAN_POINT('Ctrl Pts',(-0.0575372971903637,-0.144525479932043,
-0.215867086318529));
#81241=CARTESIAN_POINT('Ctrl Pts',(-0.0561095000501191,-0.145085763008879,
-0.215759378120908));
#81242=CARTESIAN_POINT('Ctrl Pts',(-0.0536049651461639,-0.146026070938215,
-0.215570273908284));
#81243=CARTESIAN_POINT('Ctrl Pts',(-0.052531877187648,-0.146415530034946,
-0.215489197142546));
#81244=CARTESIAN_POINT('Ctrl Pts',(-0.0502974488675162,-0.147198752444298,
-0.21532021353111));
#81245=CARTESIAN_POINT('Ctrl Pts',(-0.049135548228123,-0.147590663070567,
-0.215232252251104));
#81246=CARTESIAN_POINT('Ctrl Pts',(-0.0460916251194266,-0.148577455324181,
-0.215001514945841));
#81247=CARTESIAN_POINT('Ctrl Pts',(-0.0442027535375522,-0.149150306923946,
-0.214858036415914));
#81248=CARTESIAN_POINT('Ctrl Pts',(-0.034276544533934,-0.151955587125157,
-0.214102143810755));
#81249=CARTESIAN_POINT('Ctrl Pts',(-0.0260813924090781,-0.153574415346355,
-0.213470539638956));
#81250=CARTESIAN_POINT('Ctrl Pts',(-0.00939294721645679,-0.155496443600946,
-0.212176306844333));
#81251=CARTESIAN_POINT('Ctrl Pts',(-0.000923772004820798,-0.155777146693495,
-0.211515546075902));
#81252=CARTESIAN_POINT('Ctrl Pts',(0.010101252058171,-0.155243078568984,
-0.210672504753077));
#81253=CARTESIAN_POINT('Ctrl Pts',(0.0126729175716424,-0.155054337058813,
-0.210477167404917));
#81254=CARTESIAN_POINT('Ctrl Pts',(0.0170406186608072,-0.154624376046576,
-0.210148806440922));
#81255=CARTESIAN_POINT('Ctrl Pts',(0.0188392632569873,-0.15441555379036,
-0.21001457408816));
#81256=CARTESIAN_POINT('Ctrl Pts',(0.0214516866833292,-0.154065921958476,
-0.209821426830301));
#81257=CARTESIAN_POINT('Ctrl Pts',(0.0222685642728098,-0.153949973358863,
-0.209761291640913));
#81258=CARTESIAN_POINT('Ctrl Pts',(0.0237069678870701,-0.153734115796125,
-0.209655905590652));
#81259=CARTESIAN_POINT('Ctrl Pts',(0.0243288589255325,-0.153636927062771,
-0.209610511268554));
#81260=CARTESIAN_POINT('Ctrl Pts',(0.0257114010003854,-0.153412258696651,
-0.20950997314202));
#81261=CARTESIAN_POINT('Ctrl Pts',(0.0264717131956665,-0.153282894437996,
-0.209454933711705));
#81262=CARTESIAN_POINT('Ctrl Pts',(0.0287315571414647,-0.152881074107881,
-0.209292002426701));
#81263=CARTESIAN_POINT('Ctrl Pts',(0.0302281324291441,-0.15259222017744,
-0.209184968762462));
#81264=CARTESIAN_POINT('Ctrl Pts',(0.0432066406658109,-0.149888790417328,
-0.208262390664449));
#81265=CARTESIAN_POINT('Ctrl Pts',(0.0543871075947379,-0.146203925198292,
-0.207504017805518));
#81266=CARTESIAN_POINT('Ctrl Pts',(0.0699832823718536,-0.139023960870183,
-0.206369329884208));
#81267=CARTESIAN_POINT('Ctrl Pts',(0.074795790312722,-0.136495071689835,
-0.206007773205395));
#81268=CARTESIAN_POINT('Ctrl Pts',(0.0825877823424298,-0.131864509135969,
-0.205392399099184));
#81269=CARTESIAN_POINT('Ctrl Pts',(0.0856435118087766,-0.129900639144443,
-0.20514284075657));
#81270=CARTESIAN_POINT('Ctrl Pts',(0.0898877077246374,-0.126958079102895,
-0.204782396098733));
#81271=CARTESIAN_POINT('Ctrl Pts',(0.0911348435151286,-0.126065831426822,
-0.204674711698476));
#81272=CARTESIAN_POINT('Ctrl Pts',(0.0932870104334786,-0.124477464814844,
-0.204485634928572));
#81273=CARTESIAN_POINT('Ctrl Pts',(0.0941979615284775,-0.123789537039849,
-0.204404561525463));
#81274=CARTESIAN_POINT('Ctrl Pts',(0.0960716829542772,-0.122341890440374,
-0.204235571095911));
#81275=CARTESIAN_POINT('Ctrl Pts',(0.097033201752121,-0.121580689344235,
-0.204147599498362));
#81276=CARTESIAN_POINT('Ctrl Pts',(0.0995190138411277,-0.119564487308645,
-0.203916803451899));
#81277=CARTESIAN_POINT('Ctrl Pts',(0.101028545417739,-0.11829172874913,
-0.2037732758329));
#81278=CARTESIAN_POINT('Ctrl Pts',(0.108806358007299,-0.111476398101642,
-0.203015445949056));
#81279=CARTESIAN_POINT('Ctrl Pts',(0.114643112071185,-0.105464332792143,
-0.202381825626085));
#81280=CARTESIAN_POINT('Ctrl Pts',(0.125338765815816,-0.0925051439589563,
-0.201087160056976));
#81281=CARTESIAN_POINT('Ctrl Pts',(0.130171555052273,-0.0855708806996168,
-0.200428109296607));
#81282=CARTESIAN_POINT('Ctrl Pts',(0.135713906457741,-0.0760537205247465,
-0.199586974583617));
#81283=CARTESIAN_POINT('Ctrl Pts',(0.136954342961365,-0.0737966279380717,
-0.199391877921633));
#81284=CARTESIAN_POINT('Ctrl Pts',(0.13896982461374,-0.0699032364407014,
-0.199063874439057));
#81285=CARTESIAN_POINT('Ctrl Pts',(0.13977337725737,-0.0682823430078759,
-0.198929762072994));
#81286=CARTESIAN_POINT('Ctrl Pts',(0.140901889114958,-0.0659025063917623,
-0.198736753539964));
#81287=CARTESIAN_POINT('Ctrl Pts',(0.141249341834933,-0.0651544796425545,
-0.198676639442777));
#81288=CARTESIAN_POINT('Ctrl Pts',(0.141851440910951,-0.0638307713815762,
-0.198571275867086));
#81289=CARTESIAN_POINT('Ctrl Pts',(0.142108563670739,-0.063256263270361,
-0.198525883161269));
#81290=CARTESIAN_POINT('Ctrl Pts',(0.142673062062243,-0.0619741475840294,
-0.198425330856019));
#81291=CARTESIAN_POINT('Ctrl Pts',(0.142978669216799,-0.0612657965183183,
-0.198370275827079));
#81292=CARTESIAN_POINT('Ctrl Pts',(0.143872750261244,-0.0591503203956359,
-0.198207249253159));
#81293=CARTESIAN_POINT('Ctrl Pts',(0.144445832949263,-0.0577367341288294,
-0.198100137394947));
#81294=CARTESIAN_POINT('Ctrl Pts',(0.149243661986275,-0.0453834110946092,
-0.197177911628806));
#81295=CARTESIAN_POINT('Ctrl Pts',(0.152240098771118,-0.0340052756533205,
-0.196419897912158));
#81296=CARTESIAN_POINT('Ctrl Pts',(0.154711781701462,-0.0170180312739999,
-0.195285447231123));
#81297=CARTESIAN_POINT('Ctrl Pts',(0.155211901335296,-0.0116020601934807,
-0.194923730210237));
#81298=CARTESIAN_POINT('Ctrl Pts',(0.155571653530076,-0.00254151124503676,
-0.194308116600976));
#81299=CARTESIAN_POINT('Ctrl Pts',(0.15558856928531,0.00109195674468064,
-0.194058483745806));
#81300=CARTESIAN_POINT('Ctrl Pts',(0.155431737667368,0.006255341675108,
-0.193697950665079));
#81301=CARTESIAN_POINT('Ctrl Pts',(0.155362513388929,0.00778739452743881,
-0.19359025458497));
#81302=CARTESIAN_POINT('Ctrl Pts',(0.155202267414991,0.0104576196889015,
-0.193401164370465));
#81303=CARTESIAN_POINT('Ctrl Pts',(0.155121344088004,0.0115962969498585,
-0.193320089341715));
#81304=CARTESIAN_POINT('Ctrl Pts',(0.154927509288578,0.0139561140712787,
-0.193151102335572));
#81305=CARTESIAN_POINT('Ctrl Pts',(0.154812675239116,0.015177011601869,
-0.193063135854482));
#81306=CARTESIAN_POINT('Ctrl Pts',(0.15447533618745,0.0183594652606682,
-0.192832368840042));
#81307=CARTESIAN_POINT('Ctrl Pts',(0.15422990957344,0.0203183116072376,
-0.192688865464766));
#81308=CARTESIAN_POINT('Ctrl Pts',(0.152751053301781,0.0305404365768638,
-0.191931976267203));
#81309=CARTESIAN_POINT('Ctrl Pts',(0.150890823824713,0.0386978005737078,
-0.191299334524039));
#81310=CARTESIAN_POINT('Ctrl Pts',(0.145850529546059,0.0547248334167432,
-0.190004878172485));
#81311=CARTESIAN_POINT('Ctrl Pts',(0.142663486355955,0.0625644903227373,
-0.189344996716908));
#81312=CARTESIAN_POINT('Ctrl Pts',(0.137694367925235,0.0724065024140782,
-0.188502935737827));
#81313=CARTESIAN_POINT('Ctrl Pts',(0.136476130166284,0.0746773592631195,
-0.188307722077662));
#81314=CARTESIAN_POINT('Ctrl Pts',(0.134307119329309,0.07848996816095,-0.187979544826952));
#81315=CARTESIAN_POINT('Ctrl Pts',(0.133384833321598,0.0800472634360736,
-0.18784537413927));
#81316=CARTESIAN_POINT('Ctrl Pts',(0.13200286608517,0.0822904993063647,
-0.187652298192771));
#81317=CARTESIAN_POINT('Ctrl Pts',(0.131564610858871,0.0829893739089262,
-0.187592173859068));
#81318=CARTESIAN_POINT('Ctrl Pts',(0.130782178517708,0.084215321979754,
-0.187486799405406));
#81319=CARTESIAN_POINT('Ctrl Pts',(0.1304403358384,0.0847438346324271,-0.187441405944234));
#81320=CARTESIAN_POINT('Ctrl Pts',(0.129672446647997,0.0859153887086811,
-0.187340860633403));
#81321=CARTESIAN_POINT('Ctrl Pts',(0.129244814978104,0.0865573526913667,
-0.187285813258311));
#81322=CARTESIAN_POINT('Ctrl Pts',(0.127957761719587,0.0884586806772202,
-0.187122833303645));
#81323=CARTESIAN_POINT('Ctrl Pts',(0.127084551779746,0.0897086624777553,
-0.187015759680114));
#81324=CARTESIAN_POINT('Ctrl Pts',(0.119334929603154,0.100461770633756,
-0.186093360613191));
#81325=CARTESIAN_POINT('Ctrl Pts',(0.11142140059385,0.109173010098291,-0.185335170467301));
#81326=CARTESIAN_POINT('Ctrl Pts',(0.102515838399332,0.116988540786228,
-0.184552126385709));
#81327=CARTESIAN_POINT('Ctrl Pts',(0.10242908212953,0.117064507564331,-0.184544504392145));
#81328=CARTESIAN_POINT('Ctrl Pts',(0.102342242826532,0.117140376613853,
-0.184536881298507));
#81329=CARTESIAN_POINT('Origin',(0.,0.,-1.10400562256037));
#81330=CARTESIAN_POINT('',(0.10234224283772,0.117140376604078,-0.100698721018058));
#81331=CARTESIAN_POINT('',(0.102342241743611,0.11714037755997,-0.114635995609957));
#81332=CARTESIAN_POINT('',(0.10234224283772,0.117140376604078,-1.10400562256037));
#81333=CARTESIAN_POINT('',(-0.155549976200755,-8.60461765890906E-5,-0.145194377445451));
#81334=CARTESIAN_POINT('Ctrl Pts',(-0.15554997620071,-8.60462574926153E-5,
-0.145194377439629));
#81335=CARTESIAN_POINT('Ctrl Pts',(-0.155547169018751,-0.00516072468918725,
-0.144829200911433));
#81336=CARTESIAN_POINT('Ctrl Pts',(-0.155296045436501,-0.010228371777148,
-0.144464024383237));
#81337=CARTESIAN_POINT('Ctrl Pts',(-0.154798544359905,-0.0152713183469712,
-0.144098847855041));
#81338=CARTESIAN_POINT('Ctrl Pts',(-0.153793713525852,-0.0254568404417424,
-0.143361280334756));
#81339=CARTESIAN_POINT('Ctrl Pts',(-0.151775550772244,-0.0355806132571192,
-0.142623712814471));
#81340=CARTESIAN_POINT('Ctrl Pts',(-0.148768856287275,-0.0454271933865166,
-0.141886145294187));
#81341=CARTESIAN_POINT('Ctrl Pts',(-0.145755023185923,-0.0552971516671018,
-0.141146826611084));
#81342=CARTESIAN_POINT('Ctrl Pts',(-0.141748088156632,-0.0648876693193305,
-0.140407507927983));
#81343=CARTESIAN_POINT('Ctrl Pts',(-0.13682468791801,-0.0739919406161174,
-0.13966818924488));
#81344=CARTESIAN_POINT('Ctrl Pts',(-0.13192416200287,-0.083053913087579,
-0.13893230546731));
#81345=CARTESIAN_POINT('Ctrl Pts',(-0.126116108676144,-0.091633325525222,
-0.138196421689739));
#81346=CARTESIAN_POINT('Ctrl Pts',(-0.119522825148394,-0.0995494689516038,
-0.137460537912168));
#81347=CARTESIAN_POINT('Ctrl Pts',(-0.112883378136513,-0.107521037987988,
-0.1367195017763));
#81348=CARTESIAN_POINT('Ctrl Pts',(-0.105448260210238,-0.114819275876618,
-0.135978465640433));
#81349=CARTESIAN_POINT('Ctrl Pts',(-0.0973821576493404,-0.121295168376811,
-0.135237429504565));
#81350=CARTESIAN_POINT('Ctrl Pts',(-0.0893160550884423,-0.127771060877005,
-0.134496393368697));
#81351=CARTESIAN_POINT('Ctrl Pts',(-0.0806197845170057,-0.133424117721121,
-0.133755357232829));
#81352=CARTESIAN_POINT('Ctrl Pts',(-0.0714869563426234,-0.138149982167454,
-0.133014321096961));
#81353=CARTESIAN_POINT('Ctrl Pts',(-0.0623968021115963,-0.142853764596275,
-0.132276747517651));
#81354=CARTESIAN_POINT('Ctrl Pts',(-0.0528066258091951,-0.146673991821844,
-0.131539173938341));
#81355=CARTESIAN_POINT('Ctrl Pts',(-0.0429106352096175,-0.149514146106337,
-0.130801600359031));
#81356=CARTESIAN_POINT('Ctrl Pts',(-0.0329912509565894,-0.152361014381149,
-0.130062283190685));
#81357=CARTESIAN_POINT('Ctrl Pts',(-0.0227654554255227,-0.154222772693214,
-0.129322966022339));
#81358=CARTESIAN_POINT('Ctrl Pts',(-0.0124484318150597,-0.155051085276259,
-0.128583648853993));
#81359=CARTESIAN_POINT('Ctrl Pts',(-0.00217923318024209,-0.155875558183192,
-0.127847758819955));
#81360=CARTESIAN_POINT('Ctrl Pts',(0.00817942026916348,-0.155676067402559,
-0.127111868785917));
#81361=CARTESIAN_POINT('Ctrl Pts',(0.0184093627804832,-0.154456783153141,
-0.126375978751879));
#81362=CARTESIAN_POINT('Ctrl Pts',(0.0287107685240648,-0.153228981358937,
-0.12563494801638));
#81363=CARTESIAN_POINT('Ctrl Pts',(0.0388807135570937,-0.150967182408244,
-0.12489391728088));
#81364=CARTESIAN_POINT('Ctrl Pts',(0.0487045426096044,-0.147728365689157,
-0.12415288654538));
#81365=CARTESIAN_POINT('Ctrl Pts',(0.058528371662115,-0.14448954897007,
-0.12341185580988));
#81366=CARTESIAN_POINT('Ctrl Pts',(0.0680052289217426,-0.140274132387235,
-0.12267082507438));
#81367=CARTESIAN_POINT('Ctrl Pts',(0.0769421623588443,-0.135187670116565,
-0.121929794338881));
#81368=CARTESIAN_POINT('Ctrl Pts',(0.0858370381162951,-0.130125145005352,
-0.121192250933068));
#81369=CARTESIAN_POINT('Ctrl Pts',(0.094263193245769,-0.124162160084575,
-0.120454707527255));
#81370=CARTESIAN_POINT('Ctrl Pts',(0.102033927875157,-0.117409028879244,
-0.119717164121442));
#81371=CARTESIAN_POINT('Ctrl Pts',(0.109823430288772,-0.11063958759316,
-0.118977839409722));
#81372=CARTESIAN_POINT('Ctrl Pts',(0.116953545084801,-0.103076675214026,
-0.118238514698002));
#81373=CARTESIAN_POINT('Ctrl Pts',(0.123266536901705,-0.0948744611592639,
-0.117499189986282));
#81374=CARTESIAN_POINT('Ctrl Pts',(0.12954994540641,-0.0867106835014012,
-0.116763329824239));
#81375=CARTESIAN_POINT('Ctrl Pts',(0.135023300833802,-0.0779143198630106,
-0.116027469662196));
#81376=CARTESIAN_POINT('Ctrl Pts',(0.139571306722132,-0.068670611180305,
-0.115291609500154));
#81377=CARTESIAN_POINT('Ctrl Pts',(0.144151431740859,-0.0593616211651135,
-0.114550552513595));
#81378=CARTESIAN_POINT('Ctrl Pts',(0.147792654371947,-0.0495997892919083,
-0.113809495527036));
#81379=CARTESIAN_POINT('Ctrl Pts',(0.150425869185099,-0.0395962167373015,
-0.113068438540477));
#81380=CARTESIAN_POINT('Ctrl Pts',(0.153059083998252,-0.0295926441826946,
-0.112327381553918));
#81381=CARTESIAN_POINT('Ctrl Pts',(0.154684175489864,-0.0193482767603506,
-0.11158632456736));
#81382=CARTESIAN_POINT('Ctrl Pts',(0.155284614072203,-0.00908246290644956,
-0.110845267580801));
#81383=CARTESIAN_POINT('Ctrl Pts',(0.155882256621659,0.00113554663581544,
-0.110107661437948));
#81384=CARTESIAN_POINT('Ctrl Pts',(0.155469251660693,0.0114507651553898,
-0.109370055295096));
#81385=CARTESIAN_POINT('Ctrl Pts',(0.154036462806462,0.0216464922348542,
-0.108632449152243));
#81386=CARTESIAN_POINT('Ctrl Pts',(0.152605995913413,0.0318256962359578,
-0.107896038365445));
#81387=CARTESIAN_POINT('Ctrl Pts',(0.150159064761957,0.0418848710726706,
-0.107159627578647));
#81388=CARTESIAN_POINT('Ctrl Pts',(0.146738469077704,0.0516103109148915,
-0.106423216791849));
#81389=CARTESIAN_POINT('Ctrl Pts',(0.143321329611764,0.0613259240349885,
-0.105687550084937));
#81390=CARTESIAN_POINT('Ctrl Pts',(0.138932767306006,0.0707075924762563,
-0.104951883378026));
#81391=CARTESIAN_POINT('Ctrl Pts',(0.133665088257766,0.0795578197353582,
-0.104216216671114));
#81392=CARTESIAN_POINT('Ctrl Pts',(0.128388725433959,0.0884226366052783,
-0.103479337216707));
#81393=CARTESIAN_POINT('Ctrl Pts',(0.122230843509559,0.0967534740597384,
-0.102742457762299));
#81394=CARTESIAN_POINT('Ctrl Pts',(0.115328226724701,0.104380087279787,
-0.102005578307892));
#81395=CARTESIAN_POINT('Ctrl Pts',(0.11124762484323,0.108888692237149,-0.101569959211281));
#81396=CARTESIAN_POINT('Ctrl Pts',(0.106907560372334,0.11315178744888,-0.101134340114669));
#81397=CARTESIAN_POINT('Ctrl Pts',(0.10234224283772,0.117140376604078,-0.100698721018058));
#81398=CARTESIAN_POINT('Ctrl Pts',(0.10234224283772,0.117140376604078,-0.170697633677947));
#81399=CARTESIAN_POINT('Ctrl Pts',(0.0945586197976017,0.123940708500068,
-0.169959344960156));
#81400=CARTESIAN_POINT('Ctrl Pts',(0.0861005207429198,0.129956556556732,
-0.169221056242365));
#81401=CARTESIAN_POINT('Ctrl Pts',(0.0771519734397198,0.135068040240305,
-0.168482767524574));
#81402=CARTESIAN_POINT('Ctrl Pts',(0.0682034261365199,0.140179523923879,
-0.167744478806783));
#81403=CARTESIAN_POINT('Ctrl Pts',(0.05876529787386,0.144386293971583,-0.167006190088992));
#81404=CARTESIAN_POINT('Ctrl Pts',(0.049042847800632,0.147616400103796,
-0.166267901371201));
#81405=CARTESIAN_POINT('Ctrl Pts',(0.0393299004762808,0.15084334912158,
-0.16553033425879));
#81406=CARTESIAN_POINT('Ctrl Pts',(0.0292610015856663,0.153119533717959,
-0.16479276714638));
#81407=CARTESIAN_POINT('Ctrl Pts',(0.0190430417864429,0.154379937360785,
-0.164055200033969));
#81408=CARTESIAN_POINT('Ctrl Pts',(0.00880081501473634,0.155643334378132,
-0.163315881248898));
#81409=CARTESIAN_POINT('Ctrl Pts',(-0.00159027922619605,0.155885859586032,
-0.162576562463828));
#81410=CARTESIAN_POINT('Ctrl Pts',(-0.011910146200751,0.155093361938791,
-0.161837243678757));
#81411=CARTESIAN_POINT('Ctrl Pts',(-0.0221820614633852,0.154304546666426,
-0.161101360170661));
#81412=CARTESIAN_POINT('Ctrl Pts',(-0.0323824797595626,0.152490373977825,
-0.160365476662565));
#81413=CARTESIAN_POINT('Ctrl Pts',(-0.0422965644458576,0.149689021428017,
-0.159629593154469));
#81414=CARTESIAN_POINT('Ctrl Pts',(-0.0522800710443302,0.146868052821171,
-0.158888556730911));
#81415=CARTESIAN_POINT('Ctrl Pts',(-0.0619723009048204,0.143046271088191,
-0.158147520307353));
#81416=CARTESIAN_POINT('Ctrl Pts',(-0.0711701194738238,0.138313472207452,
-0.157406483883795));
#81417=CARTESIAN_POINT('Ctrl Pts',(-0.0803679380428271,0.133580673326713,
-0.156665447460237));
#81418=CARTESIAN_POINT('Ctrl Pts',(-0.0890705651706336,0.127937403751066,
-0.155924411036679));
#81419=CARTESIAN_POINT('Ctrl Pts',(-0.0971038891700634,0.121518053012909,
-0.155183374613121));
#81420=CARTESIAN_POINT('Ctrl Pts',(-0.105000973143479,0.115207570348742,
-0.154454905692334));
#81421=CARTESIAN_POINT('Ctrl Pts',(-0.112313136123349,0.108097583610356,
-0.153726436771547));
#81422=CARTESIAN_POINT('Ctrl Pts',(-0.11887533097625,0.100321773236357,
-0.15299796785076));
#81423=CARTESIAN_POINT('Ctrl Pts',(-0.125427954384414,0.0925573044547588,
-0.152270561455572));
#81424=CARTESIAN_POINT('Ctrl Pts',(-0.131232096894198,0.0841295966894995,
-0.151543155060384));
#81425=CARTESIAN_POINT('Ctrl Pts',(-0.136159342815408,0.0752092804384954,
-0.150815748665196));
#81426=CARTESIAN_POINT('Ctrl Pts',(-0.141082092447257,0.0662971042973398,
-0.150089006054542));
#81427=CARTESIAN_POINT('Ctrl Pts',(-0.145129060671767,0.0568940369707911,
-0.149362263443888));
#81428=CARTESIAN_POINT('Ctrl Pts',(-0.14821697669958,0.0471967193567106,
-0.148635520833233));
#81429=CARTESIAN_POINT('Ctrl Pts',(-0.151310928033582,0.0374804484160237,
-0.147907357810192));
#81430=CARTESIAN_POINT('Ctrl Pts',(-0.153441825858717,0.0274696985169037,
-0.147179194787151));
#81431=CARTESIAN_POINT('Ctrl Pts',(-0.154576475344867,0.0173757235808376,
-0.14645103176411));
#81432=CARTESIAN_POINT('Ctrl Pts',(-0.155229196476361,0.0115690398234625,
-0.146032146991224));
#81433=CARTESIAN_POINT('Ctrl Pts',(-0.155553196245258,0.0057349892904951,
-0.145613262218337));
#81434=CARTESIAN_POINT('Ctrl Pts',(-0.155549976200755,-8.60461765879318E-5,
-0.145194377445451));
#81435=CARTESIAN_POINT('Ctrl Pts',(0.102342242826532,0.117140376613853,
-0.184536881298507));
#81436=CARTESIAN_POINT('Ctrl Pts',(0.0983366947192182,0.120639911009267,
-0.184185258620294));
#81437=CARTESIAN_POINT('Ctrl Pts',(0.0941544952938237,0.123931513579687,
-0.18383113563115));
#81438=CARTESIAN_POINT('Ctrl Pts',(0.0868465589662623,0.129099457452717,
-0.183223466831916));
#81439=CARTESIAN_POINT('Ctrl Pts',(0.0838087104185499,0.131091919577572,
-0.18297387024936));
#81440=CARTESIAN_POINT('Ctrl Pts',(0.0793931506215579,0.133771752444894,
-0.182613380228226));
#81441=CARTESIAN_POINT('Ctrl Pts',(0.0780705466443553,0.134547922952287,
-0.182505689851712));
#81442=CARTESIAN_POINT('Ctrl Pts',(0.0757437695338512,0.135867534636086,
-0.182316606225206));
#81443=CARTESIAN_POINT('Ctrl Pts',(0.0747446708265066,0.136419718694302,
-0.182235532013308));
#81444=CARTESIAN_POINT('Ctrl Pts',(0.0726598507195555,0.137542184176541,
-0.182066543407407));
#81445=CARTESIAN_POINT('Ctrl Pts',(0.0715732851402894,0.138110720186298,
-0.181978574477041));
#81446=CARTESIAN_POINT('Ctrl Pts',(0.0687201973730012,0.139560863240983,
-0.18174779347322));
#81447=CARTESIAN_POINT('Ctrl Pts',(0.0669434637725879,0.140421764952022,
-0.181604278399122));
#81448=CARTESIAN_POINT('Ctrl Pts',(0.0575588653788898,0.144750410347913,
-0.180846929836045));
#81449=CARTESIAN_POINT('Ctrl Pts',(0.0496981348061524,0.147633863069435,
-0.180213810080176));
#81450=CARTESIAN_POINT('Ctrl Pts',(0.0347126592904053,0.151797900082725,
-0.179015456334295));
#81451=CARTESIAN_POINT('Ctrl Pts',(0.0276550827633492,0.153240876802733,
-0.178454710886467));
#81452=CARTESIAN_POINT('Ctrl Pts',(0.0156657943747679,0.154836675342816,
-0.177524870698505));
#81453=CARTESIAN_POINT('Ctrl Pts',(0.0107801874139766,0.155253376498215,
-0.177152336470884));
#81454=CARTESIAN_POINT('Ctrl Pts',(0.00472708396739653,0.155482456483989,
-0.176704406392737));
#81455=CARTESIAN_POINT('Ctrl Pts',(0.00357108416457462,0.155513302215766,
-0.176619478851091));
#81456=CARTESIAN_POINT('Ctrl Pts',(0.00172046394156059,0.155542035241058,
-0.176484616137419));
#81457=CARTESIAN_POINT('Ctrl Pts',(0.00102604211302602,0.155548166209317,
-0.176434257596174));
#81458=CARTESIAN_POINT('Ctrl Pts',(-0.000318162992916625,0.155551031645879,
-0.176337285112024));
#81459=CARTESIAN_POINT('Ctrl Pts',(-0.000967919269937373,0.155548345629575,
-0.176290643048398));
#81460=CARTESIAN_POINT('Ctrl Pts',(-0.00243424900611269,0.155533095634588,
-0.176185871312739));
#81461=CARTESIAN_POINT('Ctrl Pts',(-0.00325079182791444,0.155518172041095,
-0.176127868452708));
#81462=CARTESIAN_POINT('Ctrl Pts',(-0.00618614913599467,0.155441394310472,
-0.175920457760872));
#81463=CARTESIAN_POINT('Ctrl Pts',(-0.00830387491257301,0.155342660882586,
-0.175772883948787));
#81464=CARTESIAN_POINT('Ctrl Pts',(-0.0200681731245363,0.154552890995048,
-0.174961265175642));
#81465=CARTESIAN_POINT('Ctrl Pts',(-0.0296369762449393,0.153006601822503,
-0.174330769129431));
#81466=CARTESIAN_POINT('Ctrl Pts',(-0.0471386380210022,0.148473613491827,
-0.173138717343726));
#81467=CARTESIAN_POINT('Ctrl Pts',(-0.0550910692268391,0.14571003948883,
-0.172580904087223));
#81468=CARTESIAN_POINT('Ctrl Pts',(-0.0649829478118983,0.141346425787419,
-0.171836835981849));
#81469=CARTESIAN_POINT('Ctrl Pts',(-0.0671621333761477,0.140324061935305,
-0.171669683799163));
#81470=CARTESIAN_POINT('Ctrl Pts',(-0.0704945267629355,0.138665263978037,
-0.171408504112053));
#81471=CARTESIAN_POINT('Ctrl Pts',(-0.0716649068496607,0.138064023826466,
-0.17131568688325));
#81472=CARTESIAN_POINT('Ctrl Pts',(-0.0738214192480146,0.136921385507045,
-0.171142554245235));
#81473=CARTESIAN_POINT('Ctrl Pts',(-0.0748095846125761,0.136383993481202,
-0.17106238388637));
#81474=CARTESIAN_POINT('Ctrl Pts',(-0.0769950265987758,0.135164591590456,
-0.170883156048896));
#81475=CARTESIAN_POINT('Ctrl Pts',(-0.0781892312990778,0.134477302263918,
-0.170783915213729));
#81476=CARTESIAN_POINT('Ctrl Pts',(-0.0812078041497835,0.132686251089956,
-0.170529638504634));
#81477=CARTESIAN_POINT('Ctrl Pts',(-0.0830188421547394,0.131560707291047,
-0.170373831268357));
#81478=CARTESIAN_POINT('Ctrl Pts',(-0.0938167285571004,0.124538175138603,
-0.169424580496919));
#81479=CARTESIAN_POINT('Ctrl Pts',(-0.102194137706582,0.117760838976589,
-0.168598645922293));
#81480=CARTESIAN_POINT('Ctrl Pts',(-0.114105183857023,0.105889905119983,
-0.167295493259657));
#81481=CARTESIAN_POINT('Ctrl Pts',(-0.11815117015547,0.101355676680991,
-0.16682461843477));
#81482=CARTESIAN_POINT('Ctrl Pts',(-0.123907203235406,0.0940905308038684,
-0.166120131438881));
#81483=CARTESIAN_POINT('Ctrl Pts',(-0.125814956920619,0.0915238935001316,
-0.165879952406257));
#81484=CARTESIAN_POINT('Ctrl Pts',(-0.128224288826043,0.0880645836709176,
-0.165569245734799));
#81485=CARTESIAN_POINT('Ctrl Pts',(-0.128797990164475,0.0872233742701828,
-0.165494670041611));
#81486=CARTESIAN_POINT('Ctrl Pts',(-0.129732545586649,0.0858237205618625,
-0.165372272970573));
#81487=CARTESIAN_POINT('Ctrl Pts',(-0.13009814506523,0.0852685000675042,
-0.165324152084376));
#81488=CARTESIAN_POINT('Ctrl Pts',(-0.130832673815881,0.0841372794266802,
-0.165227008930521));
#81489=CARTESIAN_POINT('Ctrl Pts',(-0.131201383551625,0.0835611592153828,
-0.165178000553216));
#81490=CARTESIAN_POINT('Ctrl Pts',(-0.132157477900669,0.0820453020307706,
-0.165050214847673));
#81491=CARTESIAN_POINT('Ctrl Pts',(-0.132738654331504,0.0811016669485627,
-0.164971826779628));
#81492=CARTESIAN_POINT('Ctrl Pts',(-0.135270554436817,0.0768905748567535,
-0.164626739381644));
#81493=CARTESIAN_POINT('Ctrl Pts',(-0.137111243809965,0.0735581110413254,
-0.164366137841692));
#81494=CARTESIAN_POINT('Ctrl Pts',(-0.142594652787796,0.0627080842823455,
-0.163545835545655));
#81495=CARTESIAN_POINT('Ctrl Pts',(-0.14575522831244,0.0549633442823664,
-0.163001376773668));
#81496=CARTESIAN_POINT('Ctrl Pts',(-0.150411519134649,0.0402739491853991,
-0.16198375661037));
#81497=CARTESIAN_POINT('Ctrl Pts',(-0.152083594010951,0.0334093009859926,
-0.161513883427001));
#81498=CARTESIAN_POINT('Ctrl Pts',(-0.153749516730865,0.0237568362296076,
-0.160842542147919));
#81499=CARTESIAN_POINT('Ctrl Pts',(-0.154143883005944,0.021046685002819,
-0.160652972335974));
#81500=CARTESIAN_POINT('Ctrl Pts',(-0.15462916250251,0.0169567259175699,
-0.160364502469057));
#81501=CARTESIAN_POINT('Ctrl Pts',(-0.154773563675264,0.0155837165186166,
-0.160267263016903));
#81502=CARTESIAN_POINT('Ctrl Pts',(-0.155002427330546,0.0130887562095317,
-0.160089748022903));
#81503=CARTESIAN_POINT('Ctrl Pts',(-0.155093030031646,0.0119674530359494,
-0.160009669716657));
#81504=CARTESIAN_POINT('Ctrl Pts',(-0.155263041862571,0.00953497045006591,
-0.159835257996851));
#81505=CARTESIAN_POINT('Ctrl Pts',(-0.155338019722236,0.00822357972594806,
-0.159740792791224));
#81506=CARTESIAN_POINT('Ctrl Pts',(-0.15549986499489,0.00458465720597244,
-0.159477375803979));
#81507=CARTESIAN_POINT('Ctrl Pts',(-0.155551073925404,0.0022559733692135,
-0.159307339306242));
#81508=CARTESIAN_POINT('Ctrl Pts',(-0.155546231361191,-0.00808099791623698,
-0.158545639796813));
#81509=CARTESIAN_POINT('Ctrl Pts',(-0.154924079204671,-0.0160756561186006,
-0.157937240778656));
#81510=CARTESIAN_POINT('Ctrl Pts',(-0.152324000699988,-0.0327357129707682,
-0.156636655028277));
#81511=CARTESIAN_POINT('Ctrl Pts',(-0.150213702579628,-0.0413530871017355,
-0.155944636559827));
#81512=CARTESIAN_POINT('Ctrl Pts',(-0.146383187404494,-0.052702095370091,
-0.155034449418541));
#81513=CARTESIAN_POINT('Ctrl Pts',(-0.145295929628231,-0.0556295287590152,
-0.154799915407875));
#81514=CARTESIAN_POINT('Ctrl Pts',(-0.143730082186628,-0.0594856849865002,
-0.154492999322737));
#81515=CARTESIAN_POINT('Ctrl Pts',(-0.143329297992639,-0.0604449810732597,
-0.154416819284242));
#81516=CARTESIAN_POINT('Ctrl Pts',(-0.142680896754708,-0.0619542394754681,
-0.154297316600963));
#81517=CARTESIAN_POINT('Ctrl Pts',(-0.142439656757601,-0.06250688205075,
-0.15425363362081));
#81518=CARTESIAN_POINT('Ctrl Pts',(-0.14192674836047,-0.0636634835104297,
-0.154162390320878));
#81519=CARTESIAN_POINT('Ctrl Pts',(-0.141654426030723,-0.0642671350459861,
-0.154114873846387));
#81520=CARTESIAN_POINT('Ctrl Pts',(-0.140958855831596,-0.0657830893378421,
-0.153995766082405));
#81521=CARTESIAN_POINT('Ctrl Pts',(-0.140530590315446,-0.0666930821503648,
-0.153924470699154));
#81522=CARTESIAN_POINT('Ctrl Pts',(-0.138753682158606,-0.0703755880718805,
-0.15363652308691));
#81523=CARTESIAN_POINT('Ctrl Pts',(-0.137331480573935,-0.0731120735731565,
-0.153423859740469));
#81524=CARTESIAN_POINT('Ctrl Pts',(-0.133047980982116,-0.0807873563138952,
-0.152825987949667));
#81525=CARTESIAN_POINT('Ctrl Pts',(-0.129994928632779,-0.0856136096135604,
-0.152448241417963));
#81526=CARTESIAN_POINT('Ctrl Pts',(-0.120109523062564,-0.099487927750899,
-0.151324800387112));
#81527=CARTESIAN_POINT('Ctrl Pts',(-0.112548242317941,-0.107967611537955,
-0.150584138550943));
#81528=CARTESIAN_POINT('Ctrl Pts',(-0.102427970050515,-0.11708794011791,
-0.149645511104979));
#81529=CARTESIAN_POINT('Ctrl Pts',(-0.100688527489477,-0.118587074619857,
-0.149485929661597));
#81530=CARTESIAN_POINT('Ctrl Pts',(-0.0979083465090845,-0.120877892989764,
-0.149233102559626));
#81531=CARTESIAN_POINT('Ctrl Pts',(-0.0968896782928011,-0.121695930027374,
-0.149140919895653));
#81532=CARTESIAN_POINT('Ctrl Pts',(-0.0949745517298871,-0.123194576095098,
-0.148968371894081));
#81533=CARTESIAN_POINT('Ctrl Pts',(-0.0940807706626771,-0.123878478863977,
-0.148888143909745));
#81534=CARTESIAN_POINT('Ctrl Pts',(-0.0920671148726055,-0.12538492488059,
-0.14870800729064));
#81535=CARTESIAN_POINT('Ctrl Pts',(-0.0909434940087749,-0.126202272937342,
-0.148607906154514));
#81536=CARTESIAN_POINT('Ctrl Pts',(-0.0875347503410679,-0.128612710226155,
-0.148305366956385));
#81537=CARTESIAN_POINT('Ctrl Pts',(-0.0852177466115496,-0.13015950053001,
-0.148101222246312));
#81538=CARTESIAN_POINT('Ctrl Pts',(-0.0775859401064273,-0.134963213971767,
-0.147433147069885));
#81539=CARTESIAN_POINT('Ctrl Pts',(-0.0721171409500961,-0.137962851490374,
-0.146960734050542));
#81540=CARTESIAN_POINT('Ctrl Pts',(-0.0573195635495639,-0.144958697470478,
-0.145702817273616));
#81541=CARTESIAN_POINT('Ctrl Pts',(-0.0477539703036574,-0.148385024339524,
-0.144908331901771));
#81542=CARTESIAN_POINT('Ctrl Pts',(-0.0350582461855507,-0.151576540388081,
-0.143915129893144));
#81543=CARTESIAN_POINT('Ctrl Pts',(-0.0321732767323222,-0.15221501657956,
-0.143693517212808));
#81544=CARTESIAN_POINT('Ctrl Pts',(-0.0282705475958293,-0.152962798246914,
-0.143400632601761));
#81545=CARTESIAN_POINT('Ctrl Pts',(-0.0272675433671392,-0.153144777042819,
-0.143325969967749));
#81546=CARTESIAN_POINT('Ctrl Pts',(-0.0256722250033197,-0.15341805096287,
-0.143208256255142));
#81547=CARTESIAN_POINT('Ctrl Pts',(-0.0250810693659445,-0.153515802085592,
-0.143164862627774));
#81548=CARTESIAN_POINT('Ctrl Pts',(-0.0238313213776839,-0.153715043599704,
-0.14307362265189));
#81549=CARTESIAN_POINT('Ctrl Pts',(-0.0231726129600604,-0.153815722700847,
-0.143025824853917));
#81550=CARTESIAN_POINT('Ctrl Pts',(-0.0214982998290823,-0.15406063027223,
-0.142905026755961));
#81551=CARTESIAN_POINT('Ctrl Pts',(-0.0204818549719584,-0.154199054670654,
-0.142832340131764));
#81552=CARTESIAN_POINT('Ctrl Pts',(-0.0162211543859929,-0.15473642265913,
-0.142530078814524));
#81553=CARTESIAN_POINT('Ctrl Pts',(-0.0129658583984935,-0.155043144152888,
-0.142305009129716));
#81554=CARTESIAN_POINT('Ctrl Pts',(-0.00340403136016302,-0.15564076473401,
-0.141654694293588));
#81555=CARTESIAN_POINT('Ctrl Pts',(0.00291356860509002,-0.155650755101249,
-0.141238549804585));
#81556=CARTESIAN_POINT('Ctrl Pts',(0.0195895207723907,-0.15466114369056,
-0.140138000042312));
#81557=CARTESIAN_POINT('Ctrl Pts',(0.0298753262041725,-0.153007359109028,
-0.139455320127346));
#81558=CARTESIAN_POINT('Ctrl Pts',(0.0419928269420551,-0.149789884614514,
-0.138592190486371));
#81559=CARTESIAN_POINT('Ctrl Pts',(0.0440550760486813,-0.149196369140589,
-0.138443260984368));
#81560=CARTESIAN_POINT('Ctrl Pts',(0.0474240356535321,-0.148150844650158,
-0.138196205313304));
#81561=CARTESIAN_POINT('Ctrl Pts',(0.048738209523348,-0.14772372403685,
-0.138098879799304));
#81562=CARTESIAN_POINT('Ctrl Pts',(0.0511116894266629,-0.146917199092269,
-0.137921274174827));
#81563=CARTESIAN_POINT('Ctrl Pts',(0.0521729122818032,-0.146543697538566,
-0.137841192287007));
#81564=CARTESIAN_POINT('Ctrl Pts',(0.0544632509303803,-0.145709572541708,
-0.137666849689987));
#81565=CARTESIAN_POINT('Ctrl Pts',(0.055690766025367,-0.145244840242195,
-0.137572458014198));
#81566=CARTESIAN_POINT('Ctrl Pts',(0.0591372624536412,-0.143889897789063,
-0.137304655600798));
#81567=CARTESIAN_POINT('Ctrl Pts',(0.0613417220724725,-0.142964018066949,
-0.137130073371118));
#81568=CARTESIAN_POINT('Ctrl Pts',(0.0710783574435325,-0.138607947421825,
-0.136343727067144));
#81569=CARTESIAN_POINT('Ctrl Pts',(0.0783499054799438,-0.134631161074682,
-0.135714064036659));
#81570=CARTESIAN_POINT('Ctrl Pts',(0.0931289925420109,-0.124944375660826,
-0.134349826740864));
#81571=CARTESIAN_POINT('Ctrl Pts',(0.100505516059808,-0.119091395922819,
-0.133615163624594));
#81572=CARTESIAN_POINT('Ctrl Pts',(0.10907910426226,-0.110921283305335,
-0.132721328145162));
#81573=CARTESIAN_POINT('Ctrl Pts',(0.110809459217712,-0.109192708096999,
-0.132538696024852));
#81574=CARTESIAN_POINT('Ctrl Pts',(0.113155733713252,-0.106735599745172,
-0.132288742941705));
#81575=CARTESIAN_POINT('Ctrl Pts',(0.113806708964276,-0.106041225199133,
-0.13221913552374));
#81576=CARTESIAN_POINT('Ctrl Pts',(0.11488837918105,-0.104866006860694,
-0.132103102618546));
#81577=CARTESIAN_POINT('Ctrl Pts',(0.115322521650834,-0.10438838599056,
-0.132056428871857));
#81578=CARTESIAN_POINT('Ctrl Pts',(0.116222930309442,-0.103385329676926,
-0.131959434366982));
#81579=CARTESIAN_POINT('Ctrl Pts',(0.11668862935952,-0.102859417420478,
-0.13190915381113));
#81580=CARTESIAN_POINT('Ctrl Pts',(0.117935853602077,-0.101431558885703,
-0.131774124317263));
#81581=CARTESIAN_POINT('Ctrl Pts',(0.118710607275242,-0.100523721833283,
-0.131689848399715));
#81582=CARTESIAN_POINT('Ctrl Pts',(0.123066776400221,-0.0952986612445279,
-0.131213086612784));
#81583=CARTESIAN_POINT('Ctrl Pts',(0.126423459789405,-0.0907986245009861,
-0.130834226990511));
#81584=CARTESIAN_POINT('Ctrl Pts',(0.135994531210639,-0.0764042139687098,
-0.129683017404976));
#81585=CARTESIAN_POINT('Ctrl Pts',(0.141343742329626,-0.0659853346916232,
-0.1289290866551));
#81586=CARTESIAN_POINT('Ctrl Pts',(0.146854097051682,-0.0514277188377062,
-0.127875503560243));
#81587=CARTESIAN_POINT('Ctrl Pts',(0.148094184488826,-0.0477393394530037,
-0.127608875861934));
#81588=CARTESIAN_POINT('Ctrl Pts',(0.149650266975529,-0.0424640243738569,
-0.127225611910502));
#81589=CARTESIAN_POINT('Ctrl Pts',(0.150081846495681,-0.0409125260293477,
-0.127112669171581));
#81590=CARTESIAN_POINT('Ctrl Pts',(0.150778348355001,-0.038249155273976,
-0.126918258672288));
#81591=CARTESIAN_POINT('Ctrl Pts',(0.151055251945639,-0.0371405296906429,
-0.126837180984591));
#81592=CARTESIAN_POINT('Ctrl Pts',(0.151597291910299,-0.0348639890248439,
-0.126670322018178));
#81593=CARTESIAN_POINT('Ctrl Pts',(0.151861203818948,-0.0336958643231532,
-0.126584507704465));
#81594=CARTESIAN_POINT('Ctrl Pts',(0.152495377574027,-0.0307299715899738,
-0.126366066943848));
#81595=CARTESIAN_POINT('Ctrl Pts',(0.152847345822969,-0.028928527061049,
-0.126232872464656));
#81596=CARTESIAN_POINT('Ctrl Pts',(0.154269106263817,-0.0208991588885878,
-0.12563665539049));
#81597=CARTESIAN_POINT('Ctrl Pts',(0.154990552413085,-0.0146164698083195,
-0.125163021815002));
#81598=CARTESIAN_POINT('Ctrl Pts',(0.155668420204074,-0.00194299723188557,
-0.124194568261939));
#81599=CARTESIAN_POINT('Ctrl Pts',(0.155617286804773,0.0044366409719101,
-0.123700498307034));
#81600=CARTESIAN_POINT('Ctrl Pts',(0.154669760544396,0.0180573654061419,
-0.122642587704769));
#81601=CARTESIAN_POINT('Ctrl Pts',(0.153655243252302,0.0252762739670338,
-0.122080011683065));
#81602=CARTESIAN_POINT('Ctrl Pts',(0.151804899131552,0.0339653125853173,
-0.121417491799563));
#81603=CARTESIAN_POINT('Ctrl Pts',(0.15144695827776,0.035527302384748,-0.121299003108598));
#81604=CARTESIAN_POINT('Ctrl Pts',(0.150877432083684,0.0378473448089441,
-0.121124190463759));
#81605=CARTESIAN_POINT('Ctrl Pts',(0.150684142213483,0.03860971869733,-0.121066937926192));
#81606=CARTESIAN_POINT('Ctrl Pts',(0.150324431550832,0.0399846295194425,
-0.120964071606457));
#81607=CARTESIAN_POINT('Ctrl Pts',(0.150160036703584,0.0405976444074333,
-0.120918351041281));
#81608=CARTESIAN_POINT('Ctrl Pts',(0.149777158106643,0.0419912172752532,
-0.120814732313206));
#81609=CARTESIAN_POINT('Ctrl Pts',(0.14955632047996,0.0427710942133087,
-0.120756967878569));
#81610=CARTESIAN_POINT('Ctrl Pts',(0.148844977583074,0.045210273877995,
-0.120576897182742));
#81611=CARTESIAN_POINT('Ctrl Pts',(0.148332857576188,0.0468632075740606,
-0.120455738753383));
#81612=CARTESIAN_POINT('Ctrl Pts',(0.147037498812961,0.0508099353442831,
-0.12016776329997));
#81613=CARTESIAN_POINT('Ctrl Pts',(0.146228010115644,0.0530946888306141,
-0.12000213419497));
#81614=CARTESIAN_POINT('Ctrl Pts',(0.142711754927331,0.0623277904326568,
-0.119333661571723));
#81615=CARTESIAN_POINT('Ctrl Pts',(0.139560330334423,0.0690965093559548,
-0.11884526679557));
#81616=CARTESIAN_POINT('Ctrl Pts',(0.131647368010437,0.0833221715997394,
-0.117772539797679));
#81617=CARTESIAN_POINT('Ctrl Pts',(0.126711976141903,0.0906513281441833,
-0.117188452647073));
#81618=CARTESIAN_POINT('Ctrl Pts',(0.119819814629659,0.0992156170903066,
-0.116431941971945));
#81619=CARTESIAN_POINT('Ctrl Pts',(0.118421847140731,0.100880087168698,
-0.11628113897298));
#81620=CARTESIAN_POINT('Ctrl Pts',(0.116073545200341,0.103559964708645,
-0.116031632949334));
#81621=CARTESIAN_POINT('Ctrl Pts',(0.115143627472956,0.104592920492552,
-0.115933759000465));
#81622=CARTESIAN_POINT('Ctrl Pts',(0.113435886689785,0.106439507297926,
-0.115755580728603));
#81623=CARTESIAN_POINT('Ctrl Pts',(0.112662828363345,0.107257429053053,
-0.115675481011064));
#81624=CARTESIAN_POINT('Ctrl Pts',(0.110973561566323,0.109006316795537,
-0.11550159106784));
#81625=CARTESIAN_POINT('Ctrl Pts',(0.110054372132267,0.109934268773431,
-0.115407675138143));
#81626=CARTESIAN_POINT('Ctrl Pts',(0.10744232692818,0.112505622375854,-0.115142666372704));
#81627=CARTESIAN_POINT('Ctrl Pts',(0.105723674699108,0.114122180874038,
-0.114970440914707));
#81628=CARTESIAN_POINT('Ctrl Pts',(0.103430043567632,0.11618327608146,-0.114743209866952));
#81629=CARTESIAN_POINT('Ctrl Pts',(0.102887773590145,0.11666376178256,-0.114689672288783));
#81630=CARTESIAN_POINT('Ctrl Pts',(0.102342241743611,0.11714037755997,-0.114635995609957));
#81631=CARTESIAN_POINT('Origin',(0.,0.,-1.10400562256037));
#81632=CARTESIAN_POINT('',(0.10234224283772,0.117140376604078,-0.0306875317892119));
#81633=CARTESIAN_POINT('',(0.102472688294207,0.117287771082297,-0.0445113451759945));
#81634=CARTESIAN_POINT('',(0.10234224283772,0.117140376604078,-1.10400562256037));
#81635=CARTESIAN_POINT('',(-0.155549938411928,0.00013841981592947,-0.0751943774352678));
#81636=CARTESIAN_POINT('Ctrl Pts',(-0.155549938411928,0.00013841981592947,
-0.0751943774352684));
#81637=CARTESIAN_POINT('Ctrl Pts',(-0.155558961220896,-0.0100010054528611,
-0.0744674884213844));
#81638=CARTESIAN_POINT('Ctrl Pts',(-0.15457225557722,-0.020170319397278,
-0.0737405994074998));
#81639=CARTESIAN_POINT('Ctrl Pts',(-0.152598751870448,-0.030156648148979,
-0.0730137103936159));
#81640=CARTESIAN_POINT('Ctrl Pts',(-0.150627608514691,-0.0401310330461434,
-0.0722876907539397));
#81641=CARTESIAN_POINT('Ctrl Pts',(-0.147672161675392,-0.0499219254392591,
-0.0715616711142636));
#81642=CARTESIAN_POINT('Ctrl Pts',(-0.143792804224831,-0.0593248004898402,
-0.0708356514745874));
#81643=CARTESIAN_POINT('Ctrl Pts',(-0.139904255190837,-0.0687499543099442,
-0.0701079116350643));
#81644=CARTESIAN_POINT('Ctrl Pts',(-0.135087793914332,-0.0777843672882017,
-0.0693801717955413));
#81645=CARTESIAN_POINT('Ctrl Pts',(-0.129452156882421,-0.0862435016594814,
-0.0686524319560182));
#81646=CARTESIAN_POINT('Ctrl Pts',(-0.123914476917127,-0.0945556017231172,
-0.0679373414868388));
#81647=CARTESIAN_POINT('Ctrl Pts',(-0.117586561399235,-0.102311666098563,
-0.0672222510176595));
#81648=CARTESIAN_POINT('Ctrl Pts',(-0.110609361986205,-0.109368055395553,
-0.0665071605484802));
#81649=CARTESIAN_POINT('Ctrl Pts',(-0.10341070889456,-0.116648411828215,
-0.0657693733774343));
#81650=CARTESIAN_POINT('Ctrl Pts',(-0.0954635778570838,-0.123241902787809,
-0.0650315862063881));
#81651=CARTESIAN_POINT('Ctrl Pts',(-0.0869230970916733,-0.128996812720282,
-0.064293799035342));
#81652=CARTESIAN_POINT('Ctrl Pts',(-0.078365523499258,-0.134763240468041,
-0.0635545352649303));
#81653=CARTESIAN_POINT('Ctrl Pts',(-0.0692129102355039,-0.13968709048397,
-0.0628152714945182));
#81654=CARTESIAN_POINT('Ctrl Pts',(-0.0596549654545681,-0.143656143609016,
-0.0620760077241065));
#81655=CARTESIAN_POINT('Ctrl Pts',(-0.0501377917152772,-0.147608266061835,
-0.0613398974092399));
#81656=CARTESIAN_POINT('Ctrl Pts',(-0.0402195952627188,-0.150613357985868,
-0.0606037870943737));
#81657=CARTESIAN_POINT('Ctrl Pts',(-0.0301093058995079,-0.152608100041413,
-0.0598676767795072));
#81658=CARTESIAN_POINT('Ctrl Pts',(-0.0199340486624365,-0.154615660142574,
-0.0591268362813229));
#81659=CARTESIAN_POINT('Ctrl Pts',(-0.00956514831970885,-0.155599647111316,
-0.0583859957831381));
#81660=CARTESIAN_POINT('Ctrl Pts',(0.000775890449174843,-0.155548064899602,
-0.0576451552849537));
#81661=CARTESIAN_POINT('Ctrl Pts',(0.0111169292180593,-0.155496482687888,
-0.0569043147867693));
#81662=CARTESIAN_POINT('Ctrl Pts',(0.021429166655461,-0.154409464200979,
-0.0561634742885849));
#81663=CARTESIAN_POINT('Ctrl Pts',(0.0314967375605351,-0.152327797932757,
-0.0554226337904005));
#81664=CARTESIAN_POINT('Ctrl Pts',(0.0415054151158392,-0.150258309011066,
-0.0546861270663702));
#81665=CARTESIAN_POINT('Ctrl Pts',(0.0513470946389434,-0.14719032789149,
-0.0539496203423399));
#81666=CARTESIAN_POINT('Ctrl Pts',(0.060810581508614,-0.14317079198141,
-0.0532131136183096));
#81667=CARTESIAN_POINT('Ctrl Pts',(0.0703136072509937,-0.139134462269967,
-0.0524735297361438));
#81668=CARTESIAN_POINT('Ctrl Pts',(0.0794343486427382,-0.134138822528049,
-0.0517339458539783));
#81669=CARTESIAN_POINT('Ctrl Pts',(0.0879745491710003,-0.128282037706607,
-0.0509943619718125));
#81670=CARTESIAN_POINT('Ctrl Pts',(0.0964599027186236,-0.122462866400519,
-0.050259527854331));
#81671=CARTESIAN_POINT('Ctrl Pts',(0.10437138151846,-0.115794117272148,
-0.04952469373685));
#81672=CARTESIAN_POINT('Ctrl Pts',(0.111542561775653,-0.108416140000115,
-0.0487898596193685));
#81673=CARTESIAN_POINT('Ctrl Pts',(0.118783270824285,-0.100966628918502,
-0.0480479008548607));
#81674=CARTESIAN_POINT('Ctrl Pts',(0.125268556296564,-0.0927947320807613,
-0.0473059420903526));
#81675=CARTESIAN_POINT('Ctrl Pts',(0.130867025676167,-0.0840810566695813,
-0.0465639833258447));
#81676=CARTESIAN_POINT('Ctrl Pts',(0.13646549505577,-0.0753673812584019,
-0.0458220245613368));
#81677=CARTESIAN_POINT('Ctrl Pts',(0.141176742647482,-0.0661128063666765,
-0.0450800657968286));
#81678=CARTESIAN_POINT('Ctrl Pts',(0.144917390905267,-0.0565221400268082,
-0.0443381070323208));
#81679=CARTESIAN_POINT('Ctrl Pts',(0.148642969898444,-0.0469701098480734,
-0.0435991372612117));
#81680=CARTESIAN_POINT('Ctrl Pts',(0.151433720977259,-0.03701323759064,
-0.0428601674901025));
#81681=CARTESIAN_POINT('Ctrl Pts',(0.153214174245866,-0.0268555266222315,
-0.0421211977189935));
#81682=CARTESIAN_POINT('Ctrl Pts',(0.154994623537292,-0.0166978383441483,
-0.0413822295985973));
#81683=CARTESIAN_POINT('Ctrl Pts',(0.155764497211888,-0.00634019488119242,
-0.0406432614782013));
#81684=CARTESIAN_POINT('Ctrl Pts',(0.155498581209574,0.00399921764967614,
-0.0399042933578051));
#81685=CARTESIAN_POINT('Ctrl Pts',(0.155233287886262,0.0143144190198078,
-0.0391670556332016));
#81686=CARTESIAN_POINT('Ctrl Pts',(0.153937050533157,0.0246105496841226,
-0.0384298179085981));
#81687=CARTESIAN_POINT('Ctrl Pts',(0.151636941721272,0.0346704543584231,
-0.0376925801839947));
#81688=CARTESIAN_POINT('Ctrl Pts',(0.149328734913697,0.0447657769504627,
-0.0369527468657023));
#81689=CARTESIAN_POINT('Ctrl Pts',(0.146009791770651,0.0546222990557376,
-0.0362129135474098));
#81690=CARTESIAN_POINT('Ctrl Pts',(0.141758457587672,0.0640339144701007,
-0.0354730802291174));
#81691=CARTESIAN_POINT('Ctrl Pts',(0.137507123404693,0.0734455298844644,
-0.034733246910825));
#81692=CARTESIAN_POINT('Ctrl Pts',(0.132323889645745,0.0824114459753015,
-0.0339934135925325));
#81693=CARTESIAN_POINT('Ctrl Pts',(0.126332605879763,0.0907517228025362,
-0.03325358027424));
#81694=CARTESIAN_POINT('Ctrl Pts',(0.120350725319235,0.0990789097245675,
-0.0325149081102118));
#81695=CARTESIAN_POINT('Ctrl Pts',(0.113520461596062,0.106842110718766,
-0.0317762359461835));
#81696=CARTESIAN_POINT('Ctrl Pts',(0.105972061558888,0.113867136035642,
-0.0310375637821552));
#81697=CARTESIAN_POINT('Ctrl Pts',(0.104779750257061,0.114976777421853,
-0.030920886451174));
#81698=CARTESIAN_POINT('Ctrl Pts',(0.103569608066442,0.116068062224272,
-0.030804209120193));
#81699=CARTESIAN_POINT('Ctrl Pts',(0.10234224283772,0.117140376604078,-0.0306875317892119));
#81700=CARTESIAN_POINT('Ctrl Pts',(0.10234224283772,0.117140376604078,-0.100698721018058));
#81701=CARTESIAN_POINT('Ctrl Pts',(0.099065544252337,0.120003135731656,
-0.100386060952946));
#81702=CARTESIAN_POINT('Ctrl Pts',(0.0956728992865777,0.122724582357694,
-0.100073400887833));
#81703=CARTESIAN_POINT('Ctrl Pts',(0.0921780765868749,0.125295669106096,
-0.099760740822721));
#81704=CARTESIAN_POINT('Ctrl Pts',(0.083933296768488,0.131361225489355,
-0.0990231316172315));
#81705=CARTESIAN_POINT('Ctrl Pts',(0.075056647698021,0.13663202138511,-0.0982855224117419));
#81706=CARTESIAN_POINT('Ctrl Pts',(0.0657249117760847,0.140982404831333,
-0.0975479132062524));
#81707=CARTESIAN_POINT('Ctrl Pts',(0.0563716805356272,0.145342809229569,
-0.0968086049444514));
#81708=CARTESIAN_POINT('Ctrl Pts',(0.0465620415849983,0.148778030941094,
-0.0960692966826506));
#81709=CARTESIAN_POINT('Ctrl Pts',(0.0365009764596717,0.151206749907173,
-0.0953299884208496));
#81710=CARTESIAN_POINT('Ctrl Pts',(0.0264859355025571,0.153624358740395,
-0.0945940621118913));
#81711=CARTESIAN_POINT('Ctrl Pts',(0.0162226691210491,0.15504443073102,
-0.093858135802933));
#81712=CARTESIAN_POINT('Ctrl Pts',(0.00592733703515371,0.155437026398705,
-0.0931222094939748));
#81713=CARTESIAN_POINT('Ctrl Pts',(-0.00443896342187721,0.155832328329269,
-0.0923812102557524));
#81714=CARTESIAN_POINT('Ctrl Pts',(-0.0148368252824632,0.155185885906542,
-0.0916402110175299));
#81715=CARTESIAN_POINT('Ctrl Pts',(-0.0250453720823497,0.153520460646966,
-0.0908992117793075));
#81716=CARTESIAN_POINT('Ctrl Pts',(-0.0352539188822363,0.15185503538739,
-0.0901582125410851));
#81717=CARTESIAN_POINT('Ctrl Pts',(-0.0452722405618459,0.14917090625426,
-0.0894172133028628));
#81718=CARTESIAN_POINT('Ctrl Pts',(-0.0548933067350833,0.145542184179323,
-0.0886762140646404));
#81719=CARTESIAN_POINT('Ctrl Pts',(-0.0644677683058369,0.141931039693687,
-0.0879388042388923));
#81720=CARTESIAN_POINT('Ctrl Pts',(-0.0737200321747962,0.137357610691785,
-0.0872013944131441));
#81721=CARTESIAN_POINT('Ctrl Pts',(-0.0824485118212944,0.13190165047661,
-0.086463984587396));
#81722=CARTESIAN_POINT('Ctrl Pts',(-0.091200052634537,0.126431275287309,
-0.0857246264806598));
#81723=CARTESIAN_POINT('Ctrl Pts',(-0.0994241707757214,0.120074063795145,
-0.0849852683739235));
#81724=CARTESIAN_POINT('Ctrl Pts',(-0.106940916035916,0.112957704373802,
-0.0842459102671873));
#81725=CARTESIAN_POINT('Ctrl Pts',(-0.114420758447958,0.105876282138971,
-0.0835101819788097));
#81726=CARTESIAN_POINT('Ctrl Pts',(-0.121199478655776,0.0980437895257948,
-0.0827744536904321));
#81727=CARTESIAN_POINT('Ctrl Pts',(-0.127134317940192,0.0896251510563975,
-0.0820387254020545));
#81728=CARTESIAN_POINT('Ctrl Pts',(-0.133113077763476,0.081144210792396,
-0.0812975523861389));
#81729=CARTESIAN_POINT('Ctrl Pts',(-0.138234853997668,0.0720691822704437,
-0.0805563793702231));
#81730=CARTESIAN_POINT('Ctrl Pts',(-0.142398385512891,0.0625979416859848,
-0.0798152063543074));
#81731=CARTESIAN_POINT('Ctrl Pts',(-0.146561917028115,0.0531267011015265,
-0.0790740333383918));
#81732=CARTESIAN_POINT('Ctrl Pts',(-0.149766941868116,0.0432601666174164,
-0.0783328603224763));
#81733=CARTESIAN_POINT('Ctrl Pts',(-0.151962914424122,0.0332125750240309,
-0.0775916873065607));
#81734=CARTESIAN_POINT('Ctrl Pts',(-0.154330524758453,0.0223796610941352,
-0.0767925840175835));
#81735=CARTESIAN_POINT('Ctrl Pts',(-0.155540019209143,0.0112851670771924,
-0.0759934807286063));
#81736=CARTESIAN_POINT('Ctrl Pts',(-0.155549938411874,0.000138419876762847,
-0.0751943774396291));
#81737=CARTESIAN_POINT('',(-0.155733678035791,-9.10003121109568E-5,-0.0890056225603696));
#81738=CARTESIAN_POINT('Ctrl Pts',(0.102342241743611,0.11714037755997,-0.114635995609957));
#81739=CARTESIAN_POINT('Ctrl Pts',(0.0968453600151427,0.121942847983995,
-0.11409513927507));
#81740=CARTESIAN_POINT('Ctrl Pts',(0.0910173447333404,0.126352381427472,
-0.11353950234708));
#81741=CARTESIAN_POINT('Ctrl Pts',(0.0774511378432751,0.135189422552379,
-0.112290605212437));
#81742=CARTESIAN_POINT('Ctrl Pts',(0.069598565891125,0.1393947807694,-0.111595784377499));
#81743=CARTESIAN_POINT('Ctrl Pts',(0.0586039155637544,0.144120933261064,
-0.110686783442491));
#81744=CARTESIAN_POINT('Ctrl Pts',(0.0557425926729581,0.145251605108168,
-0.11045580441431));
#81745=CARTESIAN_POINT('Ctrl Pts',(0.0518767736557376,0.146648124126632,
-0.11015273675136));
#81746=CARTESIAN_POINT('Ctrl Pts',(0.050900632440027,0.146989787829005,
-0.110076964342815));
#81747=CARTESIAN_POINT('Ctrl Pts',(0.0493510049672212,0.147514891328427,
-0.109957942021176));
#81748=CARTESIAN_POINT('Ctrl Pts',(0.0487797585361175,0.147704773264564,
-0.109914336590083));
#81749=CARTESIAN_POINT('Ctrl Pts',(0.047576719236147,0.148096922060416,
-0.109823091959806));
#81750=CARTESIAN_POINT('Ctrl Pts',(0.0469447086619598,0.148298472330081,
-0.109775497880124));
#81751=CARTESIAN_POINT('Ctrl Pts',(0.0453462199241087,0.148796992758305,
-0.109655935606263));
#81752=CARTESIAN_POINT('Ctrl Pts',(0.0443780774605145,0.149088601506892,
-0.109584267986357));
#81753=CARTESIAN_POINT('Ctrl Pts',(0.0404005469651865,0.150244471444413,
-0.109292611450648));
#81754=CARTESIAN_POINT('Ctrl Pts',(0.0373680168798433,0.151027282277312,
-0.109076741194422));
#81755=CARTESIAN_POINT('Ctrl Pts',(0.0286006284475955,0.153010179488705,
-0.108465651796799));
#81756=CARTESIAN_POINT('Ctrl Pts',(0.0228187282802862,0.15397865608585,
-0.108078290504308));
#81757=CARTESIAN_POINT('Ctrl Pts',(0.0059827903349026,0.15582925368744,
-0.106961695665347));
#81758=CARTESIAN_POINT('Ctrl Pts',(-0.00512656899842589,0.155859665710325,
-0.106236465954617));
#81759=CARTESIAN_POINT('Ctrl Pts',(-0.0184488146127189,0.154469452875764,
-0.105313868514814));
#81760=CARTESIAN_POINT('Ctrl Pts',(-0.0207474547415164,0.15417753660979,
-0.105152877653028));
#81761=CARTESIAN_POINT('Ctrl Pts',(-0.0243351354556274,0.153640236716811,
-0.104898308155404));
#81762=CARTESIAN_POINT('Ctrl Pts',(-0.0256291087018177,0.153429689944544,
-0.104805817141266));
#81763=CARTESIAN_POINT('Ctrl Pts',(-0.0280284508453781,0.153008086431379,
-0.104632980169495));
#81764=CARTESIAN_POINT('Ctrl Pts',(-0.0291344970364497,0.152801340083493,
-0.104552775240655));
#81765=CARTESIAN_POINT('Ctrl Pts',(-0.0315957180653166,0.15231358572355,
-0.104373064867778));
#81766=CARTESIAN_POINT('Ctrl Pts',(-0.0329495663908012,0.152026457046933,
-0.104273371318934));
#81767=CARTESIAN_POINT('Ctrl Pts',(-0.0369874899900583,0.151113610919677,
-0.103973416108908));
#81768=CARTESIAN_POINT('Ctrl Pts',(-0.0396588227989189,0.150434616424488,
-0.103771491193925));
#81769=CARTESIAN_POINT('Ctrl Pts',(-0.050852546957745,0.147270554916142,
-0.102910022147505));
#81770=CARTESIAN_POINT('Ctrl Pts',(-0.0591709003089992,0.144129657031934,
-0.102230545409286));
#81771=CARTESIAN_POINT('Ctrl Pts',(-0.0758443782874427,0.136146330023963,
-0.100799703513772));
#81772=CARTESIAN_POINT('Ctrl Pts',(-0.0841110990631629,0.131200403202779,
-0.100050059253136));
#81773=CARTESIAN_POINT('Ctrl Pts',(-0.093070702087738,0.124642950555568,
-0.099223382073601));
#81774=CARTESIAN_POINT('Ctrl Pts',(-0.0942599236657631,0.123746062276734,
-0.099113375727178));
#81775=CARTESIAN_POINT('Ctrl Pts',(-0.0960471084537074,0.122357484813098,
-0.0989478456297389));
#81776=CARTESIAN_POINT('Ctrl Pts',(-0.0966545488592804,0.121878215383102,
-0.0988915464626218));
#81777=CARTESIAN_POINT('Ctrl Pts',(-0.0977045129919885,0.121037008375313,
-0.0987942034440611));
#81778=CARTESIAN_POINT('Ctrl Pts',(-0.0981486413247851,0.12067714567441,
-0.0987530212801998));
#81779=CARTESIAN_POINT('Ctrl Pts',(-0.0986020514402913,0.120305603208518,
-0.0987109690894652));
#81780=CARTESIAN_POINT('Ctrl Pts',(-0.0986133015423969,0.120296381784774,
-0.098709925674646));
#81781=CARTESIAN_POINT('Ctrl Pts',(-0.0986343142312683,0.120279153287461,
-0.0987079767934577));
#81782=CARTESIAN_POINT('Ctrl Pts',(-0.0986440771352481,0.120271146604481,
-0.0987070712995619));
#81783=CARTESIAN_POINT('Ctrl Pts',(-0.0986623573757319,0.12025615102128,
-0.0987053758251081));
#81784=CARTESIAN_POINT('Ctrl Pts',(-0.0986708749438864,0.12024916240539,
-0.0987045858244758));
#81785=CARTESIAN_POINT('Ctrl Pts',(-0.0986868575231541,0.12023604594913,
-0.0987031034387955));
#81786=CARTESIAN_POINT('Ctrl Pts',(-0.0986943227053451,0.120229918319069,
-0.0987024110389428));
#81787=CARTESIAN_POINT('Ctrl Pts',(-0.0987083565367617,0.120218396770432,
-0.0987011093864393));
#81788=CARTESIAN_POINT('Ctrl Pts',(-0.0987149253142471,0.12021300300901,
-0.0987005001227003));
#81789=CARTESIAN_POINT('Ctrl Pts',(-0.0987272939401283,0.120202845172625,
-0.098699352909224));
#81790=CARTESIAN_POINT('Ctrl Pts',(-0.0987330938853791,0.120198081216613,
-0.0986988149511227));
#81791=CARTESIAN_POINT('Ctrl Pts',(-0.0987504054580136,0.120183859747638,
-0.0986972092567941));
#81792=CARTESIAN_POINT('Ctrl Pts',(-0.0987619160762045,0.120174400996715,
-0.098696141607642));
#81793=CARTESIAN_POINT('Ctrl Pts',(-0.0987846854587873,0.120155684972726,
-0.0986940296519114));
#81794=CARTESIAN_POINT('Ctrl Pts',(-0.098795944280803,0.120146427770956,
-0.0986929853403719));
#81795=CARTESIAN_POINT('Ctrl Pts',(-0.0988182315009227,0.120128097574941,
-0.0986909180728842));
#81796=CARTESIAN_POINT('Ctrl Pts',(-0.0988292599509602,0.120119024644269,
-0.0986898951124704));
#81797=CARTESIAN_POINT('Ctrl Pts',(-0.09885110625777,0.120101046989337,
-0.0986878687084864));
#81798=CARTESIAN_POINT('Ctrl Pts',(-0.0988619241610093,0.120092142322065,
-0.0986868652609278));
#81799=CARTESIAN_POINT('Ctrl Pts',(-0.0988833677845966,0.120074486320233,
-0.0986848761755496));
#81800=CARTESIAN_POINT('Ctrl Pts',(-0.0988939935463891,0.120065735036849,
-0.0986838905341799));
#81801=CARTESIAN_POINT('Ctrl Pts',(-0.0989150700336364,0.120048371932408,
-0.0986819354712143));
#81802=CARTESIAN_POINT('Ctrl Pts',(-0.0989255207964517,0.120039760156925,
-0.0986809660464215));
#81803=CARTESIAN_POINT('Ctrl Pts',(-0.0989462633091198,0.120022663089445,
-0.0986790419307446));
#81804=CARTESIAN_POINT('Ctrl Pts',(-0.0989565550921221,0.120014177838372,
-0.0986780872370303));
#81805=CARTESIAN_POINT('Ctrl Pts',(-0.0989769946672544,0.119997321635479,
-0.0986761911904458));
#81806=CARTESIAN_POINT('Ctrl Pts',(-0.098987142488969,0.119988950720136,
-0.0986752498350535));
#81807=CARTESIAN_POINT('Ctrl Pts',(-0.0990073082722792,0.119972311711489,
-0.0986733791546542));
#81808=CARTESIAN_POINT('Ctrl Pts',(-0.0990173262601682,0.119964043650623,
-0.0986724498274095));
#81809=CARTESIAN_POINT('Ctrl Pts',(-0.0990372457123638,0.119947599503267,
-0.0986706019664489));
#81810=CARTESIAN_POINT('Ctrl Pts',(-0.0990471472001404,0.119939423445343,
-0.0986696834307372));
#81811=CARTESIAN_POINT('Ctrl Pts',(-0.0990668462827558,0.119923153015172,
-0.0986678559813986));
#81812=CARTESIAN_POINT('Ctrl Pts',(-0.0990766438981405,0.119915058668179,
-0.0986669470660283));
#81813=CARTESIAN_POINT('Ctrl Pts',(-0.0990961472383411,0.119898941868049,
-0.0986651377441451));
#81814=CARTESIAN_POINT('Ctrl Pts',(-0.0991058529812392,0.119890919436886,
-0.0986642373360991));
#81815=CARTESIAN_POINT('Ctrl Pts',(-0.0991251840221976,0.119874937116027,
-0.0986624439672103));
#81816=CARTESIAN_POINT('Ctrl Pts',(-0.0991348093358464,0.11986697724541,
-0.0986615510050484));
#81817=CARTESIAN_POINT('Ctrl Pts',(-0.0991539904710281,0.119851111081601,
-0.0986597715119472));
#81818=CARTESIAN_POINT('Ctrl Pts',(-0.0991635463059423,0.119843204804664,
-0.0986588849798768));
#81819=CARTESIAN_POINT('Ctrl Pts',(-0.099182599002665,0.119827437204787,
-0.0986571173711519));
#81820=CARTESIAN_POINT('Ctrl Pts',(-0.0991920958754488,0.119819575895705,
-0.0986562362935733));
#81821=CARTESIAN_POINT('Ctrl Pts',(-0.0992110407855756,0.119803889906521,
-0.0986544786533435));
#81822=CARTESIAN_POINT('Ctrl Pts',(-0.0992204888319279,0.119796065237738,
-0.0986536020899347));
#81823=CARTESIAN_POINT('Ctrl Pts',(-0.0992393458956281,0.11978044446201,
-0.0986518525682251));
#81824=CARTESIAN_POINT('Ctrl Pts',(-0.0992487549198683,0.119772648364161,
-0.0986509796093476));
#81825=CARTESIAN_POINT('Ctrl Pts',(-0.0992675434581723,0.119757076885717,
-0.0986492364135049));
#81826=CARTESIAN_POINT('Ctrl Pts',(-0.0992769229777406,0.119749301511548,
-0.0986483661760762));
#81827=CARTESIAN_POINT('Ctrl Pts',(-0.0999553900851921,0.119186735686285,
-0.0985854170076944));
#81828=CARTESIAN_POINT('Ctrl Pts',(-0.100619837119209,0.118626331143525,
-0.0985237274904377));
#81829=CARTESIAN_POINT('Ctrl Pts',(-0.102105530527473,0.11735181038016,
-0.0983856043935393));
#81830=CARTESIAN_POINT('Ctrl Pts',(-0.102924058891223,0.116634579030526,
-0.098309376209202));
#81831=CARTESIAN_POINT('Ctrl Pts',(-0.105258513591226,0.114545309526885,
-0.0980913603341662));
#81832=CARTESIAN_POINT('Ctrl Pts',(-0.106755056684746,0.113151850869635,
-0.0979508393857119));
#81833=CARTESIAN_POINT('Ctrl Pts',(-0.112148857126832,0.107927278532898,
-0.0974395989850106));
#81834=CARTESIAN_POINT('Ctrl Pts',(-0.115871171224845,0.103920854332224,
-0.0970772306831424));
#81835=CARTESIAN_POINT('Ctrl Pts',(-0.12690615788372,0.0907117062908546,
-0.0959414475563277));
#81836=CARTESIAN_POINT('Ctrl Pts',(-0.133391034276816,0.0808738828897926,
-0.0951750182441215));
#81837=CARTESIAN_POINT('Ctrl Pts',(-0.139726588698447,0.0683912260705418,
-0.0942099975423691));
#81838=CARTESIAN_POINT('Ctrl Pts',(-0.140702539902558,0.0663601821256566,
-0.0940533298573491));
#81839=CARTESIAN_POINT('Ctrl Pts',(-0.142170248052984,0.0631276921755986,
-0.0938041055498973));
#81840=CARTESIAN_POINT('Ctrl Pts',(-0.142691694226751,0.0619400126611123,
-0.093712561729332));
#81841=CARTESIAN_POINT('Ctrl Pts',(-0.143637953927149,0.05970936804908,
-0.0935406000739668));
#81842=CARTESIAN_POINT('Ctrl Pts',(-0.144066415149209,0.058668035126323,
-0.093460311893836));
#81843=CARTESIAN_POINT('Ctrl Pts',(-0.145002677541301,0.0563204231500957,
-0.0932792333460877));
#81844=CARTESIAN_POINT('Ctrl Pts',(-0.145504199860699,0.0550117636832779,
-0.0931782408994444));
#81845=CARTESIAN_POINT('Ctrl Pts',(-0.146972063398045,0.0510209967130532,
-0.092870009362029));
#81846=CARTESIAN_POINT('Ctrl Pts',(-0.147882367790324,0.0483190734494026,
-0.0926609661109985));
#81847=CARTESIAN_POINT('Ctrl Pts',(-0.150977206614264,0.0382243320342762,
-0.0918781477971599));
#81848=CARTESIAN_POINT('Ctrl Pts',(-0.152685338588339,0.0306981094270853,
-0.0912902640206059));
#81849=CARTESIAN_POINT('Ctrl Pts',(-0.154978712495817,0.0154109329596322,
-0.0900962633168567));
#81850=CARTESIAN_POINT('Ctrl Pts',(-0.155554107791177,0.00766935171596105,
-0.0894917598193654));
#81851=CARTESIAN_POINT('Ctrl Pts',(-0.155549977927097,-8.28666372969583E-5,
-0.0889002981283004));
#81852=CARTESIAN_POINT('Ctrl Pts',(-0.155733678035791,-9.10003121109568E-5,
-0.0890056225603696));
#81853=CARTESIAN_POINT('Ctrl Pts',(-0.155771337450929,-0.00550761823091695,
-0.0886163681581111));
#81854=CARTESIAN_POINT('Ctrl Pts',(-0.153061777043569,-0.062301176855948,
-0.0845322715031591));
#81855=CARTESIAN_POINT('Ctrl Pts',(-0.0833593216436694,-0.163684077812068,
-0.0767533325955136));
#81856=CARTESIAN_POINT('Ctrl Pts',(0.0918939642601181,-0.159053435166454,
-0.0656688058374342));
#81857=CARTESIAN_POINT('Ctrl Pts',(0.180657312075961,-0.0140801128612938,
-0.0549214766975938));
#81858=CARTESIAN_POINT('Ctrl Pts',(0.137438874464206,0.0863139887816716,
-0.0478689898104475));
#81859=CARTESIAN_POINT('Ctrl Pts',(0.102472688294207,0.117287771082297,
-0.0445113451759945));
#81860=CARTESIAN_POINT('Origin',(0.,0.,-0.485));
#81861=CARTESIAN_POINT('',(-0.1956163961968,0.000134331411914747,-0.952013030787577));
#81862=CARTESIAN_POINT('',(0.0863231127633264,0.175648025443413,-0.974597867473044));
#81863=CARTESIAN_POINT('Ctrl Pts',(-0.1956163961968,0.000134331411914747,
-0.952013030787577));
#81864=CARTESIAN_POINT('Ctrl Pts',(-0.19566971989317,0.00745513469970677,
-0.952431787590014));
#81865=CARTESIAN_POINT('Ctrl Pts',(-0.191981342224257,0.0793125058488746,
-0.956545386645138));
#81866=CARTESIAN_POINT('Ctrl Pts',(-0.106281980654299,0.201804323958761,
-0.964073665540303));
#81867=CARTESIAN_POINT('Ctrl Pts',(0.03262926834607,0.201667302277058,-0.971183187633017));
#81868=CARTESIAN_POINT('Ctrl Pts',(0.0863231127633264,0.175648025443413,
-0.974597867473044));
#81869=CARTESIAN_POINT('',(-0.0861525859670517,0.175382131162755,-0.9746));
#81870=CARTESIAN_POINT('Origin',(0.,0.,-0.9746));
#81871=CARTESIAN_POINT('',(-0.195414161199284,0.000207025558219241,-0.962186969212424));
#81872=CARTESIAN_POINT('Ctrl Pts',(-0.0861525859670515,0.175382131162755,
-0.9746));
#81873=CARTESIAN_POINT('Ctrl Pts',(-0.144317765490378,0.146809775496019,
-0.970905157747306));
#81874=CARTESIAN_POINT('Ctrl Pts',(-0.191736685832022,0.0801530562864324,
-0.966767480818114));
#81875=CARTESIAN_POINT('Ctrl Pts',(-0.195639513638137,0.00794474237382261,
-0.962629803888923));
#81876=CARTESIAN_POINT('Ctrl Pts',(-0.195579810854541,0.000207201050681732,
-0.962186969212424));
#81877=CARTESIAN_POINT('',(-0.1953805473626,6.85612951323299E-5,-0.892186972544719));
#81878=CARTESIAN_POINT('Ctrl Pts',(-0.19539989034459,0.00020701043939857,
-0.962186969212424));
#81879=CARTESIAN_POINT('Ctrl Pts',(-0.195412469673056,-0.0116667839925565,
-0.961506776602131));
#81880=CARTESIAN_POINT('Ctrl Pts',(-0.194338478881212,-0.023590350489055,
-0.960826583991837));
#81881=CARTESIAN_POINT('Ctrl Pts',(-0.192177141769211,-0.0353426962952271,
-0.960146391381544));
#81882=CARTESIAN_POINT('Ctrl Pts',(-0.190018078336246,-0.0470826788924694,
-0.959466914318895));
#81883=CARTESIAN_POINT('Ctrl Pts',(-0.186774007411375,-0.0586508853449791,
-0.958787437256246));
#81884=CARTESIAN_POINT('Ctrl Pts',(-0.182496005115271,-0.0698309968206588,
-0.958107960193597));
#81885=CARTESIAN_POINT('Ctrl Pts',(-0.178221276950605,-0.081002551696338,
-0.957429003162742));
#81886=CARTESIAN_POINT('Ctrl Pts',(-0.172914506347834,-0.0917857398504531,
-0.956750046131888));
#81887=CARTESIAN_POINT('Ctrl Pts',(-0.1666757469373,-0.101982132664959,
-0.956071089101033));
#81888=CARTESIAN_POINT('Ctrl Pts',(-0.160422453067151,-0.112202280051459,
-0.95539055030161));
#81889=CARTESIAN_POINT('Ctrl Pts',(-0.153233342828904,-0.121832131556134,
-0.954710011502186));
#81890=CARTESIAN_POINT('Ctrl Pts',(-0.145252308775906,-0.130701670973515,
-0.954029472702763));
#81891=CARTESIAN_POINT('Ctrl Pts',(-0.139003391399146,-0.137646262190778,
-0.953496630629789));
#81892=CARTESIAN_POINT('Ctrl Pts',(-0.132269980151298,-0.14412527246669,
-0.952963788556815));
#81893=CARTESIAN_POINT('Ctrl Pts',(-0.125135862889114,-0.150073901192035,
-0.952430946483841));
#81894=CARTESIAN_POINT('Ctrl Pts',(-0.115793508275601,-0.157863820669655,
-0.951733172755742));
#81895=CARTESIAN_POINT('Ctrl Pts',(-0.105688809723304,-0.164804873099924,
-0.951035399027644));
#81896=CARTESIAN_POINT('Ctrl Pts',(-0.0950001891611107,-0.170751644382574,
-0.950337625299546));
#81897=CARTESIAN_POINT('Ctrl Pts',(-0.0843338282669652,-0.17668603117146,
-0.949641304725432));
#81898=CARTESIAN_POINT('Ctrl Pts',(-0.0730866783110694,-0.181629763867164,
-0.948944984151319));
#81899=CARTESIAN_POINT('Ctrl Pts',(-0.0614658534741819,-0.185480750636529,
-0.948248663577205));
#81900=CARTESIAN_POINT('Ctrl Pts',(-0.0498469122605606,-0.189331113198201,
-0.947552455869919));
#81901=CARTESIAN_POINT('Ctrl Pts',(-0.0378552285880504,-0.192088765254431,
-0.946856248162633));
#81902=CARTESIAN_POINT('Ctrl Pts',(-0.0257162504914437,-0.193700372897579,
-0.946160040455347));
#81903=CARTESIAN_POINT('Ctrl Pts',(-0.0135780569622602,-0.195311876379171,
-0.945463877745414));
#81904=CARTESIAN_POINT('Ctrl Pts',(-0.00129345549938047,-0.195777393556016,
-0.944767715035481));
#81905=CARTESIAN_POINT('Ctrl Pts',(0.0109063693168893,-0.195095389766964,
-0.944071552325549));
#81906=CARTESIAN_POINT('Ctrl Pts',(0.0231334414868171,-0.19441186277584,
-0.943373834790703));
#81907=CARTESIAN_POINT('Ctrl Pts',(0.0352744927484605,-0.192575810342531,
-0.942676117255857));
#81908=CARTESIAN_POINT('Ctrl Pts',(0.0471040609448881,-0.189637463183044,
-0.941978399721011));
#81909=CARTESIAN_POINT('Ctrl Pts',(0.0506757309876744,-0.188750295845185,
-0.941767739722594));
#81910=CARTESIAN_POINT('Ctrl Pts',(0.0542191050569545,-0.187762990553711,
-0.941557079724177));
#81911=CARTESIAN_POINT('Ctrl Pts',(0.0577282871149016,-0.186677810322436,
-0.941346419725759));
#81912=CARTESIAN_POINT('Ctrl Pts',(0.0693538915815736,-0.183082705840671,
-0.940648522102294));
#81913=CARTESIAN_POINT('Ctrl Pts',(0.0806815561660394,-0.17838535157395,
-0.939950624478829));
#81914=CARTESIAN_POINT('Ctrl Pts',(0.0914921904373815,-0.172656708786453,
-0.939252726855364));
#81915=CARTESIAN_POINT('Ctrl Pts',(0.102280936127439,-0.16693966493572,
-0.938556242283943));
#81916=CARTESIAN_POINT('Ctrl Pts',(0.112553933870211,-0.160195819692752,
-0.937859757712523));
#81917=CARTESIAN_POINT('Ctrl Pts',(0.122112927822495,-0.152543740804459,
-0.937163273141102));
#81918=CARTESIAN_POINT('Ctrl Pts',(0.131671149266465,-0.144892280317496,
-0.936466844855952));
#81919=CARTESIAN_POINT('Ctrl Pts',(0.140514775110156,-0.136333242083167,
-0.935770416570802));
#81920=CARTESIAN_POINT('Ctrl Pts',(0.148476551225366,-0.127027059070976,
-0.935073988285653));
#81921=CARTESIAN_POINT('Ctrl Pts',(0.156438191522455,-0.117721034810836,
-0.934377571880714));
#81922=CARTESIAN_POINT('Ctrl Pts',(0.163517466935723,-0.107668571558001,
-0.933681155475775));
#81923=CARTESIAN_POINT('Ctrl Pts',(0.169587527661876,-0.0970630231423506,
-0.932984739070836));
#81924=CARTESIAN_POINT('Ctrl Pts',(0.175671530092538,-0.0864331159222585,
-0.932286723137957));
#81925=CARTESIAN_POINT('Ctrl Pts',(0.180741314795697,-0.0752483757505814,
-0.931588707205077));
#81926=CARTESIAN_POINT('Ctrl Pts',(0.184716614286542,-0.0637254455183864,
-0.930890691272198));
#81927=CARTESIAN_POINT('Ctrl Pts',(0.18591031272142,-0.0602653530611877,
-0.930681091837359));
#81928=CARTESIAN_POINT('Ctrl Pts',(0.187005666383098,-0.0567748710197401,
-0.930471492402519));
#81929=CARTESIAN_POINT('Ctrl Pts',(0.188001393688077,-0.0532600785893206,
-0.93026189296768));
#81930=CARTESIAN_POINT('Ctrl Pts',(0.191306541060573,-0.0415933231351084,
-0.929566163305681));
#81931=CARTESIAN_POINT('Ctrl Pts',(0.19353343416577,-0.0295756893586034,
-0.928870433643683));
#81932=CARTESIAN_POINT('Ctrl Pts',(0.194621241094103,-0.0174279234273898,
-0.928174703981684));
#81933=CARTESIAN_POINT('Ctrl Pts',(0.195706742013875,-0.00530590917279384,
-0.927480449175669));
#81934=CARTESIAN_POINT('Ctrl Pts',(0.195657796133363,0.00694483124659212,
-0.926786194369654));
#81935=CARTESIAN_POINT('Ctrl Pts',(0.194464779426019,0.019094752231698,
-0.926091939563638));
#81936=CARTESIAN_POINT('Ctrl Pts',(0.193271955408107,0.0312427108290403,
-0.925397796889804));
#81937=CARTESIAN_POINT('Ctrl Pts',(0.190935466520171,0.0432890056340155,
-0.924703654215969));
#81938=CARTESIAN_POINT('Ctrl Pts',(0.187497697320824,0.0550070313631696,
-0.924009511542135));
#81939=CARTESIAN_POINT('Ctrl Pts',(0.184060158236639,0.0667242727187282,
-0.923315415332372));
#81940=CARTESIAN_POINT('Ctrl Pts',(0.179521757891869,0.0781124538651824,
-0.922621319122609));
#81941=CARTESIAN_POINT('Ctrl Pts',(0.173974552805762,0.0889607496373264,
-0.921927222912846));
#81942=CARTESIAN_POINT('Ctrl Pts',(0.168414633078311,0.099833910578108,
-0.921231535778603));
#81943=CARTESIAN_POINT('Ctrl Pts',(0.161841750388756,0.110163964756701,
-0.92053584864436));
#81944=CARTESIAN_POINT('Ctrl Pts',(0.154392924816104,0.11976637577688,-0.919840161510117));
#81945=CARTESIAN_POINT('Ctrl Pts',(0.152027375543106,0.122815846621144,
-0.919619229743278));
#81946=CARTESIAN_POINT('Ctrl Pts',(0.14957378835313,0.125792186122078,-0.919398297976439));
#81947=CARTESIAN_POINT('Ctrl Pts',(0.147037348322021,0.128690241271157,
-0.9191773662096));
#81948=CARTESIAN_POINT('Ctrl Pts',(0.13903647670072,0.137831780954669,-0.918480465560712));
#81949=CARTESIAN_POINT('Ctrl Pts',(0.130151875512212,0.146256274009908,
-0.917783564911824));
#81950=CARTESIAN_POINT('Ctrl Pts',(0.120536523779986,0.153792413450849,
-0.917086664262936));
#81951=CARTESIAN_POINT('Ctrl Pts',(0.110941208816254,0.161312848850427,
-0.916391215837259));
#81952=CARTESIAN_POINT('Ctrl Pts',(0.100618801895239,0.167948013162257,
-0.915695767411581));
#81953=CARTESIAN_POINT('Ctrl Pts',(0.0897574317888426,0.173564868100291,
-0.915000318985904));
#81954=CARTESIAN_POINT('Ctrl Pts',(0.0788975818574243,0.179180936894196,
-0.914304967896316));
#81955=CARTESIAN_POINT('Ctrl Pts',(0.0674996732154317,0.183778538112216,
-0.913609616806729));
#81956=CARTESIAN_POINT('Ctrl Pts',(0.0557775892654056,0.187269913589289,
-0.912914265717141));
#81957=CARTESIAN_POINT('Ctrl Pts',(0.0440561228898835,0.190761105124284,
-0.912218951261919));
#81958=CARTESIAN_POINT('Ctrl Pts',(0.0320113607683633,0.19314596284133,
-0.911523636806696));
#81959=CARTESIAN_POINT('Ctrl Pts',(0.0198709322294458,0.194387000728785,
-0.910828322351473));
#81960=CARTESIAN_POINT('Ctrl Pts',(0.00770286041451154,0.195630864410467,
-0.910131424692714));
#81961=CARTESIAN_POINT('Ctrl Pts',(-0.00456043690471319,0.195725684784602,
-0.909434527033955));
#81962=CARTESIAN_POINT('Ctrl Pts',(-0.0166889294022454,0.194686002669444,
-0.908737629375195));
#81963=CARTESIAN_POINT('Ctrl Pts',(-0.0204294737291825,0.194365354654989,
-0.908522699400637));
#81964=CARTESIAN_POINT('Ctrl Pts',(-0.0241572412903161,0.193937169211189,
-0.908307769426078));
#81965=CARTESIAN_POINT('Ctrl Pts',(-0.0278656665062796,0.193402855796291,
-0.90809283945152));
#81966=CARTESIAN_POINT('Ctrl Pts',(-0.039888809400841,0.191670549988924,
-0.907396011648354));
#81967=CARTESIAN_POINT('Ctrl Pts',(-0.0517917869311965,0.188806759265524,
-0.906699183845189));
#81968=CARTESIAN_POINT('Ctrl Pts',(-0.0633476521767701,0.184846517315558,
-0.906002356042024));
#81969=CARTESIAN_POINT('Ctrl Pts',(-0.0748794964147279,0.180894507462455,
-0.905306976724594));
#81970=CARTESIAN_POINT('Ctrl Pts',(-0.086064817578607,0.175850781673614,
-0.904611597407164));
#81971=CARTESIAN_POINT('Ctrl Pts',(-0.0966896311347117,0.169800692669475,
-0.903916218089734));
#81972=CARTESIAN_POINT('Ctrl Pts',(-0.107313058275478,0.163751393132007,
-0.903220929511266));
#81973=CARTESIAN_POINT('Ctrl Pts',(-0.117375341855184,0.15669638402423,
-0.902525640932798));
#81974=CARTESIAN_POINT('Ctrl Pts',(-0.126686456383126,0.148767273851093,
-0.90183035235433));
#81975=CARTESIAN_POINT('Ctrl Pts',(-0.135997130929772,0.140838538354927,
-0.901135096630573));
#81976=CARTESIAN_POINT('Ctrl Pts',(-0.144556058695458,0.13203637152894,
-0.900439840906815));
#81977=CARTESIAN_POINT('Ctrl Pts',(-0.152207903038364,0.122531278670648,
-0.899744585183057));
#81978=CARTESIAN_POINT('Ctrl Pts',(-0.15987724574609,0.11300444940803,-0.899047739536955));
#81979=CARTESIAN_POINT('Ctrl Pts',(-0.166634866901655,0.102772206786369,
-0.898350893890853));
#81980=CARTESIAN_POINT('Ctrl Pts',(-0.172367766296594,0.0920353907033747,
-0.89765404824475));
#81981=CARTESIAN_POINT('Ctrl Pts',(-0.174138573060907,0.0887189490152927,
-0.89743880306098));
#81982=CARTESIAN_POINT('Ctrl Pts',(-0.175811949310168,0.0853545311005462,
-0.89722355787721));
#81983=CARTESIAN_POINT('Ctrl Pts',(-0.17738549331188,0.0819484396587333,
-0.89700831269344));
#81984=CARTESIAN_POINT('Ctrl Pts',(-0.182914406178021,0.0699805615597355,
-0.8962520123519));
#81985=CARTESIAN_POINT('Ctrl Pts',(-0.187241060727249,0.0574235374384502,
-0.89549571201036));
#81986=CARTESIAN_POINT('Ctrl Pts',(-0.190259811913753,0.0445237461422927,
-0.89473941166882));
#81987=CARTESIAN_POINT('Ctrl Pts',(-0.193259450024786,0.0317056292437173,
-0.893987899805898));
#81988=CARTESIAN_POINT('Ctrl Pts',(-0.194967423098108,0.0185496467069044,
-0.893236387942975));
#81989=CARTESIAN_POINT('Ctrl Pts',(-0.195327639122108,0.00531727326583664,
-0.892484876080052));
#81990=CARTESIAN_POINT('Ctrl Pts',(-0.195375236304858,0.00356881218990247,
-0.892385574979892));
#81991=CARTESIAN_POINT('Ctrl Pts',(-0.195399373672046,0.00181903830544178,
-0.892286273879733));
#81992=CARTESIAN_POINT('Ctrl Pts',(-0.195399987967877,6.85722511850599E-5,
-0.892186972779573));
#81993=CARTESIAN_POINT('',(-0.195366936014536,-0.0001759764390597,-0.822186969212424));
#81994=CARTESIAN_POINT('Ctrl Pts',(-0.195104707912954,6.84058415591362E-5,
-0.892186969212424));
#81995=CARTESIAN_POINT('Ctrl Pts',(-0.19499122330115,-0.0366782010199141,
-0.890099241453403));
#81996=CARTESIAN_POINT('Ctrl Pts',(-0.167386274654172,-0.138618456874515,
-0.884316671441687));
#81997=CARTESIAN_POINT('Ctrl Pts',(-0.00315354223898925,-0.230724950314991,
-0.874839259177279));
#81998=CARTESIAN_POINT('Ctrl Pts',(0.191799192978493,-0.128288297037242,
-0.8637547324192));
#81999=CARTESIAN_POINT('Ctrl Pts',(0.212042795889746,0.0910094176328911,
-0.852670205661119));
#82000=CARTESIAN_POINT('Ctrl Pts',(0.03913571544926,0.227404907853978,-0.841585678903039));
#82001=CARTESIAN_POINT('Ctrl Pts',(-0.152045168436665,0.162551660997725,
-0.831424600086807));
#82002=CARTESIAN_POINT('Ctrl Pts',(-0.194931245944501,0.0484383113115352,
-0.824958363523269));
#82003=CARTESIAN_POINT('Ctrl Pts',(-0.195366936014536,-0.0001759764390597,
-0.822186969212424));
#82004=CARTESIAN_POINT('',(-0.195681094571072,7.47969092022707E-5,-0.752186969212423));
#82005=CARTESIAN_POINT('Ctrl Pts',(-0.195366936014536,-0.0001759764390597,
-0.822186969212424));
#82006=CARTESIAN_POINT('Ctrl Pts',(-0.195512110989054,-0.0163745966758234,
-0.821263521270576));
#82007=CARTESIAN_POINT('Ctrl Pts',(-0.186273967132678,-0.09722283275531,
-0.81664523107603));
#82008=CARTESIAN_POINT('Ctrl Pts',(-0.074157745877468,-0.218507032466107,
-0.808332098628802));
#82009=CARTESIAN_POINT('Ctrl Pts',(0.142885639710072,-0.181186120176718,
-0.797247571870717));
#82010=CARTESIAN_POINT('Ctrl Pts',(0.229774287535425,0.0211775855982428,
-0.78616304511264));
#82011=CARTESIAN_POINT('Ctrl Pts',(0.107361153908771,0.204250560881833,
-0.775078518354558));
#82012=CARTESIAN_POINT('Ctrl Pts',(-0.112847422116822,0.201271387892123,
-0.76399399159648));
#82013=CARTESIAN_POINT('Ctrl Pts',(-0.193675615340973,0.0730115495022533,
-0.756363475215766));
#82014=CARTESIAN_POINT('Ctrl Pts',(-0.195701748231673,0.00428175194181416,
-0.752427801087748));
#82015=CARTESIAN_POINT('Ctrl Pts',(-0.195681094571072,7.47969092022707E-5,
-0.752186969212423));
#82016=CARTESIAN_POINT('',(-0.19515607959856,0.000116101941455404,-0.682186969212424));
#82017=CARTESIAN_POINT('Ctrl Pts',(-0.195681094571072,7.47969092022707E-5,
-0.752186969212423));
#82018=CARTESIAN_POINT('Ctrl Pts',(-0.195384879803195,-0.060261345555979,
-0.748732958835055));
#82019=CARTESIAN_POINT('Ctrl Pts',(-0.133195868508463,-0.185668250759869,
-0.741584106204994));
#82020=CARTESIAN_POINT('Ctrl Pts',(0.0800418565502769,-0.216420915704385,
-0.730740411322238));
#82021=CARTESIAN_POINT('Ctrl Pts',(0.225105205951166,-0.0507184155460289,
-0.719655884564159));
#82022=CARTESIAN_POINT('Ctrl Pts',(0.165119859323233,0.161183570570169,
-0.708571357806077));
#82023=CARTESIAN_POINT('Ctrl Pts',(-0.0452734338024108,0.226263182214096,
-0.697486831048));
#82024=CARTESIAN_POINT('Ctrl Pts',(-0.179485015703818,0.114370598042359,
-0.688692034850112));
#82025=CARTESIAN_POINT('Ctrl Pts',(-0.195290790666625,0.0248312161815972,
-0.683592080904922));
#82026=CARTESIAN_POINT('Ctrl Pts',(-0.19515607959856,0.000116101941455404,
-0.682186969212424));
#82027=CARTESIAN_POINT('',(-0.195399931967772,-0.000163055175443911,-0.612186967161044));
#82028=CARTESIAN_POINT('Ctrl Pts',(-0.19515607959856,0.000116101941455404,
-0.682186969212424));
#82029=CARTESIAN_POINT('Ctrl Pts',(-0.194936558224572,-0.0401589542526584,
-0.679897238652229));
#82030=CARTESIAN_POINT('Ctrl Pts',(-0.163203532909971,-0.145741425442279,
-0.67391266583934));
#82031=CARTESIAN_POINT('Ctrl Pts',(0.00939477616280343,-0.230556825089081,
-0.664233250773757));
#82032=CARTESIAN_POINT('Ctrl Pts',(0.198490591378379,-0.117669862515987,
-0.653148724015678));
#82033=CARTESIAN_POINT('Ctrl Pts',(0.206781006218889,0.102402767916716,
-0.642064197257598));
#82034=CARTESIAN_POINT('Ctrl Pts',(0.0267142684199375,0.229196551618941,
-0.630979670499519));
#82035=CARTESIAN_POINT('Ctrl Pts',(-0.15693301120472,0.155538717273989,
-0.621020594484459));
#82036=CARTESIAN_POINT('Ctrl Pts',(-0.194907926478866,0.0449665939000981,
-0.614756360722095));
#82037=CARTESIAN_POINT('Ctrl Pts',(-0.19526695444957,-0.000162908179064867,
-0.612186969212424));
#82038=CARTESIAN_POINT('',(-0.195399999600512,1.24947932985652E-5,-0.542186969209066));
#82039=CARTESIAN_POINT('Ctrl Pts',(-0.195399931967772,-0.000163055175443911,
-0.612186967161044));
#82040=CARTESIAN_POINT('Ctrl Pts',(-0.195387649960393,-0.0148814067991219,
-0.611349560425973));
#82041=CARTESIAN_POINT('Ctrl Pts',(-0.193708372206648,-0.0295270808785863,
-0.610512153690901));
#82042=CARTESIAN_POINT('Ctrl Pts',(-0.19043429106854,-0.0437714608531942,
-0.60967474695583));
#82043=CARTESIAN_POINT('Ctrl Pts',(-0.189308103309253,-0.0486711092398252,
-0.609386703631673));
#82044=CARTESIAN_POINT('Ctrl Pts',(-0.187993644156325,-0.0535234622546284,
-0.609098660307515));
#82045=CARTESIAN_POINT('Ctrl Pts',(-0.186495138743599,-0.0583157202219598,
-0.608810616983358));
#82046=CARTESIAN_POINT('Ctrl Pts',(-0.182870726121707,-0.069906682868242,
-0.608113930904775));
#82047=CARTESIAN_POINT('Ctrl Pts',(-0.178148868935771,-0.0811991380356456,
-0.607417244826192));
#82048=CARTESIAN_POINT('Ctrl Pts',(-0.172400175377746,-0.0919746678695959,
-0.606720558747608));
#82049=CARTESIAN_POINT('Ctrl Pts',(-0.166663476446175,-0.102727714603012,
-0.606025326301783));
#82050=CARTESIAN_POINT('Ctrl Pts',(-0.159904536385181,-0.112965177748617,
-0.605330093855957));
#82051=CARTESIAN_POINT('Ctrl Pts',(-0.152241585329039,-0.122489426876367,
-0.604634861410131));
#82052=CARTESIAN_POINT('Ctrl Pts',(-0.144579692509108,-0.132012360726853,
-0.603939724974334));
#82053=CARTESIAN_POINT('Ctrl Pts',(-0.136014548859102,-0.140821566983641,
-0.603244588538537));
#82054=CARTESIAN_POINT('Ctrl Pts',(-0.126706245102679,-0.148750420006062,
-0.60254945210274));
#82055=CARTESIAN_POINT('Ctrl Pts',(-0.117398424234648,-0.156678861702082,
-0.601854351728648));
#82056=CARTESIAN_POINT('Ctrl Pts',(-0.107348203422377,-0.163726494047941,
-0.601159251354557));
#82057=CARTESIAN_POINT('Ctrl Pts',(-0.0967485603789931,-0.169767123037979,
-0.600464150980466));
#82058=CARTESIAN_POINT('Ctrl Pts',(-0.0861247016104804,-0.175821552323992,
-0.599767462594446));
#82059=CARTESIAN_POINT('Ctrl Pts',(-0.0749497067662055,-0.180864009385805,
-0.599070774208426));
#82060=CARTESIAN_POINT('Ctrl Pts',(-0.0634397670242631,-0.184814923531373,
-0.598374085822406));
#82061=CARTESIAN_POINT('Ctrl Pts',(-0.059871270488526,-0.186039849443893,
-0.59815808729003));
#82062=CARTESIAN_POINT('Ctrl Pts',(-0.0562706882353161,-0.187160216173435,
-0.597942088757653));
#82063=CARTESIAN_POINT('Ctrl Pts',(-0.0526446969434173,-0.188174641978498,
-0.597726090225277));
#82064=CARTESIAN_POINT('Ctrl Pts',(-0.0409493505614043,-0.191446591692103,
-0.597029404146688));
#82065=CARTESIAN_POINT('Ctrl Pts',(-0.0289067584796694,-0.19363553092092,
-0.5963327180681));
#82066=CARTESIAN_POINT('Ctrl Pts',(-0.0167385637002627,-0.194681741530253,
-0.595636031989512));
#82067=CARTESIAN_POINT('Ctrl Pts',(-0.00459575781131094,-0.195725769225272,
-0.594940799543681));
#82068=CARTESIAN_POINT('Ctrl Pts',(0.00767127380048421,-0.195631653110166,
-0.59424556709785));
#82069=CARTESIAN_POINT('Ctrl Pts',(0.0198323906566823,-0.194390936725046,
-0.593550334652019));
#82070=CARTESIAN_POINT('Ctrl Pts',(0.0319918280901456,-0.193150391680052,
-0.592855198216217));
#82071=CARTESIAN_POINT('Ctrl Pts',(0.04404450606983,-0.190763604270154,
-0.592160061780414));
#82072=CARTESIAN_POINT('Ctrl Pts',(0.0557634935802237,-0.187274111354795,
-0.591464925344612));
#82073=CARTESIAN_POINT('Ctrl Pts',(0.0674818731427938,-0.18378479946443,
-0.590769824970516));
#82074=CARTESIAN_POINT('Ctrl Pts',(0.0788657657328716,-0.179193171261107,
-0.590074724596419));
#82075=CARTESIAN_POINT('Ctrl Pts',(0.0897042429323871,-0.173592363887146,
-0.589379624222323));
#82076=CARTESIAN_POINT('Ctrl Pts',(0.100567481492599,-0.167978761024573,
-0.588682935836298));
#82077=CARTESIAN_POINT('Ctrl Pts',(0.11088207040143,-0.161351835747051,
-0.587986247450273));
#82078=CARTESIAN_POINT('Ctrl Pts',(0.12046354468802,-0.153849583688736,
-0.587289559064248));
#82079=CARTESIAN_POINT('Ctrl Pts',(0.123434147363716,-0.151523614910699,
-0.587073560531898));
#82080=CARTESIAN_POINT('Ctrl Pts',(0.126334525481837,-0.14911379729535,
-0.586857561999547));
#82081=CARTESIAN_POINT('Ctrl Pts',(0.129159884355811,-0.146624978339959,
-0.586641563467197));
#82082=CARTESIAN_POINT('Ctrl Pts',(0.138272854583456,-0.138597490840445,
-0.585944877388607));
#82083=CARTESIAN_POINT('Ctrl Pts',(0.146666564977586,-0.129689005850555,
-0.585248191310016));
#82084=CARTESIAN_POINT('Ctrl Pts',(0.154170232694714,-0.120052902300851,
-0.584551505231425));
#82085=CARTESIAN_POINT('Ctrl Pts',(0.161658244038721,-0.11043690444323,
-0.583856272785592));
#82086=CARTESIAN_POINT('Ctrl Pts',(0.168259308287332,-0.10009693958862,
-0.583161040339758));
#82087=CARTESIAN_POINT('Ctrl Pts',(0.173841009951574,-0.0892214282502628,
-0.582465807893925));
#82088=CARTESIAN_POINT('Ctrl Pts',(0.17942194079544,-0.0783474187954233,
-0.58177067145812));
#82089=CARTESIAN_POINT('Ctrl Pts',(0.183983349260585,-0.0669387662265575,
-0.581075535022315));
#82090=CARTESIAN_POINT('Ctrl Pts',(0.187438175868307,-0.055209512107621,
-0.58038039858651));
#82091=CARTESIAN_POINT('Ctrl Pts',(0.190892823249427,-0.0434808664691095,
-0.579685298212411));
#82092=CARTESIAN_POINT('Ctrl Pts',(0.193240781464953,-0.0314324992652491,
-0.578990197838312));
#82093=CARTESIAN_POINT('Ctrl Pts',(0.194445306428671,-0.0192920400129258,
-0.578295097464213));
#82094=CARTESIAN_POINT('Ctrl Pts',(0.195652583225192,-0.00712384491865252,
-0.577598409078185));
#82095=CARTESIAN_POINT('Ctrl Pts',(0.195711190497023,0.00513598575638776,
-0.576901720692157));
#82096=CARTESIAN_POINT('Ctrl Pts',(0.194636418920523,0.017257590497937,
-0.576205032306129));
#82097=CARTESIAN_POINT('Ctrl Pts',(0.194303200959987,0.0210157252483613,
-0.575989033773791));
#82098=CARTESIAN_POINT('Ctrl Pts',(0.193861415829799,0.0247606204490827,
-0.575773035241454));
#82099=CARTESIAN_POINT('Ctrl Pts',(0.193312518323342,0.0284856149571576,
-0.575557036709117));
#82100=CARTESIAN_POINT('Ctrl Pts',(0.191542093093218,0.0405002883371504,
-0.574860350630529));
#82101=CARTESIAN_POINT('Ctrl Pts',(0.188641077440746,0.0523914441757711,
-0.574163664551941));
#82102=CARTESIAN_POINT('Ctrl Pts',(0.184645115049052,0.063932319592851,
-0.573466978473353));
#82103=CARTESIAN_POINT('Ctrl Pts',(0.180657490217141,0.0754491150188532,
-0.572771746027523));
#82104=CARTESIAN_POINT('Ctrl Pts',(0.175579667013763,0.0866162379215019,
-0.572076513581693));
#82105=CARTESIAN_POINT('Ctrl Pts',(0.169497572422247,0.097220023364351,
-0.571381281135863));
#82106=CARTESIAN_POINT('Ctrl Pts',(0.163416317754239,0.107822344448413,
-0.570686144700061));
#82107=CARTESIAN_POINT('Ctrl Pts',(0.156331462364505,0.117860702119283,
-0.56999100826426));
#82108=CARTESIAN_POINT('Ctrl Pts',(0.148375120930957,0.12714552091491,-0.569295871828458));
#82109=CARTESIAN_POINT('Ctrl Pts',(0.140419192249829,0.136429858040481,
-0.568600771454362));
#82110=CARTESIAN_POINT('Ctrl Pts',(0.131592457158933,0.144960087093375,
-0.567905671080266));
#82111=CARTESIAN_POINT('Ctrl Pts',(0.122065826151406,0.15258143427683,-0.567210570706171));
#82112=CARTESIAN_POINT('Ctrl Pts',(0.112517430799842,0.16022019303233,-0.566513882320146));
#82113=CARTESIAN_POINT('Ctrl Pts',(0.102266670976131,0.166945429535853,
-0.565817193934121));
#82114=CARTESIAN_POINT('Ctrl Pts',(0.0915146647020496,0.172644797617743,
-0.565120505548097));
#82115=CARTESIAN_POINT('Ctrl Pts',(0.0881811548838333,0.174411807324983,
-0.564904507015744));
#82116=CARTESIAN_POINT('Ctrl Pts',(0.084799629294112,0.176080549022716,
-0.564688508483391));
#82117=CARTESIAN_POINT('Ctrl Pts',(0.0813764670325799,0.177648615568192,
-0.564472509951038));
#82118=CARTESIAN_POINT('Ctrl Pts',(0.0703353295471433,0.182706289435856,
-0.563775823872449));
#82119=CARTESIAN_POINT('Ctrl Pts',(0.0587821276928241,0.186748443058392,
-0.56307913779386));
#82120=CARTESIAN_POINT('Ctrl Pts',(0.046926463790817,0.18968148827993,-0.562382451715271));
#82121=CARTESIAN_POINT('Ctrl Pts',(0.0350955366848213,0.192608413714171,
-0.561687219269439));
#82122=CARTESIAN_POINT('Ctrl Pts',(0.0229642233891814,0.194430544371172,
-0.560991986823608));
#82123=CARTESIAN_POINT('Ctrl Pts',(0.0107585223315926,0.19510359862709,
-0.560296754377776));
#82124=CARTESIAN_POINT('Ctrl Pts',(-0.00144549314628636,0.195776559935737,
-0.559601617941973));
#82125=CARTESIAN_POINT('Ctrl Pts',(-0.0137230061700573,0.195300666488192,
-0.558906481506169));
#82126=CARTESIAN_POINT('Ctrl Pts',(-0.02584307137875,0.19368349351897,-0.558211345070366));
#82127=CARTESIAN_POINT('Ctrl Pts',(-0.0379625078328463,0.192066404444093,
-0.557516244696269));
#82128=CARTESIAN_POINT('Ctrl Pts',(-0.0499236489753525,0.189308295920255,
-0.556821144322172));
#82129=CARTESIAN_POINT('Ctrl Pts',(-0.0615036123781013,0.185468233572341,
-0.556126043948074));
#82130=CARTESIAN_POINT('Ctrl Pts',(-0.0731100311255822,0.18161939829746,
-0.555429355562048));
#82131=CARTESIAN_POINT('Ctrl Pts',(-0.0843327243602488,0.176684011833073,
-0.554732667176022));
#82132=CARTESIAN_POINT('Ctrl Pts',(-0.0949679454458698,0.170769579661573,
-0.554035978789996));
#82133=CARTESIAN_POINT('Ctrl Pts',(-0.0982652476425931,0.168935892328281,
-0.55381998025765));
#82134=CARTESIAN_POINT('Ctrl Pts',(-0.101506276568824,0.167008421014308,
-0.553603981725303));
#82135=CARTESIAN_POINT('Ctrl Pts',(-0.104685539550776,0.164991205247319,
-0.553387983192956));
#82136=CARTESIAN_POINT('Ctrl Pts',(-0.114939999317868,0.158484836305347,
-0.552691297114367));
#82137=CARTESIAN_POINT('Ctrl Pts',(-0.124621557139461,0.150995983446465,
-0.551994611035779));
#82138=CARTESIAN_POINT('Ctrl Pts',(-0.133537579149304,0.142649482841486,
-0.55129792495719));
#82139=CARTESIAN_POINT('Ctrl Pts',(-0.14243499791436,0.134320397177128,
-0.550602692511358));
#82140=CARTESIAN_POINT('Ctrl Pts',(-0.150569368421779,0.125137753829151,
-0.549907460065527));
#82141=CARTESIAN_POINT('Ctrl Pts',(-0.157780483132415,0.115266990689016,
-0.549212227619695));
#82142=CARTESIAN_POINT('Ctrl Pts',(-0.164990602004419,0.105397590678945,
-0.548517091183892));
#82143=CARTESIAN_POINT('Ctrl Pts',(-0.171277166213182,0.0948409382232021,
-0.547821954748089));
#82144=CARTESIAN_POINT('Ctrl Pts',(-0.176520768217102,0.0837948589595091,
-0.547126818312286));
#82145=CARTESIAN_POINT('Ctrl Pts',(-0.181764098197827,0.0727493527350705,
-0.546431717938189));
#82146=CARTESIAN_POINT('Ctrl Pts',(-0.185964222600671,0.0612152721448906,
-0.545736617564093));
#82147=CARTESIAN_POINT('Ctrl Pts',(-0.189049311026348,0.0494117192623678,
-0.545041517189996));
#82148=CARTESIAN_POINT('Ctrl Pts',(-0.192141447581195,0.037581200227212,
-0.54434482880397));
#82149=CARTESIAN_POINT('Ctrl Pts',(-0.194113304827838,0.0254808422989893,
-0.543648140417944));
#82150=CARTESIAN_POINT('Ctrl Pts',(-0.194944100655711,0.0133400756945423,
-0.542951452031918));
#82151=CARTESIAN_POINT('Ctrl Pts',(-0.195201677332887,0.00957600007519466,
-0.542735453499571));
#82152=CARTESIAN_POINT('Ctrl Pts',(-0.195349951110585,0.0058080524835065,
-0.542519454967224));
#82153=CARTESIAN_POINT('Ctrl Pts',(-0.195389319026348,0.00204303950528141,
-0.542303456434878));
#82154=CARTESIAN_POINT('Ctrl Pts',(-0.195396396017583,0.00136622023931689,
-0.542264627360726));
#82155=CARTESIAN_POINT('Ctrl Pts',(-0.195399956318106,0.000689364137931553,
-0.542225798286575));
#82156=CARTESIAN_POINT('Ctrl Pts',(-0.195399999600508,1.24948518317515E-5,
-0.542186969212424));
#82157=CARTESIAN_POINT('',(-0.19539994003323,0.000153084976888024,-0.472186969216991));
#82158=CARTESIAN_POINT('Ctrl Pts',(-0.195399999600512,1.24947932979144E-5,
-0.542186969209066));
#82159=CARTESIAN_POINT('Ctrl Pts',(-0.195400774759589,-0.0121098412592945,
-0.541491563027797));
#82160=CARTESIAN_POINT('Ctrl Pts',(-0.194269147082837,-0.0242755331708231,
-0.540796156846527));
#82161=CARTESIAN_POINT('Ctrl Pts',(-0.192006980379885,-0.0362557510665349,
-0.540100750665258));
#82162=CARTESIAN_POINT('Ctrl Pts',(-0.189749524678251,-0.0482110199510932,
-0.539406792679399));
#82163=CARTESIAN_POINT('Ctrl Pts',(-0.186366290974367,-0.0599807128695843,
-0.53871283469354));
#82164=CARTESIAN_POINT('Ctrl Pts',(-0.181910805132108,-0.0713415655574515,
-0.538018876707681));
#82165=CARTESIAN_POINT('Ctrl Pts',(-0.177455905552505,-0.0827009233592614,
-0.537325010034345));
#82166=CARTESIAN_POINT('Ctrl Pts',(-0.171929312599577,-0.0936507146707394,
-0.536631143361008));
#82167=CARTESIAN_POINT('Ctrl Pts',(-0.165433757398891,-0.10398476769645,
-0.535937276687672));
#82168=CARTESIAN_POINT('Ctrl Pts',(-0.158938385641453,-0.114318528874554,
-0.535243429610067));
#82169=CARTESIAN_POINT('Ctrl Pts',(-0.151474597899374,-0.124035857891667,
-0.534549582532462));
#82170=CARTESIAN_POINT('Ctrl Pts',(-0.143188554114146,-0.132959384665771,
-0.533855735454857));
#82171=CARTESIAN_POINT('Ctrl Pts',(-0.134883733044484,-0.141903133346097,
-0.533160316026892));
#82172=CARTESIAN_POINT('Ctrl Pts',(-0.125753584127312,-0.150048893232625,
-0.532464896598927));
#82173=CARTESIAN_POINT('Ctrl Pts',(-0.115980235201907,-0.157256939568689,
-0.531769477170962));
#82174=CARTESIAN_POINT('Ctrl Pts',(-0.113401123688238,-0.159159087485262,
-0.531585961339573));
#82175=CARTESIAN_POINT('Ctrl Pts',(-0.110777377410633,-0.160996168259883,
-0.531402445508185));
#82176=CARTESIAN_POINT('Ctrl Pts',(-0.108112652127949,-0.162766134222881,
-0.531218929676797));
#82177=CARTESIAN_POINT('Ctrl Pts',(-0.0979964839823108,-0.169485503536523,
-0.530522243598208));
#82178=CARTESIAN_POINT('Ctrl Pts',(-0.0872159900895472,-0.175281746321541,
-0.529825557519619));
#82179=CARTESIAN_POINT('Ctrl Pts',(-0.0759635920383071,-0.180029699451612,
-0.52912887144103));
#82180=CARTESIAN_POINT('Ctrl Pts',(-0.0647346720712546,-0.184767745996189,
-0.528433638995198));
#82181=CARTESIAN_POINT('Ctrl Pts',(-0.0530365717809753,-0.188461439541515,
-0.527738406549367));
#82182=CARTESIAN_POINT('Ctrl Pts',(-0.0410856054130471,-0.191031759212554,
-0.527043174103535));
#82183=CARTESIAN_POINT('Ctrl Pts',(-0.0291362894465465,-0.19360172392826,
-0.526348037667732));
#82184=CARTESIAN_POINT('Ctrl Pts',(-0.0169350213056709,-0.195048394718982,
-0.525652901231929));
#82185=CARTESIAN_POINT('Ctrl Pts',(-0.00471109725244599,-0.195343199427771,
-0.524957764796126));
#82186=CARTESIAN_POINT('Ctrl Pts',(0.00751219265827948,-0.195637988842929,
-0.524262664422029));
#82187=CARTESIAN_POINT('Ctrl Pts',(0.0197572607745834,-0.194781036751348,
-0.523567564047932));
#82188=CARTESIAN_POINT('Ctrl Pts',(0.0317947363763054,-0.192795888801502,
-0.522872463673835));
#82189=CARTESIAN_POINT('Ctrl Pts',(0.0438597125456626,-0.190806205623735,
-0.522175775287809));
#82190=CARTESIAN_POINT('Ctrl Pts',(0.0557152973938653,-0.187683387841771,
-0.521479086901783));
#82191=CARTESIAN_POINT('Ctrl Pts',(0.067143459072765,-0.183501814442648,
-0.520782398515756));
#82192=CARTESIAN_POINT('Ctrl Pts',(0.0706866014583335,-0.18220537584079,
-0.52056639998341));
#82193=CARTESIAN_POINT('Ctrl Pts',(0.0741888018429137,-0.180807517967788,
-0.520350401451063));
#82194=CARTESIAN_POINT('Ctrl Pts',(0.0776440042616577,-0.179311373320868,
-0.520134402918717));
#82195=CARTESIAN_POINT('Ctrl Pts',(0.0887884847249885,-0.174485677813866,
-0.519437716840128));
#82196=CARTESIAN_POINT('Ctrl Pts',(0.0995204703340839,-0.168600105294485,
-0.518741030761539));
#82197=CARTESIAN_POINT('Ctrl Pts',(0.109630200136307,-0.161747887831877,
-0.51804434468295));
#82198=CARTESIAN_POINT('Ctrl Pts',(0.11971883602714,-0.154909967493999,
-0.517349112237119));
#82199=CARTESIAN_POINT('Ctrl Pts',(0.129187034635739,-0.147109830474931,
-0.516653879791288));
#82200=CARTESIAN_POINT('Ctrl Pts',(0.137850725122369,-0.138485875031488,
-0.515958647345456));
#82201=CARTESIAN_POINT('Ctrl Pts',(0.146513219172936,-0.129863110536789,
-0.515263510909653));
#82202=CARTESIAN_POINT('Ctrl Pts',(0.154370774492035,-0.120417337671136,
-0.51456837447385));
#82203=CARTESIAN_POINT('Ctrl Pts',(0.161274563691475,-0.110325314892478,
-0.513873238038047));
#82204=CARTESIAN_POINT('Ctrl Pts',(0.16817799474192,-0.100233815659326,
-0.51317813766395));
#82205=CARTESIAN_POINT('Ctrl Pts',(0.174127286203008,-0.0894968705085294,
-0.512483037289853));
#82206=CARTESIAN_POINT('Ctrl Pts',(0.179017282850342,-0.0783196810570658,
-0.511787936915756));
#82207=CARTESIAN_POINT('Ctrl Pts',(0.183918451082812,-0.0671169564299077,
-0.51109124852973));
#82208=CARTESIAN_POINT('Ctrl Pts',(0.187755202693892,-0.0554728068230441,
-0.510394560143704));
#82209=CARTESIAN_POINT('Ctrl Pts',(0.190471192423205,-0.0436106048671915,
-0.509697871757678));
#82210=CARTESIAN_POINT('Ctrl Pts',(0.19131324721724,-0.0399328943379754,
-0.509481873225331));
#82211=CARTESIAN_POINT('Ctrl Pts',(0.192047943803405,-0.0362342952662712,
-0.509265874692984));
#82212=CARTESIAN_POINT('Ctrl Pts',(0.192674611726904,-0.0325215927636833,
-0.509049876160637));
#82213=CARTESIAN_POINT('Ctrl Pts',(0.194695879248751,-0.0205465662698088,
-0.508353190082048));
#82214=CARTESIAN_POINT('Ctrl Pts',(0.195603573544156,-0.00834035596272215,
-0.507656504003459));
#82215=CARTESIAN_POINT('Ctrl Pts',(0.195361665887142,0.00387033613536681,
-0.50695981792487));
#82216=CARTESIAN_POINT('Ctrl Pts',(0.195120262969501,0.0160555506725137,
-0.506264585479039));
#82217=CARTESIAN_POINT('Ctrl Pts',(0.193733962486938,0.0282443608433282,
-0.505569353033207));
#82218=CARTESIAN_POINT('Ctrl Pts',(0.19121860743086,0.0402070164548739,
-0.504874120587376));
#82219=CARTESIAN_POINT('Ctrl Pts',(0.188703599739626,0.052168020050737,
-0.504178984151573));
#82220=CARTESIAN_POINT('Ctrl Pts',(0.185059982402041,0.0639020668087616,
-0.50348384771577));
#82221=CARTESIAN_POINT('Ctrl Pts',(0.1803549640121,0.0751880772210209,-0.502788711279967));
#82222=CARTESIAN_POINT('Ctrl Pts',(0.175650189705162,0.086473502147082,
-0.50209361090587));
#82223=CARTESIAN_POINT('Ctrl Pts',(0.169884485307396,0.0973101396725234,
-0.501398510531773));
#82224=CARTESIAN_POINT('Ctrl Pts',(0.163172697153958,0.107498050696293,
-0.500703410157675));
#82225=CARTESIAN_POINT('Ctrl Pts',(0.156445575388213,0.117709236810736,
-0.50000672177165));
#82226=CARTESIAN_POINT('Ctrl Pts',(0.148768590520948,0.12726804355321,-0.499310033385624));
#82227=CARTESIAN_POINT('Ctrl Pts',(0.140298408868267,0.136005575139523,
-0.498613344999598));
#82228=CARTESIAN_POINT('Ctrl Pts',(0.137672346998442,0.138714525133288,
-0.498397346467251));
#82229=CARTESIAN_POINT('Ctrl Pts',(0.134970303478862,0.141344805533783,
-0.498181347934904));
#82230=CARTESIAN_POINT('Ctrl Pts',(0.132197604083141,0.143892159184151,
-0.497965349402556));
#82231=CARTESIAN_POINT('Ctrl Pts',(0.123254482812271,0.152108445684661,
-0.497268663323968));
#82232=CARTESIAN_POINT('Ctrl Pts',(0.113511065593818,0.159516637090257,
-0.496571977245379));
#82233=CARTESIAN_POINT('Ctrl Pts',(0.103137874553166,0.165963064663965,
-0.49587529116679));
#82234=CARTESIAN_POINT('Ctrl Pts',(0.092786327134741,0.172396041791944,
-0.495180058720958));
#82235=CARTESIAN_POINT('Ctrl Pts',(0.0818083109103004,0.177870718237551,
-0.494484826275126));
#82236=CARTESIAN_POINT('Ctrl Pts',(0.0704051512959251,0.182275271693661,
-0.493789593829295));
#82237=CARTESIAN_POINT('Ctrl Pts',(0.0590035664321041,0.186679216890899,
-0.493094457393492));
#82238=CARTESIAN_POINT('Ctrl Pts',(0.047177753357304,0.190012975391768,
-0.492399320957689));
#82239=CARTESIAN_POINT('Ctrl Pts',(0.0351497362308519,0.19221252831931,
-0.491704184521886));
#82240=CARTESIAN_POINT('Ctrl Pts',(0.0231223430838024,0.194411967140287,
-0.491009084147789));
#82241=CARTESIAN_POINT('Ctrl Pts',(0.0108936322782355,0.195477186410669,
-0.490313983773692));
#82242=CARTESIAN_POINT('Ctrl Pts',(-0.00130616200337565,0.195395634395503,
-0.489618883399595));
#82243=CARTESIAN_POINT('Ctrl Pts',(-0.0135338276825206,0.19531389606829,
-0.488922195013569));
#82244=CARTESIAN_POINT('Ctrl Pts',(-0.0257315711095326,0.194080227441351,
-0.488225506627542));
#82245=CARTESIAN_POINT('Ctrl Pts',(-0.0376724219922772,0.191734057019706,
-0.487528818241516));
#82246=CARTESIAN_POINT('Ctrl Pts',(-0.0413745165260365,0.191006659552094,
-0.48731281970917));
#82247=CARTESIAN_POINT('Ctrl Pts',(-0.045052004343916,0.190172694615065,
-0.487096821176823));
#82248=CARTESIAN_POINT('Ctrl Pts',(-0.0486984146996827,0.189234310857565,
-0.486880822644477));
#82249=CARTESIAN_POINT('Ctrl Pts',(-0.0604596211490331,0.186207628717083,
-0.486184136565888));
#82250=CARTESIAN_POINT('Ctrl Pts',(-0.0719788553954887,0.182069667701086,
-0.4854874504873));
#82251=CARTESIAN_POINT('Ctrl Pts',(-0.0830343733418138,0.176879769458614,
-0.484790764408711));
#82252=CARTESIAN_POINT('Ctrl Pts',(-0.0940668239935134,0.17170069991837,
-0.48409553196288));
#82253=CARTESIAN_POINT('Ctrl Pts',(-0.104636663244794,0.165474351019529,
-0.483400299517049));
#82254=CARTESIAN_POINT('Ctrl Pts',(-0.114540470901671,0.158308687460996,
-0.482705067071217));
#82255=CARTESIAN_POINT('Ctrl Pts',(-0.124442910865109,0.151144013464396,
-0.482009930635415));
#82256=CARTESIAN_POINT('Ctrl Pts',(-0.133678767441387,0.143040757703623,
-0.481314794199612));
#82257=CARTESIAN_POINT('Ctrl Pts',(-0.142073443071281,0.13415027683114,
-0.480619657763809));
#82258=CARTESIAN_POINT('Ctrl Pts',(-0.150467683209224,0.125260257171577,
-0.479924557389713));
#82259=CARTESIAN_POINT('Ctrl Pts',(-0.158020247992978,0.115583748232537,
-0.479229457015616));
#82260=CARTESIAN_POINT('Ctrl Pts',(-0.16459523608154,0.105307019040814,
-0.478534356641519));
#82261=CARTESIAN_POINT('Ctrl Pts',(-0.171185245251811,0.0950068118462686,
-0.477837668255493));
#82262=CARTESIAN_POINT('Ctrl Pts',(-0.176792803044107,0.0841044185953307,
-0.477140979869468));
#82263=CARTESIAN_POINT('Ctrl Pts',(-0.181327382796066,0.0728116765933106,
-0.476444291483442));
#82264=CARTESIAN_POINT('Ctrl Pts',(-0.18273326610184,0.0693105191927391,
-0.476228292951094));
#82265=CARTESIAN_POINT('Ctrl Pts',(-0.184036368623349,0.0657719689266645,
-0.476012294418746));
#82266=CARTESIAN_POINT('Ctrl Pts',(-0.185234968854937,0.0622026230420426,
-0.475796295886397));
#82267=CARTESIAN_POINT('Ctrl Pts',(-0.189780639450348,0.0486659406645715,
-0.474977125197729));
#82268=CARTESIAN_POINT('Ctrl Pts',(-0.192845581036781,0.0346083663153122,
-0.474157954509061));
#82269=CARTESIAN_POINT('Ctrl Pts',(-0.194339139427583,0.0203336884638898,
-0.473338783820393));
#82270=CARTESIAN_POINT('Ctrl Pts',(-0.195039157299054,0.0136432706891088,
-0.472954845619259));
#82271=CARTESIAN_POINT('Ctrl Pts',(-0.195394649920554,0.00690546343110999,
-0.472570907418125));
#82272=CARTESIAN_POINT('Ctrl Pts',(-0.19539994003323,0.000153084976888612,
-0.472186969216991));
#82273=CARTESIAN_POINT('',(-0.195399955328571,-0.000132127182848954,-0.402186969207341));
#82274=CARTESIAN_POINT('Ctrl Pts',(-0.195399940033293,0.000153084896563632,
-0.472186969212424));
#82275=CARTESIAN_POINT('Ctrl Pts',(-0.19540950022769,-0.0120496957420093,
-0.471493122787954));
#82276=CARTESIAN_POINT('Ctrl Pts',(-0.19427161528297,-0.0242672138561955,
-0.470799276363485));
#82277=CARTESIAN_POINT('Ctrl Pts',(-0.192004361224299,-0.0362696191164001,
-0.470105429939015));
#82278=CARTESIAN_POINT('Ctrl Pts',(-0.189737689439945,-0.0482689419287917,
-0.469411761707611));
#82279=CARTESIAN_POINT('Ctrl Pts',(-0.186342403735455,-0.0600524012197707,
-0.468718093476208));
#82280=CARTESIAN_POINT('Ctrl Pts',(-0.18188770489363,-0.0714004398342741,
-0.468024425244804));
#82281=CARTESIAN_POINT('Ctrl Pts',(-0.177421977072317,-0.0827765740147284,
-0.467329039623973));
#82282=CARTESIAN_POINT('Ctrl Pts',(-0.171891965994688,-0.0937143332632155,
-0.466633654003141));
#82283=CARTESIAN_POINT('Ctrl Pts',(-0.165414615592323,-0.104015214985328,
-0.46593826838231));
#82284=CARTESIAN_POINT('Ctrl Pts',(-0.161606433389355,-0.110071338556273,
-0.465529435297646));
#82285=CARTESIAN_POINT('Ctrl Pts',(-0.157471670309908,-0.115907817660625,
-0.465120602212981));
#82286=CARTESIAN_POINT('Ctrl Pts',(-0.153040690612817,-0.121489534597644,
-0.464711769128317));
#82287=CARTESIAN_POINT('Ctrl Pts',(-0.145489927268878,-0.131001251311659,
-0.464015083049728));
#82288=CARTESIAN_POINT('Ctrl Pts',(-0.137022523335021,-0.139839721180116,
-0.463318396971139));
#82289=CARTESIAN_POINT('Ctrl Pts',(-0.127782919780465,-0.147826538254737,
-0.462621710892551));
#82290=CARTESIAN_POINT('Ctrl Pts',(-0.118562594622314,-0.155796690867007,
-0.461926478446719));
#82291=CARTESIAN_POINT('Ctrl Pts',(-0.10857387499208,-0.162918095402392,
-0.461231246000888));
#82292=CARTESIAN_POINT('Ctrl Pts',(-0.0979981603981727,-0.169048870326228,
-0.460536013555057));
#82293=CARTESIAN_POINT('Ctrl Pts',(-0.0874239062865325,-0.175178798603914,
-0.459840877119254));
#82294=CARTESIAN_POINT('Ctrl Pts',(-0.0762635512230363,-0.180317891469279,
-0.459145740683451));
#82295=CARTESIAN_POINT('Ctrl Pts',(-0.0647264025934293,-0.184368253252325,
-0.458450604247648));
#82296=CARTESIAN_POINT('Ctrl Pts',(-0.0531898524783568,-0.188418404914094,
-0.457755503873551));
#82297=CARTESIAN_POINT('Ctrl Pts',(-0.0412773821397646,-0.191379673306578,
-0.457060403499454));
#82298=CARTESIAN_POINT('Ctrl Pts',(-0.0292144432181752,-0.193203717116033,
-0.456365303125357));
#82299=CARTESIAN_POINT('Ctrl Pts',(-0.0171239455559803,-0.195031928098224,
-0.455668614739331));
#82300=CARTESIAN_POINT('Ctrl Pts',(-0.00488316729722413,-0.195717661728824,
-0.454971926353305));
#82301=CARTESIAN_POINT('Ctrl Pts',(0.00727754878625668,-0.195264429130509,
-0.454275237967279));
#82302=CARTESIAN_POINT('Ctrl Pts',(0.0110478094637903,-0.195123910674896,
-0.454059239434932));
#82303=CARTESIAN_POINT('Ctrl Pts',(0.01481040213799,-0.194874289892408,
-0.453843240902584));
#82304=CARTESIAN_POINT('Ctrl Pts',(0.0185585999625431,-0.19451667889266,
-0.453627242370237));
#82305=CARTESIAN_POINT('Ctrl Pts',(0.0306481137929486,-0.193363233068902,
-0.452930556291648));
#82306=CARTESIAN_POINT('Ctrl Pts',(0.0426721119260769,-0.191074358260331,
-0.452233870213059));
#82307=CARTESIAN_POINT('Ctrl Pts',(0.0544023049230485,-0.187674050467985,
-0.45153718413447));
#82308=CARTESIAN_POINT('Ctrl Pts',(0.0661080229185633,-0.184280837404446,
-0.450841951688638));
#82309=CARTESIAN_POINT('Ctrl Pts',(0.0775202999573865,-0.179780964606533,
-0.450146719242806));
#82310=CARTESIAN_POINT('Ctrl Pts',(0.0884213549394379,-0.174249315610346,
-0.449451486796974));
#82311=CARTESIAN_POINT('Ctrl Pts',(0.0993209045104476,-0.168718430522376,
-0.448756350361171));
#82312=CARTESIAN_POINT('Ctrl Pts',(0.109708572580216,-0.162156407001039,
-0.448061213925368));
#82313=CARTESIAN_POINT('Ctrl Pts',(0.119388273052745,-0.154685488192924,
-0.447366077489565));
#82314=CARTESIAN_POINT('Ctrl Pts',(0.129067471369876,-0.14721495695488,
-0.446670977115468));
#82315=CARTESIAN_POINT('Ctrl Pts',(0.138038098868157,-0.138836180054443,
-0.445975876741371));
#82316=CARTESIAN_POINT('Ctrl Pts',(0.146136840781684,-0.129711926076012,
-0.445280776367273));
#82317=CARTESIAN_POINT('Ctrl Pts',(0.154254084913376,-0.120566827015775,
-0.444584087981247));
#82318=CARTESIAN_POINT('Ctrl Pts',(0.161494935443626,-0.110673548156325,
-0.443887399595221));
#82319=CARTESIAN_POINT('Ctrl Pts',(0.16773690428218,-0.100227196617639,
-0.443190711209195));
#82320=CARTESIAN_POINT('Ctrl Pts',(0.169672139797977,-0.0969884507938373,
-0.442974712676849));
#82321=CARTESIAN_POINT('Ctrl Pts',(0.171511692433523,-0.0936967247621157,
-0.442758714144502));
#82322=CARTESIAN_POINT('Ctrl Pts',(0.173252831848573,-0.0903582661213127,
-0.442542715612156));
#82323=CARTESIAN_POINT('Ctrl Pts',(0.178868738485392,-0.079590333424156,
-0.441846029533567));
#82324=CARTESIAN_POINT('Ctrl Pts',(0.183496651492235,-0.0682590536996094,
-0.441149343454978));
#82325=CARTESIAN_POINT('Ctrl Pts',(0.187032382179265,-0.0565689669019102,
-0.440452657376389));
#82326=CARTESIAN_POINT('Ctrl Pts',(0.19056073557815,-0.0449032714242446,
-0.439757424930557));
#82327=CARTESIAN_POINT('Ctrl Pts',(0.193001108433104,-0.0328810626946885,
-0.439062192484725));
#82328=CARTESIAN_POINT('Ctrl Pts',(0.19429771520829,-0.0207257777860888,
-0.438366960038894));
#82329=CARTESIAN_POINT('Ctrl Pts',(0.195594142925012,-0.00857217149484689,
-0.437671823603091));
#82330=CARTESIAN_POINT('Ctrl Pts',(0.195746980373878,0.003713610585935,
-0.436976687167288));
#82331=CARTESIAN_POINT('Ctrl Pts',(0.194751977890278,0.0159005379728084,
-0.436281550731485));
#82332=CARTESIAN_POINT('Ctrl Pts',(0.193757027024584,0.0280868331364667,
-0.435586450357388));
#82333=CARTESIAN_POINT('Ctrl Pts',(0.191614452601334,0.0401734139143807,
-0.434891349983291));
#82334=CARTESIAN_POINT('Ctrl Pts',(0.188371840413358,0.0519346679905087,
-0.434196249609194));
#82335=CARTESIAN_POINT('Ctrl Pts',(0.185121820220687,0.0637227915842889,
-0.433499561223168));
#82336=CARTESIAN_POINT('Ctrl Pts',(0.180767040576033,0.0751832792370354,
-0.432802872837142));
#82337=CARTESIAN_POINT('Ctrl Pts',(0.175404442670033,0.0861071512222719,
-0.432106184451116));
#82338=CARTESIAN_POINT('Ctrl Pts',(0.173741843866187,0.0894939456108076,
-0.431890185918769));
#82339=CARTESIAN_POINT('Ctrl Pts',(0.171982704995381,0.0928293383313204,
-0.431674187386423));
#82340=CARTESIAN_POINT('Ctrl Pts',(0.170130779294777,0.0961076372436237,
-0.431458188854077));
#82341=CARTESIAN_POINT('Ctrl Pts',(0.164157540309418,0.106681529523558,
-0.430761502775488));
#82342=CARTESIAN_POINT('Ctrl Pts',(0.157173794755142,0.116733533156061,
-0.430064816696899));
#82343=CARTESIAN_POINT('Ctrl Pts',(0.149294360337056,0.126064880008468,
-0.42936813061831));
#82344=CARTESIAN_POINT('Ctrl Pts',(0.141431366327829,0.135376757042442,
-0.428672898172479));
#82345=CARTESIAN_POINT('Ctrl Pts',(0.13267689542265,0.143970252348691,-0.427977665726647));
#82346=CARTESIAN_POINT('Ctrl Pts',(0.123187972784648,0.151676904508263,
-0.427282433280815));
#82347=CARTESIAN_POINT('Ctrl Pts',(0.113700360545405,0.159382492396599,
-0.426587296845013));
#82348=CARTESIAN_POINT('Ctrl Pts',(0.103479147494276,0.166200894290413,
-0.42589216040921));
#82349=CARTESIAN_POINT('Ctrl Pts',(0.0927157914244005,0.172002738410024,
-0.425197023973407));
#82350=CARTESIAN_POINT('Ctrl Pts',(0.0819529937268978,0.177804281546424,
-0.42450192359931));
#82351=CARTESIAN_POINT('Ctrl Pts',(0.0706488918858232,0.182588980244017,
-0.423806823225213));
#82352=CARTESIAN_POINT('Ctrl Pts',(0.0590186262771717,0.186273889078302,
-0.423111722851116));
#82353=CARTESIAN_POINT('Ctrl Pts',(0.0473617904044113,0.189967216379047,
-0.42241503446509));
#82354=CARTESIAN_POINT('Ctrl Pts',(0.0353781563987997,0.19255553610653,
-0.421718346079064));
#82355=CARTESIAN_POINT('Ctrl Pts',(0.0232957908446915,0.194006355898255,
-0.421021657693038));
#82356=CARTESIAN_POINT('Ctrl Pts',(0.0195498216577193,0.194456162371277,
-0.420805659160691));
#82357=CARTESIAN_POINT('Ctrl Pts',(0.0157943937200415,0.194797007162778,
-0.420589660628343));
#82358=CARTESIAN_POINT('Ctrl Pts',(0.0120363250164336,0.195028938570918,
-0.420373662095996));
#82359=CARTESIAN_POINT('Ctrl Pts',(-8.50265489191378E-5,0.195777014872558,
-0.419676976017407));
#82360=CARTESIAN_POINT('Ctrl Pts',(-0.01231892555592,0.19539335606406,-0.418980289938818));
#82361=CARTESIAN_POINT('Ctrl Pts',(-0.0244361355376008,0.193866024047506,
-0.418283603860229));
#82362=CARTESIAN_POINT('Ctrl Pts',(-0.0365280630084035,0.192341878803185,
-0.417588371414398));
#82363=CARTESIAN_POINT('Ctrl Pts',(-0.048502915982378,0.189678831927933,
-0.416893138968566));
#82364=CARTESIAN_POINT('Ctrl Pts',(-0.0601338930722158,0.185916849435384,
-0.416197906522735));
#82365=CARTESIAN_POINT('Ctrl Pts',(-0.0717632639504217,0.18215538646411,
-0.415502770086932));
#82366=CARTESIAN_POINT('Ctrl Pts',(-0.0830480080197834,0.177295514870008,
-0.414807633651129));
#82367=CARTESIAN_POINT('Ctrl Pts',(-0.0937753592425063,0.17142736654029,
-0.414112497215327));
#82368=CARTESIAN_POINT('Ctrl Pts',(-0.104502153960684,0.165559522633457,
-0.41341739684123));
#82369=CARTESIAN_POINT('Ctrl Pts',(-0.114670858589535,0.158683949476888,
-0.412722296467133));
#82370=CARTESIAN_POINT('Ctrl Pts',(-0.124094749885975,0.150935923658807,
-0.412027196093036));
#82371=CARTESIAN_POINT('Ctrl Pts',(-0.133540170809439,0.143170196861291,
-0.41133050770701));
#82372=CARTESIAN_POINT('Ctrl Pts',(-0.14223674759943,0.134528644042031,
-0.410633819320984));
#82373=CARTESIAN_POINT('Ctrl Pts',(-0.15003303449803,0.125184857547999,
-0.409937130934958));
#82374=CARTESIAN_POINT('Ctrl Pts',(-0.15245016468368,0.122287946662505,
-0.409721132402611));
#82375=CARTESIAN_POINT('Ctrl Pts',(-0.15478105631248,0.11932376745373,-0.409505133870263));
#82376=CARTESIAN_POINT('Ctrl Pts',(-0.15702203716539,0.116298064663308,
-0.409289135337916));
#82377=CARTESIAN_POINT('Ctrl Pts',(-0.164283431344131,0.106493955627549,
-0.40858924069876));
#82378=CARTESIAN_POINT('Ctrl Pts',(-0.170648781995794,0.0959725610274841,
-0.407889346059604));
#82379=CARTESIAN_POINT('Ctrl Pts',(-0.175981797535575,0.0849209452146396,
-0.407189451420448));
#82380=CARTESIAN_POINT('Ctrl Pts',(-0.18130290098295,0.0738940148481088,
-0.406491120101247));
#82381=CARTESIAN_POINT('Ctrl Pts',(-0.185595803747284,0.0623399493630731,
-0.405792788782047));
#82382=CARTESIAN_POINT('Ctrl Pts',(-0.188768944226097,0.0504722269744916,
-0.405094457462846));
#82383=CARTESIAN_POINT('Ctrl Pts',(-0.191939372373936,0.0386146488550512,
-0.40439672306196));
#82384=CARTESIAN_POINT('Ctrl Pts',(-0.193991676483236,0.026444767287892,
-0.403698988661075));
#82385=CARTESIAN_POINT('Ctrl Pts',(-0.194883961543337,0.0141916007967856,
-0.403001254260189));
#82386=CARTESIAN_POINT('Ctrl Pts',(-0.195231072794582,0.00942494926059903,
-0.402729825910934));
#82387=CARTESIAN_POINT('Ctrl Pts',(-0.195403186105232,0.00464579988061832,
-0.402458397561678));
#82388=CARTESIAN_POINT('Ctrl Pts',(-0.195399955328631,-0.000132127093388512,
-0.402186969212423));
#82389=CARTESIAN_POINT('',(-0.195399993177235,-5.16365805523595E-5,-0.332186969215685));
#82390=CARTESIAN_POINT('Ctrl Pts',(-0.195399955328571,-0.000132127182848178,
-0.402186969207341));
#82391=CARTESIAN_POINT('Ctrl Pts',(-0.195390495806332,-0.0141216044664258,
-0.401392243639799));
#82392=CARTESIAN_POINT('Ctrl Pts',(-0.193874546778018,-0.0280515508001564,
-0.400597518072257));
#82393=CARTESIAN_POINT('Ctrl Pts',(-0.190914403766276,-0.0416275201587533,
-0.399802792504715));
#82394=CARTESIAN_POINT('Ctrl Pts',(-0.188930132645979,-0.0507278926142205,
-0.399270064529755));
#82395=CARTESIAN_POINT('Ctrl Pts',(-0.186297990982151,-0.0596695466865476,
-0.398737336554796));
#82396=CARTESIAN_POINT('Ctrl Pts',(-0.183048772006924,-0.0683689042383835,
-0.398204608579836));
#82397=CARTESIAN_POINT('Ctrl Pts',(-0.178799538377885,-0.079745669837172,
-0.397507922501247));
#82398=CARTESIAN_POINT('Ctrl Pts',(-0.173470712728011,-0.0907647031971384,
-0.396811236422658));
#82399=CARTESIAN_POINT('Ctrl Pts',(-0.167144673837974,-0.101211748367456,
-0.396114550344069));
#82400=CARTESIAN_POINT('Ctrl Pts',(-0.160831834203152,-0.111636995819194,
-0.395419317898238));
#82401=CARTESIAN_POINT('Ctrl Pts',(-0.153526296825704,-0.121491844678251,
-0.394724085452406));
#82402=CARTESIAN_POINT('Ctrl Pts',(-0.145356861814906,-0.13058538479984,
-0.394028853006575));
#82403=CARTESIAN_POINT('Ctrl Pts',(-0.137188554984605,-0.139677669124106,
-0.393333716570772));
#82404=CARTESIAN_POINT('Ctrl Pts',(-0.128157137483981,-0.1480081732236,
-0.392638580134969));
#82405=CARTESIAN_POINT('Ctrl Pts',(-0.118431522417887,-0.155419221777043,
-0.391943443699166));
#82406=CARTESIAN_POINT('Ctrl Pts',(-0.108706411889108,-0.162829885866313,
-0.391248343325069));
#82407=CARTESIAN_POINT('Ctrl Pts',(-0.0982878876309854,-0.169320680297132,
-0.390553242950972));
#82408=CARTESIAN_POINT('Ctrl Pts',(-0.0873755028942675,-0.174776089594583,
-0.389858142576875));
#82409=CARTESIAN_POINT('Ctrl Pts',(-0.0764381879492221,-0.180243962207211,
-0.389161454190848));
#82410=CARTESIAN_POINT('Ctrl Pts',(-0.0650055713650576,-0.184671394988378,
-0.388464765804822));
#82411=CARTESIAN_POINT('Ctrl Pts',(-0.0532978506901253,-0.187990688896586,
-0.387768077418796));
#82412=CARTESIAN_POINT('Ctrl Pts',(-0.0496680349308383,-0.189019789749967,
-0.38755207888645));
#82413=CARTESIAN_POINT('Ctrl Pts',(-0.046011865622575,-0.189942741620966,
-0.387336080354103));
#82414=CARTESIAN_POINT('Ctrl Pts',(-0.0423360846919803,-0.190758527811874,
-0.387120081821756));
#82415=CARTESIAN_POINT('Ctrl Pts',(-0.0304801457906265,-0.193389781256677,
-0.386423395743169));
#82416=CARTESIAN_POINT('Ctrl Pts',(-0.0183363562956327,-0.194920746865561,
-0.385726709664581));
#82417=CARTESIAN_POINT('Ctrl Pts',(-0.00612927816464614,-0.195303845198143,
-0.385030023585993));
#82418=CARTESIAN_POINT('Ctrl Pts',(0.00605232994592505,-0.195686144197565,
-0.384334791140163));
#82419=CARTESIAN_POINT('Ctrl Pts',(0.0182961010228765,-0.194925228812739,
-0.383639558694332));
#82420=CARTESIAN_POINT('Ctrl Pts',(0.0303717752139235,-0.193025167453249,
-0.382944326248502));
#82421=CARTESIAN_POINT('Ctrl Pts',(0.0424457817816759,-0.191125368487935,
-0.3822491898127));
#82422=CARTESIAN_POINT('Ctrl Pts',(0.0543508674734123,-0.188086826848566,
-0.381554053376898));
#82423=CARTESIAN_POINT('Ctrl Pts',(0.0658628039446593,-0.183965352869901,
-0.380858916941096));
#82424=CARTESIAN_POINT('Ctrl Pts',(0.0773741432093051,-0.179844092701613,
-0.380163816567));
#82425=CARTESIAN_POINT('Ctrl Pts',(0.0884915590880914,-0.174640332115474,
-0.379468716192904));
#82426=CARTESIAN_POINT('Ctrl Pts',(0.0990094988516552,-0.168458538332564,
-0.378773615818808));
#82427=CARTESIAN_POINT('Ctrl Pts',(0.109551467682724,-0.162262621751516,
-0.378076927432783));
#82428=CARTESIAN_POINT('Ctrl Pts',(0.119490505659969,-0.155084710698945,
-0.377380239046758));
#82429=CARTESIAN_POINT('Ctrl Pts',(0.128649923243319,-0.14707262576526,
-0.376683550660733));
#82430=CARTESIAN_POINT('Ctrl Pts',(0.131489673115562,-0.144588590403863,
-0.376467552128381));
#82431=CARTESIAN_POINT('Ctrl Pts',(0.134254743571772,-0.142024648216559,
-0.376251553596028));
#82432=CARTESIAN_POINT('Ctrl Pts',(0.136940610567483,-0.139385900210189,
-0.376035555063675));
#82433=CARTESIAN_POINT('Ctrl Pts',(0.145603660841381,-0.130874828487042,
-0.375338868985085));
#82434=CARTESIAN_POINT('Ctrl Pts',(0.153500616710919,-0.121523167298244,
-0.374642182906494));
#82435=CARTESIAN_POINT('Ctrl Pts',(0.160469286891498,-0.111493353902975,
-0.373945496827903));
#82436=CARTESIAN_POINT('Ctrl Pts',(0.167423416969206,-0.101484467673832,
-0.37325026438207));
#82437=CARTESIAN_POINT('Ctrl Pts',(0.173452550890537,-0.0908009070984694,
-0.372555031936237));
#82438=CARTESIAN_POINT('Ctrl Pts',(0.178434713131651,-0.0796380132199777,
-0.371859799490404));
#82439=CARTESIAN_POINT('Ctrl Pts',(0.183416187347428,-0.0684766609118829,
-0.371164663054599));
#82440=CARTESIAN_POINT('Ctrl Pts',(0.187350579439717,-0.0568368860220045,
-0.370469526618794));
#82441=CARTESIAN_POINT('Ctrl Pts',(0.190162595785668,-0.044937146817044,
-0.369774390182989));
#82442=CARTESIAN_POINT('Ctrl Pts',(0.19297446625219,-0.0330380249367914,
-0.369079289808891));
#82443=CARTESIAN_POINT('Ctrl Pts',(0.194663901666248,-0.0208798232588043,
-0.368384189434792));
#82444=CARTESIAN_POINT('Ctrl Pts',(0.195206588133133,-0.00869183233969888,
-0.367689089060693));
#82445=CARTESIAN_POINT('Ctrl Pts',(0.195750514410289,0.00352400301121695,
-0.366992400674666));
#82446=CARTESIAN_POINT('Ctrl Pts',(0.19514248802952,0.0157688871230913,
-0.366295712288638));
#82447=CARTESIAN_POINT('Ctrl Pts',(0.193410274246544,0.0278141297882296,
-0.36559902390261));
#82448=CARTESIAN_POINT('Ctrl Pts',(0.192873225485115,0.0315485895402594,
-0.365383025370272));
#82449=CARTESIAN_POINT('Ctrl Pts',(0.192228489943372,0.0352639267049012,
-0.365167026837934));
#82450=CARTESIAN_POINT('Ctrl Pts',(0.191477882418444,0.0389535690861376,
-0.364951028305596));
#82451=CARTESIAN_POINT('Ctrl Pts',(0.189056857574245,0.050854216994026,
-0.364254342227008));
#82452=CARTESIAN_POINT('Ctrl Pts',(0.185513629958333,0.0625700616949622,
-0.363557656148419));
#82453=CARTESIAN_POINT('Ctrl Pts',(0.180896119262338,0.07387661359203,-0.362860970069831));
#82454=CARTESIAN_POINT('Ctrl Pts',(0.176288242984212,0.0851595744131221,
-0.362165737624));
#82455=CARTESIAN_POINT('Ctrl Pts',(0.170610791920237,0.0960341075904182,
-0.361470505178169));
#82456=CARTESIAN_POINT('Ctrl Pts',(0.163961182576747,0.106291535919068,
-0.360775272732339));
#82457=CARTESIAN_POINT('Ctrl Pts',(0.157312491529268,0.116547547720066,
-0.360080136296536));
#82458=CARTESIAN_POINT('Ctrl Pts',(0.149692345908798,0.12618586610788,-0.359384999860733));
#82459=CARTESIAN_POINT('Ctrl Pts',(0.141242971896812,0.135024378871952,
-0.358689863424931));
#82460=CARTESIAN_POINT('Ctrl Pts',(0.132794036214376,0.143862433119059,
-0.357994763050834));
#82461=CARTESIAN_POINT('Ctrl Pts',(0.123516581715587,0.151900150337455,
-0.357299662676738));
#82462=CARTESIAN_POINT('Ctrl Pts',(0.113589680906363,0.158992277773452,
-0.356604562302641));
#82463=CARTESIAN_POINT('Ctrl Pts',(0.103640101304996,0.166100607737013,
-0.355907873916616));
#82464=CARTESIAN_POINT('Ctrl Pts',(0.0930388627788211,0.172258580187678,
-0.35521118553059));
#82465=CARTESIAN_POINT('Ctrl Pts',(0.0819928939630575,0.177364949580132,
-0.354514497144565));
#82466=CARTESIAN_POINT('Ctrl Pts',(0.0785682451524217,0.178948108301491,
-0.354298498612215));
#82467=CARTESIAN_POINT('Ctrl Pts',(0.0751009942593462,0.180430533817913,
-0.354082500079865));
#82468=CARTESIAN_POINT('Ctrl Pts',(0.0715976418209153,0.181810169368173,
-0.353866501547515));
#82469=CARTESIAN_POINT('Ctrl Pts',(0.0602978573007469,0.186260074054694,
-0.353169815468932));
#82470=CARTESIAN_POINT('Ctrl Pts',(0.0485419779593049,0.189668120401466,
-0.352473129390349));
#82471=CARTESIAN_POINT('Ctrl Pts',(0.0365443843399179,0.191952254410352,
-0.351776443311766));
#82472=CARTESIAN_POINT('Ctrl Pts',(0.0245718236523404,0.194231622582629,
-0.351081210865941));
#82473=CARTESIAN_POINT('Ctrl Pts',(0.0123593869498785,0.19539149852171,
-0.350385978420115));
#82474=CARTESIAN_POINT('Ctrl Pts',(0.000135145916032145,0.19539995326402,
-0.34969074597429));
#82475=CARTESIAN_POINT('Ctrl Pts',(-0.012087406977776,0.19540840683875,
-0.348995609538493));
#82476=CARTESIAN_POINT('Ctrl Pts',(-0.0243208873540597,0.194265708933368,
-0.348300473102696));
#82477=CARTESIAN_POINT('Ctrl Pts',(-0.0363351032855113,0.191991979700276,
-0.347605336666898));
#82478=CARTESIAN_POINT('Ctrl Pts',(-0.0483486959535267,0.189718368421806,
-0.346910236292807));
#82479=CARTESIAN_POINT('Ctrl Pts',(-0.0601421920734194,0.186314031580679,
-0.346215135918716));
#82480=CARTESIAN_POINT('Ctrl Pts',(-0.0714962501735998,0.181850065194143,
-0.345520035544625));
#82481=CARTESIAN_POINT('Ctrl Pts',(-0.0828762475199363,0.177375900522385,
-0.344823347158605));
#82482=CARTESIAN_POINT('Ctrl Pts',(-0.0938140128905463,0.171837654257794,
-0.344126658772585));
#82483=CARTESIAN_POINT('Ctrl Pts',(-0.104111945898851,0.165353750248232,
-0.343429970386565));
#82484=CARTESIAN_POINT('Ctrl Pts',(-0.107304676624578,0.163343506101441,
-0.343213971854189));
#82485=CARTESIAN_POINT('Ctrl Pts',(-0.110436118429122,0.161242676171266,
-0.342997973321812));
#82486=CARTESIAN_POINT('Ctrl Pts',(-0.113501006385173,0.159055592638401,
-0.342781974789436));
#82487=CARTESIAN_POINT('Ctrl Pts',(-0.123318976184754,0.152049555098778,
-0.342090051594189));
#82488=CARTESIAN_POINT('Ctrl Pts',(-0.132522561191368,0.144104678485816,
-0.341398128398942));
#82489=CARTESIAN_POINT('Ctrl Pts',(-0.14092759677856,0.135353509249741,
-0.340706205203695));
#82490=CARTESIAN_POINT('Ctrl Pts',(-0.149551444308025,0.126374517023762,
-0.339996268871361));
#82491=CARTESIAN_POINT('Ctrl Pts',(-0.157333699405892,0.116547121797068,
-0.339286332539027));
#82492=CARTESIAN_POINT('Ctrl Pts',(-0.164112187289878,0.106058238637704,
-0.338576396206692));
#82493=CARTESIAN_POINT('Ctrl Pts',(-0.170703821381919,0.0958584889289168,
-0.337886029769297));
#82494=CARTESIAN_POINT('Ctrl Pts',(-0.176345925822205,0.0850341114372617,
-0.337195663331902));
#82495=CARTESIAN_POINT('Ctrl Pts',(-0.180932531280471,0.0737873913649312,
-0.336505296894507));
#82496=CARTESIAN_POINT('Ctrl Pts',(-0.18571416226884,0.0620624532370067,
-0.335785575614703));
#82497=CARTESIAN_POINT('Ctrl Pts',(-0.189347895449973,0.0498793191282996,
-0.3350658543349));
#82498=CARTESIAN_POINT('Ctrl Pts',(-0.191770197879697,0.0374880141536166,
-0.334346133055096));
#82499=CARTESIAN_POINT('Ctrl Pts',(-0.194192500309422,0.0250967091789336,
-0.333626411775292));
#82500=CARTESIAN_POINT('Ctrl Pts',(-0.195403309639771,0.0124983183140073,
-0.332906690495488));
#82501=CARTESIAN_POINT('Ctrl Pts',(-0.195399993177235,-5.16365805518149E-5,
-0.332186969215685));
#82502=CARTESIAN_POINT('',(-0.195399923138918,0.000173312737304163,-0.262186969217073));
#82503=CARTESIAN_POINT('Ctrl Pts',(-0.19539999317722,-5.16366374107664E-5,
-0.332186969212424));
#82504=CARTESIAN_POINT('Ctrl Pts',(-0.195399241274833,-0.0028969365771944,
-0.332023795485401));
#82505=CARTESIAN_POINT('Ctrl Pts',(-0.195336344993682,-0.00574133241449791,
-0.331860621758378));
#82506=CARTESIAN_POINT('Ctrl Pts',(-0.195211404501634,-0.00858298039724923,
-0.331697448031355));
#82507=CARTESIAN_POINT('Ctrl Pts',(-0.194677958933839,-0.0207156725035708,
-0.331000761952774));
#82508=CARTESIAN_POINT('Ctrl Pts',(-0.193007219482665,-0.0328410223409046,
-0.330304075874194));
#82509=CARTESIAN_POINT('Ctrl Pts',(-0.190211471622053,-0.0447298117967517,
-0.329607389795614));
#82510=CARTESIAN_POINT('Ctrl Pts',(-0.187421557078334,-0.0565937953402518,
-0.328912157349791));
#82511=CARTESIAN_POINT('Ctrl Pts',(-0.18351141975519,-0.0682213380092308,
-0.328216924903969));
#82512=CARTESIAN_POINT('Ctrl Pts',(-0.178544703623131,-0.0793911129039529,
-0.327521692458147));
#82513=CARTESIAN_POINT('Ctrl Pts',(-0.173578673383334,-0.0905593452780333,
-0.326826556022353));
#82514=CARTESIAN_POINT('Ctrl Pts',(-0.167556667527731,-0.101269118669381,
-0.32613141958656));
#82515=CARTESIAN_POINT('Ctrl Pts',(-0.160590737519437,-0.111318349893283,
-0.325436283150766));
#82516=CARTESIAN_POINT('Ctrl Pts',(-0.153625168883825,-0.121367059791584,
-0.324741182776679));
#82517=CARTESIAN_POINT('Ctrl Pts',(-0.145716294008896,-0.130754591856478,
-0.324046082402591));
#82518=CARTESIAN_POINT('Ctrl Pts',(-0.137018313282915,-0.139309518070751,
-0.323350982028503));
#82519=CARTESIAN_POINT('Ctrl Pts',(-0.128300461330176,-0.147883988692406,
-0.322654293642487));
#82520=CARTESIAN_POINT('Ctrl Pts',(-0.11879057371783,-0.155621489618999,
-0.32195760525647));
#82521=CARTESIAN_POINT('Ctrl Pts',(-0.108677235682741,-0.162389711633335,
-0.321260916870453));
#82522=CARTESIAN_POINT('Ctrl Pts',(-0.105541736057656,-0.164488104618403,
-0.321044918338061));
#82523=CARTESIAN_POINT('Ctrl Pts',(-0.102348430542222,-0.166493650443819,
-0.32082891980567));
#82524=CARTESIAN_POINT('Ctrl Pts',(-0.099103418872104,-0.168403302722543,
-0.320612921273278));
#82525=CARTESIAN_POINT('Ctrl Pts',(-0.0886368919457939,-0.174562734190601,
-0.319916235194723));
#82526=CARTESIAN_POINT('Ctrl Pts',(-0.0775572107272582,-0.179764286177824,
-0.319219549116168));
#82527=CARTESIAN_POINT('Ctrl Pts',(-0.0660633171180524,-0.183893442328321,
-0.318522863037613));
#82528=CARTESIAN_POINT('Ctrl Pts',(-0.0545934054725746,-0.18801398301078,
-0.317827630591816));
#82529=CARTESIAN_POINT('Ctrl Pts',(-0.0427117872134389,-0.19106620678016,
-0.317132398146018));
#82530=CARTESIAN_POINT('Ctrl Pts',(-0.0306387528817784,-0.192982970289736,
-0.316437165700221));
#82531=CARTESIAN_POINT('Ctrl Pts',(-0.0185673858088527,-0.194899469098607,
-0.315742029264451));
#82532=CARTESIAN_POINT('Ctrl Pts',(-0.00630551086825178,-0.195680637166155,
-0.315046892828682));
#82533=CARTESIAN_POINT('Ctrl Pts',(0.00591636139793886,-0.19531041105842,
-0.314351756392912));
#82534=CARTESIAN_POINT('Ctrl Pts',(0.0181375996280714,-0.194940204156965,
-0.313656656018849));
#82535=CARTESIAN_POINT('Ctrl Pts',(0.0303179655481477,-0.193418775190653,
-0.312961555644785));
#82536=CARTESIAN_POINT('Ctrl Pts',(0.0422297078280292,-0.190782105494093,
-0.312266455270722));
#82537=CARTESIAN_POINT('Ctrl Pts',(0.0541686634278107,-0.18813941211651,
-0.311569766884729));
#82538=CARTESIAN_POINT('Ctrl Pts',(0.0658369307298061,-0.184376644365591,
-0.310873078498736));
#82539=CARTESIAN_POINT('Ctrl Pts',(0.0770208442306797,-0.179579925253335,
-0.310176390112744));
#82540=CARTESIAN_POINT('Ctrl Pts',(0.0804882608728209,-0.178092769288098,
-0.309960391580227));
#82541=CARTESIAN_POINT('Ctrl Pts',(0.0839092820691905,-0.176506570005805,
-0.309744393047711));
#82542=CARTESIAN_POINT('Ctrl Pts',(0.0872780311207803,-0.174824784523477,
-0.309528394515195));
#82543=CARTESIAN_POINT('Ctrl Pts',(0.0981436631207327,-0.169400319277181,
-0.308831708436502));
#82544=CARTESIAN_POINT('Ctrl Pts',(0.108539786586155,-0.16293997130447,
-0.30813502235781));
#82545=CARTESIAN_POINT('Ctrl Pts',(0.118262019687355,-0.15554823913972,
-0.307438336279117));
#82546=CARTESIAN_POINT('Ctrl Pts',(0.127963967387505,-0.148171929795002,
-0.306743103833182));
#82547=CARTESIAN_POINT('Ctrl Pts',(0.136994081315752,-0.139868559100433,
-0.306047871387248));
#82548=CARTESIAN_POINT('Ctrl Pts',(0.145176087370112,-0.130786328245369,
-0.305352638941313));
#82549=CARTESIAN_POINT('Ctrl Pts',(0.153356963507925,-0.121705351625864,
-0.304657502505408));
#82550=CARTESIAN_POINT('Ctrl Pts',(0.160689345840531,-0.111846347112711,
-0.303962366069503));
#82551=CARTESIAN_POINT('Ctrl Pts',(0.167034237172029,-0.101393903230709,
-0.303267229633599));
#82552=CARTESIAN_POINT('Ctrl Pts',(0.173378799348559,-0.0909420015918515,
-0.302572129259401));
#82553=CARTESIAN_POINT('Ctrl Pts',(0.178735541318582,-0.0798974836952926,
-0.301877028885203));
#82554=CARTESIAN_POINT('Ctrl Pts',(0.183010619864622,-0.0684709647716965,
-0.301181928511005));
#82555=CARTESIAN_POINT('Ctrl Pts',(0.187295465166611,-0.057018341059503,
-0.300485240124881));
#82556=CARTESIAN_POINT('Ctrl Pts',(0.190493468620826,-0.0451828158518389,
-0.299788551738757));
#82557=CARTESIAN_POINT('Ctrl Pts',(0.192560512709603,-0.0331904947991887,
-0.299091863352634));
#82558=CARTESIAN_POINT('Ctrl Pts',(0.19320137094309,-0.029472442665253,
-0.298875864820794));
#82559=CARTESIAN_POINT('Ctrl Pts',(0.193733894081805,-0.0257393697745842,
-0.298659866288955));
#82560=CARTESIAN_POINT('Ctrl Pts',(0.194157781558028,-0.0219980876547268,
-0.298443867757116));
#82561=CARTESIAN_POINT('Ctrl Pts',(0.195524996885923,-0.00993087985273009,
-0.29774718167862));
#82562=CARTESIAN_POINT('Ctrl Pts',(0.195767716935638,0.0023066266717942,
-0.297050495600125));
#82563=CARTESIAN_POINT('Ctrl Pts',(0.194862291688264,0.014486106378107,
-0.296353809521629));
#82564=CARTESIAN_POINT('Ctrl Pts',(0.1939587556071,0.0266401736480271,-0.29565857707589));
#82565=CARTESIAN_POINT('Ctrl Pts',(0.191911819837225,0.0387355850229386,
-0.29496334463015));
#82566=CARTESIAN_POINT('Ctrl Pts',(0.188749795080135,0.050543791480331,
-0.29426811218441));
#82567=CARTESIAN_POINT('Ctrl Pts',(0.185588206991497,0.0623503672511719,
-0.293572975748696));
#82568=CARTESIAN_POINT('Ctrl Pts',(0.181312017803303,0.0738689612024969,
-0.292877839312982));
#82569=CARTESIAN_POINT('Ctrl Pts',(0.176000356436181,0.0848824748363132,
-0.292182702877267));
#82570=CARTESIAN_POINT('Ctrl Pts',(0.170688970622967,0.0958954171203168,
-0.291487602503257));
#82571=CARTESIAN_POINT('Ctrl Pts',(0.164342623729396,0.106402554748214,
-0.290792502129247));
#82572=CARTESIAN_POINT('Ctrl Pts',(0.157086862589102,0.116210488347277,
-0.290097401755237));
#82573=CARTESIAN_POINT('Ctrl Pts',(0.149814525087026,0.126040828948517,
-0.289400713369294));
#82574=CARTESIAN_POINT('Ctrl Pts',(0.141629198182814,0.135168112576547,
-0.288704024983351));
#82575=CARTESIAN_POINT('Ctrl Pts',(0.132696499062621,0.143432210944836,
-0.288007336597408));
#82576=CARTESIAN_POINT('Ctrl Pts',(0.129927040086767,0.145994379567717,
-0.287791338064617));
#82577=CARTESIAN_POINT('Ctrl Pts',(0.127085988979078,0.148473863955332,
-0.287575339531826));
#82578=CARTESIAN_POINT('Ctrl Pts',(0.124178895090764,0.150866702800973,
-0.287359340999035));
#82579=CARTESIAN_POINT('Ctrl Pts',(0.114802295099811,0.158584614076071,
-0.286662654920628));
#82580=CARTESIAN_POINT('Ctrl Pts',(0.104670517652445,0.165452114689179,
-0.285965968842221));
#82581=CARTESIAN_POINT('Ctrl Pts',(0.0939621873808109,0.17132503419703,
-0.285269282763813));
#82582=CARTESIAN_POINT('Ctrl Pts',(0.0832761999981347,0.177185699881446,
-0.284574050318166));
#82583=CARTESIAN_POINT('Ctrl Pts',(0.0720167716332992,0.182055422176276,
-0.283878817872519));
#82584=CARTESIAN_POINT('Ctrl Pts',(0.0603910095274079,0.185833489899589,
-0.283183585426872));
#82585=CARTESIAN_POINT('Ctrl Pts',(0.0487668529129842,0.189611035880289,
-0.282488448991254));
#82586=CARTESIAN_POINT('Ctrl Pts',(0.0367772798465013,0.192296913433613,
-0.281793312555636));
#82587=CARTESIAN_POINT('Ctrl Pts',(0.0246474667033551,0.193839269460827,
-0.281098176120018));
#82588=CARTESIAN_POINT('Ctrl Pts',(0.0125182828205135,0.195381545474984,
-0.280403075746107));
#82589=CARTESIAN_POINT('Ctrl Pts',(0.000249744703043385,0.195780334198186,
-0.279707975372196));
#82590=CARTESIAN_POINT('Ctrl Pts',(-0.0119275715780176,0.195035619916597,
-0.279012874998285));
#82591=CARTESIAN_POINT('Ctrl Pts',(-0.0241327079038838,0.194289204276169,
-0.278316186612442));
#82592=CARTESIAN_POINT('Ctrl Pts',(-0.0362453376655141,0.192394188927021,
-0.2776194982266));
#82593=CARTESIAN_POINT('Ctrl Pts',(-0.0480409699354846,0.189402284061354,
-0.276922809840757));
#82594=CARTESIAN_POINT('Ctrl Pts',(-0.0516980414771468,0.188474685617356,
-0.27670681130749));
#82595=CARTESIAN_POINT('Ctrl Pts',(-0.0553247487980788,0.187442015148976,
-0.276490812774223));
#82596=CARTESIAN_POINT('Ctrl Pts',(-0.058914747541078,0.18630676993113,
-0.276274814240956));
#82597=CARTESIAN_POINT('Ctrl Pts',(-0.0704940027847687,0.182645126826868,
-0.275578128161653));
#82598=CARTESIAN_POINT('Ctrl Pts',(-0.0817712252968662,0.177887004119356,
-0.27488144208235));
#82599=CARTESIAN_POINT('Ctrl Pts',(-0.0925282252597426,0.172103711552896,
-0.274184756003048));
#82600=CARTESIAN_POINT('Ctrl Pts',(-0.103262780784625,0.166332485803565,
-0.273489523556501));
#82601=CARTESIAN_POINT('Ctrl Pts',(-0.113478470266465,0.159540681102335,
-0.272794291109955));
#82602=CARTESIAN_POINT('Ctrl Pts',(-0.122978044244706,0.151847162086577,
-0.272099058663409));
#82603=CARTESIAN_POINT('Ctrl Pts',(-0.132476306353136,0.144154705528499,
-0.271403922226901));
#82604=CARTESIAN_POINT('Ctrl Pts',(-0.141257941827696,0.135561296467514,
-0.270708785790392));
#82605=CARTESIAN_POINT('Ctrl Pts',(-0.149156840362037,0.126227560275931,
-0.270013649353884));
#82606=CARTESIAN_POINT('Ctrl Pts',(-0.157055329123879,0.116894308292164,
-0.269318548979086));
#82607=CARTESIAN_POINT('Ctrl Pts',(-0.164070627274964,0.106821490801852,
-0.268623448604289));
#82608=CARTESIAN_POINT('Ctrl Pts',(-0.170077161622158,0.096202490064189,
-0.267928348229492));
#82609=CARTESIAN_POINT('Ctrl Pts',(-0.176097418373224,0.08555922937754,
-0.267231659842785));
#82610=CARTESIAN_POINT('Ctrl Pts',(-0.181103936970048,0.0743680875759282,
-0.266534971456079));
#82611=CARTESIAN_POINT('Ctrl Pts',(-0.185017841892093,0.0628455104330651,
-0.265838283069372));
#82612=CARTESIAN_POINT('Ctrl Pts',(-0.186231293589125,0.0592730959092883,
-0.26562228454054));
#82613=CARTESIAN_POINT('Ctrl Pts',(-0.187340083534537,0.0556689318504821,
-0.265406286011707));
#82614=CARTESIAN_POINT('Ctrl Pts',(-0.188342851450472,0.0520396993410366,
-0.265190287482875));
#82615=CARTESIAN_POINT('Ctrl Pts',(-0.192396085389066,0.0373701749729622,
-0.264317211516006));
#82616=CARTESIAN_POINT('Ctrl Pts',(-0.194736418589095,0.0222079032156958,
-0.263444135549137));
#82617=CARTESIAN_POINT('Ctrl Pts',(-0.195277763789369,0.00691049704604845,
-0.262571059582269));
#82618=CARTESIAN_POINT('Ctrl Pts',(-0.195357148052045,0.00466724577307081,
-0.262443029460537));
#82619=CARTESIAN_POINT('Ctrl Pts',(-0.195397929407478,0.00242112773447588,
-0.262314999338805));
#82620=CARTESIAN_POINT('Ctrl Pts',(-0.195399923138918,0.000173312737304944,
-0.262186969217073));
#82621=CARTESIAN_POINT('',(-0.195399980573749,-8.71308121574774E-5,-0.19218696920821));
#82622=CARTESIAN_POINT('Ctrl Pts',(-0.19539992313899,0.000173312655682386,
-0.262186969212424));
#82623=CARTESIAN_POINT('Ctrl Pts',(-0.195410653058069,-0.0119240460448848,
-0.2614979328331));
#82624=CARTESIAN_POINT('Ctrl Pts',(-0.194293610829215,-0.0240463379113419,
-0.260808896453775));
#82625=CARTESIAN_POINT('Ctrl Pts',(-0.192061369462662,-0.0359665172087442,
-0.260119860074451));
#82626=CARTESIAN_POINT('Ctrl Pts',(-0.189830801962487,-0.0478777580518912,
-0.259431340375287));
#82627=CARTESIAN_POINT('Ctrl Pts',(-0.186486850453256,-0.059586306886096,
-0.258742820676124));
#82628=CARTESIAN_POINT('Ctrl Pts',(-0.182093486969189,-0.0708739867892439,
-0.25805430097696));
#82629=CARTESIAN_POINT('Ctrl Pts',(-0.177689492763121,-0.0821889797493508,
-0.257364115250949));
#82630=CARTESIAN_POINT('Ctrl Pts',(-0.172231359849049,-0.093080239188824,
-0.256673929524939));
#82631=CARTESIAN_POINT('Ctrl Pts',(-0.165831481543612,-0.103349309281923,
-0.255983743798928));
#82632=CARTESIAN_POINT('Ctrl Pts',(-0.160026829896396,-0.112663294921408,
-0.255357749440884));
#82633=CARTESIAN_POINT('Ctrl Pts',(-0.153448374712411,-0.121465349160077,
-0.254731755082839));
#82634=CARTESIAN_POINT('Ctrl Pts',(-0.14620914768459,-0.129630417469612,
-0.254105760724795));
#82635=CARTESIAN_POINT('Ctrl Pts',(-0.138152415832565,-0.138717543162808,
-0.253409074647088));
#82636=CARTESIAN_POINT('Ctrl Pts',(-0.129217002484211,-0.147082581529689,
-0.252712388569381));
#82637=CARTESIAN_POINT('Ctrl Pts',(-0.119556834612108,-0.154555243513551,
-0.252015702491674));
#82638=CARTESIAN_POINT('Ctrl Pts',(-0.109916822642486,-0.162012313817412,
-0.251320470046744));
#82639=CARTESIAN_POINT('Ctrl Pts',(-0.0995556977450317,-0.168580115038724,
-0.250625237601813));
#82640=CARTESIAN_POINT('Ctrl Pts',(-0.0886623049952405,-0.174126837888164,
-0.249930005156882));
#82641=CARTESIAN_POINT('Ctrl Pts',(-0.0777704165985586,-0.179672794747617,
-0.249234868721993));
#82642=CARTESIAN_POINT('Ctrl Pts',(-0.0663471642281377,-0.184197516344812,
-0.248539732287103));
#82643=CARTESIAN_POINT('Ctrl Pts',(-0.0546068681200209,-0.18761463150331,
-0.247844595852214));
#82644=CARTESIAN_POINT('Ctrl Pts',(-0.0428671810652999,-0.191031569391526,
-0.247149495479039));
#82645=CARTESIAN_POINT('Ctrl Pts',(-0.0308113305979205,-0.193340796361407,
-0.246454395105865));
#82646=CARTESIAN_POINT('Ctrl Pts',(-0.0186670631411277,-0.194506300035976,
-0.24575929473269));
#82647=CARTESIAN_POINT('Ctrl Pts',(-0.00649505114212026,-0.19567446639613,
-0.245062606347582));
#82648=CARTESIAN_POINT('Ctrl Pts',(0.00576490455346149,-0.195693674682041,
-0.244365917962473));
#82649=CARTESIAN_POINT('Ctrl Pts',(0.0178829927575548,-0.194579954183449,
-0.243669229577365));
#82650=CARTESIAN_POINT('Ctrl Pts',(0.0216400373385423,-0.194234660644279,
-0.243453231040481));
#82651=CARTESIAN_POINT('Ctrl Pts',(0.0253834935417705,-0.193780843038646,
-0.243237232503598));
#82652=CARTESIAN_POINT('Ctrl Pts',(0.0291067049334456,-0.193219977559044,
-0.243021233966715));
#82653=CARTESIAN_POINT('Ctrl Pts',(0.041115626843582,-0.191410950609435,
-0.242324547883315));
#82654=CARTESIAN_POINT('Ctrl Pts',(0.0529973985326241,-0.188471736001752,
-0.241627861799915));
#82655=CARTESIAN_POINT('Ctrl Pts',(0.0645253728350063,-0.184438705971668,
-0.240931175716515));
#82656=CARTESIAN_POINT('Ctrl Pts',(0.0760292940647887,-0.180414090842725,
-0.240235943265861));
#82657=CARTESIAN_POINT('Ctrl Pts',(0.0871800410625355,-0.175300406681039,
-0.239540710815207));
#82658=CARTESIAN_POINT('Ctrl Pts',(0.0977642261316131,-0.169184266670654,
-0.238845478364553));
#82659=CARTESIAN_POINT('Ctrl Pts',(0.108346949547824,-0.16306897128586,
-0.238150341923984));
#82660=CARTESIAN_POINT('Ctrl Pts',(0.118362487240594,-0.155951892727064,
-0.237455205483415));
#82661=CARTESIAN_POINT('Ctrl Pts',(0.127621689294173,-0.147965754219352,
-0.236760069042845));
#82662=CARTESIAN_POINT('Ctrl Pts',(0.13688041100625,-0.139980030010166,
-0.23606496866401));
#82663=CARTESIAN_POINT('Ctrl Pts',(0.145382230068811,-0.131125927311856,
-0.235369868285175));
#82664=CARTESIAN_POINT('Ctrl Pts',(0.152972922727515,-0.121574853124327,
-0.23467476790634));
#82665=CARTESIAN_POINT('Ctrl Pts',(0.160580956924063,-0.112001958752276,
-0.233978079515703));
#82666=CARTESIAN_POINT('Ctrl Pts',(0.167273216425432,-0.101729639260994,
-0.233281391125066));
#82667=CARTESIAN_POINT('Ctrl Pts',(0.172938001961387,-0.0909593726759544,
-0.232584702734429));
#82668=CARTESIAN_POINT('Ctrl Pts',(0.174694289627061,-0.0876202018919485,
-0.232368704225831));
#82669=CARTESIAN_POINT('Ctrl Pts',(0.176352155506728,-0.0842333313931768,
-0.232152705717234));
#82670=CARTESIAN_POINT('Ctrl Pts',(0.177909212970956,-0.0808051479799098,
-0.231936707208636));
#82671=CARTESIAN_POINT('Ctrl Pts',(0.182931378426524,-0.0697478140606376,
-0.231240021136826));
#82672=CARTESIAN_POINT('Ctrl Pts',(0.186936383309858,-0.0581816819394014,
-0.230543335065016));
#82673=CARTESIAN_POINT('Ctrl Pts',(0.189831313534887,-0.0463166536099004,
-0.229846648993206));
#82674=CARTESIAN_POINT('Ctrl Pts',(0.192720203499534,-0.0344763816147428,
-0.22915141655411));
#82675=CARTESIAN_POINT('Ctrl Pts',(0.194503339078234,-0.0223392753961914,
-0.228456184115014));
#82676=CARTESIAN_POINT('Ctrl Pts',(0.195137165153437,-0.0101314745165962,
-0.227760951675918));
#82677=CARTESIAN_POINT('Ctrl Pts',(0.19577090369884,0.00207464049617775,
-0.227065815246685));
#82678=CARTESIAN_POINT('Ctrl Pts',(0.195255557244779,0.0143505606708363,
-0.226370678817453));
#82679=CARTESIAN_POINT('Ctrl Pts',(0.193599443161949,0.0264653661864563,
-0.225675542388221));
#82680=CARTESIAN_POINT('Ctrl Pts',(0.191943414993408,0.0385795432218813,
-0.224980442020606));
#82681=CARTESIAN_POINT('Ctrl Pts',(0.189146881990735,0.0505317589418535,
-0.224285341652991));
#82682=CARTESIAN_POINT('Ctrl Pts',(0.185269625737726,0.0620993218884295,
-0.223590241285376));
#82683=CARTESIAN_POINT('Ctrl Pts',(0.181383511583866,0.0736933118542674,
-0.222893552905585));
#82684=CARTESIAN_POINT('Ctrl Pts',(0.176412085024892,0.0849000865122645,
-0.222196864525794));
#82685=CARTESIAN_POINT('Ctrl Pts',(0.170463505756305,0.0955162457662059,
-0.221500176146003));
#82686=CARTESIAN_POINT('Ctrl Pts',(0.168619231294489,0.0988076386367702,
-0.221284177580853));
#82687=CARTESIAN_POINT('Ctrl Pts',(0.166681354149909,0.102042457122414,
-0.221068179015704));
#82688=CARTESIAN_POINT('Ctrl Pts',(0.164653931482825,0.105215221556813,
-0.220852180450555));
#82689=CARTESIAN_POINT('Ctrl Pts',(0.15811464202164,0.115448719172049,-0.22015549437535));
#82690=CARTESIAN_POINT('Ctrl Pts',(0.150594714827337,0.125106160460965,
-0.219458808300145));
#82691=CARTESIAN_POINT('Ctrl Pts',(0.142219604478747,0.133995313731148,
-0.218762122224941));
#82692=CARTESIAN_POINT('Ctrl Pts',(0.133861968766583,0.14286591981627,-0.218066889782627));
#82693=CARTESIAN_POINT('Ctrl Pts',(0.124653231947698,0.150970738568163,
-0.217371657340313));
#82694=CARTESIAN_POINT('Ctrl Pts',(0.114759345905742,0.158150094932903,
-0.216676424898));
#82695=CARTESIAN_POINT('Ctrl Pts',(0.104866826189024,0.16532845984335,-0.215981288465851));
#82696=CARTESIAN_POINT('Ctrl Pts',(0.0942900255519612,0.171581066289418,
-0.215286152033703));
#82697=CARTESIAN_POINT('Ctrl Pts',(0.0832271523410599,0.176789143086328,
-0.214591015601554));
#82698=CARTESIAN_POINT('Ctrl Pts',(0.0721648530419438,0.181996949702373,
-0.213895915231194));
#82699=CARTESIAN_POINT('Ctrl Pts',(0.0606173343890308,0.186159986037156,
-0.213200814860834));
#82700=CARTESIAN_POINT('Ctrl Pts',(0.0488039281591277,0.18920712617721,
-0.212505714490473));
#82701=CARTESIAN_POINT('Ctrl Pts',(0.0369635332665546,0.19226122775038,
-0.211809026108234));
#82702=CARTESIAN_POINT('Ctrl Pts',(0.0248569010483798,0.194194188646917,
-0.211112337725996));
#82703=CARTESIAN_POINT('Ctrl Pts',(0.0127135273208923,0.194985964169375,
-0.210415649343757));
#82704=CARTESIAN_POINT('Ctrl Pts',(0.00894864306373339,0.195231443166119,
-0.21019965079333));
#82705=CARTESIAN_POINT('Ctrl Pts',(0.00518023811354474,0.195367607366277,
-0.209983652242902));
#82706=CARTESIAN_POINT('Ctrl Pts',(0.00141511774680491,0.195394875679386,
-0.209767653692475));
#82707=CARTESIAN_POINT('Ctrl Pts',(-0.0107289779310962,0.195482827450142,
-0.20907096758229));
#82708=CARTESIAN_POINT('Ctrl Pts',(-0.0229239239752086,0.194434598883651,
-0.208374281472106));
#82709=CARTESIAN_POINT('Ctrl Pts',(-0.0349401738991443,0.192250732762966,
-0.207677595361922));
#82710=CARTESIAN_POINT('Ctrl Pts',(-0.0469313519681011,0.190071423269767,
-0.20698236288438));
#82711=CARTESIAN_POINT('Ctrl Pts',(-0.0587437084385229,0.186761261699367,
-0.206287130406837));
#82712=CARTESIAN_POINT('Ctrl Pts',(-0.0701529502464144,0.182372485785888,
-0.205591897929295));
#82713=CARTESIAN_POINT('Ctrl Pts',(-0.0815606164587637,0.177984315954381,
-0.204896761462093));
#82714=CARTESIAN_POINT('Ctrl Pts',(-0.0925644468468266,0.172518098822333,
-0.204201624994891));
#82715=CARTESIAN_POINT('Ctrl Pts',(-0.102956890375255,0.166075400719847,
-0.203506488527689));
#82716=CARTESIAN_POINT('Ctrl Pts',(-0.113348794770967,0.159633036847642,
-0.202811388122344));
#82717=CARTESIAN_POINT('Ctrl Pts',(-0.123128645861872,0.152214776589438,
-0.202116287716999));
#82718=CARTESIAN_POINT('Ctrl Pts',(-0.132117351332421,0.14396584830058,
-0.201421187311655));
#82719=CARTESIAN_POINT('Ctrl Pts',(-0.141126592202309,0.135698074691104,
-0.200724498895172));
#82720=CARTESIAN_POINT('Ctrl Pts',(-0.149340479210109,0.12659648382991,
-0.200027810478689));
#82721=CARTESIAN_POINT('Ctrl Pts',(-0.156617228512917,0.11684264518117,
-0.199331122062206));
#82722=CARTESIAN_POINT('Ctrl Pts',(-0.158873281569522,0.113818605657282,
-0.199115123686269));
#82723=CARTESIAN_POINT('Ctrl Pts',(-0.161039566480852,0.110732086044716,
-0.198899125310332));
#82724=CARTESIAN_POINT('Ctrl Pts',(-0.16311272879862,0.107589022227493,
-0.198683126934395));
#82725=CARTESIAN_POINT('Ctrl Pts',(-0.169922682695037,0.0972646402409293,
-0.19797361231066));
#82726=CARTESIAN_POINT('Ctrl Pts',(-0.175770941149539,0.0862577317658504,
-0.197264097686925));
#82727=CARTESIAN_POINT('Ctrl Pts',(-0.180529547933672,0.0747679230878049,
-0.196554583063191));
#82728=CARTESIAN_POINT('Ctrl Pts',(-0.185411701687211,0.0629798062902586,
-0.195826647421396));
#82729=CARTESIAN_POINT('Ctrl Pts',(-0.189146194866463,0.0506840503841172,
-0.195098711779602));
#82730=CARTESIAN_POINT('Ctrl Pts',(-0.191644763603409,0.038124068295415,
-0.194370776137807));
#82731=CARTESIAN_POINT('Ctrl Pts',(-0.194143332340355,0.0255640862067136,
-0.193642840496012));
#82732=CARTESIAN_POINT('Ctrl Pts',(-0.195405700671203,0.012740798323454,
-0.192914904854218));
#82733=CARTESIAN_POINT('Ctrl Pts',(-0.195399980573782,-8.71307379076436E-5,
-0.192186969212423));
#82734=CARTESIAN_POINT('',(-0.195399970103672,-0.000108090166289862,-0.122186969217338));
#82735=CARTESIAN_POINT('Ctrl Pts',(-0.195399980573749,-8.71308121576554E-5,
-0.19218696920821));
#82736=CARTESIAN_POINT('Ctrl Pts',(-0.195393971356559,-0.0135634303337909,
-0.191422241036227));
#82737=CARTESIAN_POINT('Ctrl Pts',(-0.193989563708496,-0.0269934619489129,
-0.190657512864245));
#82738=CARTESIAN_POINT('Ctrl Pts',(-0.191240294421705,-0.0401037378494752,
-0.189892784692262));
#82739=CARTESIAN_POINT('Ctrl Pts',(-0.188491025134915,-0.0532140137500375,
-0.18912805652028));
#82740=CARTESIAN_POINT('Ctrl Pts',(-0.184397210802687,-0.066004022077199,
-0.188363328348297));
#82741=CARTESIAN_POINT('Ctrl Pts',(-0.179060927217783,-0.0782198462278453,
-0.187598600176314));
#82742=CARTESIAN_POINT('Ctrl Pts',(-0.174199442314772,-0.089348760900636,
-0.186901914101849));
#82743=CARTESIAN_POINT('Ctrl Pts',(-0.168279411507396,-0.100061776817748,
-0.186205228027384));
#82744=CARTESIAN_POINT('Ctrl Pts',(-0.161394740466552,-0.110149433724075,
-0.185508541952918));
#82745=CARTESIAN_POINT('Ctrl Pts',(-0.15452443427393,-0.120216042760501,
-0.184813309512136));
#82746=CARTESIAN_POINT('Ctrl Pts',(-0.146693910245396,-0.129659125533717,
-0.184118077071353));
#82747=CARTESIAN_POINT('Ctrl Pts',(-0.138042157449026,-0.138295056913898,
-0.18342284463057));
#82748=CARTESIAN_POINT('Ctrl Pts',(-0.12939159945556,-0.146929795676105,
-0.182727708201054));
#82749=CARTESIAN_POINT('Ctrl Pts',(-0.119920624130205,-0.154756955044027,
-0.182032571771537));
#82750=CARTESIAN_POINT('Ctrl Pts',(-0.109806467286001,-0.161628276431348,
-0.18133743534202));
#82751=CARTESIAN_POINT('Ctrl Pts',(-0.0996928351460712,-0.168499241346869,
-0.180642334974932));
#82752=CARTESIAN_POINT('Ctrl Pts',(-0.088936826680016,-0.174413997399687,
-0.179947234607844));
#82753=CARTESIAN_POINT('Ctrl Pts',(-0.0777439803686978,-0.179268049346311,
-0.179252134240755));
#82754=CARTESIAN_POINT('Ctrl Pts',(-0.0665255631267537,-0.184133190753304,
-0.178555445862649));
#82755=CARTESIAN_POINT('Ctrl Pts',(-0.0548691438273311,-0.187932502481423,
-0.177858757484542));
#82756=CARTESIAN_POINT('Ctrl Pts',(-0.0429982750156473,-0.190610357393502,
-0.177162069106436));
#82757=CARTESIAN_POINT('Ctrl Pts',(-0.0393178768888787,-0.191440589144735,
-0.176946070543702));
#82758=CARTESIAN_POINT('Ctrl Pts',(-0.035616935330501,-0.192163396083465,
-0.176730071980969));
#82759=CARTESIAN_POINT('Ctrl Pts',(-0.0319022375746728,-0.192778129562793,
-0.176514073418235));
#82760=CARTESIAN_POINT('Ctrl Pts',(-0.0199207737687746,-0.194760903779428,
-0.17581738713805));
#82761=CARTESIAN_POINT('Ctrl Pts',(-0.007711706010355,-0.19562936689701,
-0.175120700857864));
#82762=CARTESIAN_POINT('Ctrl Pts',(0.0044981489421037,-0.195348218973439,
-0.174424014577679));
#82763=CARTESIAN_POINT('Ctrl Pts',(0.0166825281058876,-0.195067657663314,
-0.173728781929213));
#82764=CARTESIAN_POINT('Ctrl Pts',(0.0288668234303841,-0.193642192521187,
-0.173033549280747));
#82765=CARTESIAN_POINT('Ctrl Pts',(0.040821336716632,-0.191088404851439,
-0.172338316632281));
#82766=CARTESIAN_POINT('Ctrl Pts',(0.0527741990849647,-0.188534969859689,
-0.171643179995422));
#82767=CARTESIAN_POINT('Ctrl Pts',(0.0644964785721529,-0.184853659848699,
-0.170948043358563));
#82768=CARTESIAN_POINT('Ctrl Pts',(0.0757673127012417,-0.180112393593645,
-0.170252906721704));
#82769=CARTESIAN_POINT('Ctrl Pts',(0.0870375621198938,-0.175371373306888,
-0.169557806147274));
#82770=CARTESIAN_POINT('Ctrl Pts',(0.0978556166444629,-0.169570870150772,
-0.168862705572843));
#82771=CARTESIAN_POINT('Ctrl Pts',(0.10802190718798,-0.162826372456895,
-0.168167604998413));
#82772=CARTESIAN_POINT('Ctrl Pts',(0.118211423352824,-0.156066466473356,
-0.167470916416768));
#82773=CARTESIAN_POINT('Ctrl Pts',(0.127745510547746,-0.148358798376342,
-0.166774227835123));
#82774=CARTESIAN_POINT('Ctrl Pts',(0.136455777234141,-0.139860576501838,
-0.166077539253478));
#82775=CARTESIAN_POINT('Ctrl Pts',(0.139156260849229,-0.137225834104648,
-0.16586154172237));
#82776=CARTESIAN_POINT('Ctrl Pts',(0.141777831823451,-0.134515363975046,
-0.165645544191262));
#82777=CARTESIAN_POINT('Ctrl Pts',(0.144316250195574,-0.131734505462649,
-0.165429546660155));
#82778=CARTESIAN_POINT('Ctrl Pts',(0.152503749882229,-0.122765031222731,
-0.164732860984663));
#82779=CARTESIAN_POINT('Ctrl Pts',(0.159880587869742,-0.112997862757875,
-0.164036175309172));
#82780=CARTESIAN_POINT('Ctrl Pts',(0.166293644268259,-0.10260401491161,
-0.16333948963368));
#82781=CARTESIAN_POINT('Ctrl Pts',(0.172693319853186,-0.092231853782545,
-0.162644257589745));
#82782=CARTESIAN_POINT('Ctrl Pts',(0.178132687595168,-0.0812363071400706,
-0.16194902554581));
#82783=CARTESIAN_POINT('Ctrl Pts',(0.182500572794291,-0.0698190584994946,
-0.161253793501875));
#82784=CARTESIAN_POINT('Ctrl Pts',(0.186867854846755,-0.0584033864285969,
-0.160558657460208));
#82785=CARTESIAN_POINT('Ctrl Pts',(0.190163593566233,-0.0465669277301283,
-0.15986352141854));
#82786=CARTESIAN_POINT('Ctrl Pts',(0.192324483949466,-0.034531910945844,
-0.159168385376873));
#82787=CARTESIAN_POINT('Ctrl Pts',(0.194485262244566,-0.0224975184331854,
-0.158473285392796));
#82788=CARTESIAN_POINT('Ctrl Pts',(0.19551118106135,-0.010265454266999,
-0.157778185408719));
#82789=CARTESIAN_POINT('Ctrl Pts',(0.195390428658573,0.00193400843301484,
-0.157083085424642));
#82790=CARTESIAN_POINT('Ctrl Pts',(0.195269400384929,0.014161342018218,
-0.156386397415558));
#82791=CARTESIAN_POINT('Ctrl Pts',(0.193996545096175,0.0263550518336399,
-0.155689709406473));
#82792=CARTESIAN_POINT('Ctrl Pts',(0.191612020533415,0.0382882956933619,
-0.154993021397388));
#82793=CARTESIAN_POINT('Ctrl Pts',(0.190872724769203,0.0419880674535577,
-0.15477702089895));
#82794=CARTESIAN_POINT('Ctrl Pts',(0.190026939225289,0.0456628897167423,
-0.154561020400512));
#82795=CARTESIAN_POINT('Ctrl Pts',(0.189076833400025,0.0493062984964319,
-0.154345019902075));
#82796=CARTESIAN_POINT('Ctrl Pts',(0.186012370094469,0.0610577184073582,
-0.153648333718449));
#82797=CARTESIAN_POINT('Ctrl Pts',(0.181837411076989,0.0725635961155488,
-0.152951647534823));
#82798=CARTESIAN_POINT('Ctrl Pts',(0.176612010267933,0.0836023793269029,
-0.152254961351197));
#82799=CARTESIAN_POINT('Ctrl Pts',(0.171397512282338,0.0946181300649645,
-0.151559728806582));
#82800=CARTESIAN_POINT('Ctrl Pts',(0.165137226816864,0.105167906177253,
-0.150864496261968));
#82801=CARTESIAN_POINT('Ctrl Pts',(0.157939771708267,0.1150486354232,-0.150169263717353));
#82802=CARTESIAN_POINT('Ctrl Pts',(0.150743310659152,0.124928000015606,
-0.149474127193137));
#82803=CARTESIAN_POINT('Ctrl Pts',(0.142610414659424,0.134137768326967,
-0.148778990668921));
#82804=CARTESIAN_POINT('Ctrl Pts',(0.133693000655849,0.142503830038477,
-0.148083854144704));
#82805=CARTESIAN_POINT('Ctrl Pts',(0.124776049338251,0.150869457671292,
-0.14738875368811));
#82806=CARTESIAN_POINT('Ctrl Pts',(0.115075317446932,0.158390886677845,
-0.146693653231516));
#82807=CARTESIAN_POINT('Ctrl Pts',(0.104777509781274,0.164932814940008,
-0.145998552774923));
#82808=CARTESIAN_POINT('Ctrl Pts',(0.0944561761087307,0.171489688659917,
-0.14530186431643));
#82809=CARTESIAN_POINT('Ctrl Pts',(0.0835358165499775,0.177062180688005,
-0.144605175857937));
#82810=CARTESIAN_POINT('Ctrl Pts',(0.0722285582496733,0.181560445508303,
-0.143908487399444));
#82811=CARTESIAN_POINT('Ctrl Pts',(0.0687229078956497,0.182955066842756,
-0.143692489314294));
#82812=CARTESIAN_POINT('Ctrl Pts',(0.0651801953146029,0.184246788178321,
-0.143476491229144));
#82813=CARTESIAN_POINT('Ctrl Pts',(0.0616070232095414,0.18543390922714,
-0.143260493143995));
#82814=CARTESIAN_POINT('Ctrl Pts',(0.0500819964771528,0.189262888470214,
-0.142563805821834));
#82815=CARTESIAN_POINT('Ctrl Pts',(0.0381581932723761,0.192026748952457,
-0.141867118499673));
#82816=CARTESIAN_POINT('Ctrl Pts',(0.0260541390244445,0.193655213820065,
-0.141170431177512));
#82817=CARTESIAN_POINT('Ctrl Pts',(0.0139753396432458,0.195280280928346,
-0.140475197479493));
#82818=CARTESIAN_POINT('Ctrl Pts',(0.00171788443870832,0.195774465915562,
-0.139779963781474));
#82819=CARTESIAN_POINT('Ctrl Pts',(-0.0104887555978503,0.195118287215752,
-0.139084730083456));
#82820=CARTESIAN_POINT('Ctrl Pts',(-0.0226937098116175,0.194462199138832,
-0.138389592402098));
#82821=CARTESIAN_POINT('Ctrl Pts',(-0.0348469879742808,0.192656064389134,
-0.137694454720739));
#82822=CARTESIAN_POINT('Ctrl Pts',(-0.0467198318879055,0.189732488805597,
-0.136999317039381));
#82823=CARTESIAN_POINT('Ctrl Pts',(-0.0585920598278827,0.186809064899747,
-0.136304215422381));
#82824=CARTESIAN_POINT('Ctrl Pts',(-0.0701830392759854,0.182768550720884,
-0.135609113805381));
#82825=CARTESIAN_POINT('Ctrl Pts',(-0.0812776179338772,0.177693862648643,
-0.134914012188381));
#82826=CARTESIAN_POINT('Ctrl Pts',(-0.0923975425663838,0.172607581264116,
-0.13421732258607));
#82827=CARTESIAN_POINT('Ctrl Pts',(-0.103018034568636,0.166482832497714,
-0.133520632983759));
#82828=CARTESIAN_POINT('Ctrl Pts',(-0.112948223695707,0.159448608535742,
-0.132823943381448));
#82829=CARTESIAN_POINT('Ctrl Pts',(-0.116026846798592,0.157267811763085,
-0.132607951049604));
#82830=CARTESIAN_POINT('Ctrl Pts',(-0.119039350369695,0.154999900408411,
-0.132391958717759));
#82831=CARTESIAN_POINT('Ctrl Pts',(-0.121980713235812,0.152649486073431,
-0.132175966385915));
#82832=CARTESIAN_POINT('Ctrl Pts',(-0.131351103176399,0.145161699002201,
-0.131487872986465));
#82833=CARTESIAN_POINT('Ctrl Pts',(-0.140066232538382,0.136778248077627,
-0.130799779587016));
#82834=CARTESIAN_POINT('Ctrl Pts',(-0.147950444101791,0.127639437832054,
-0.130111686187566));
#82835=CARTESIAN_POINT('Ctrl Pts',(-0.155823820626387,0.118513186783163,
-0.129424538414528));
#82836=CARTESIAN_POINT('Ctrl Pts',(-0.162867891285451,0.108634248342843,
-0.12873739064149));
#82837=CARTESIAN_POINT('Ctrl Pts',(-0.168943071069768,0.0981804396889495,
-0.128050242868453));
#82838=CARTESIAN_POINT('Ctrl Pts',(-0.175012463749694,0.0877365891406759,
-0.12736374965973));
#82839=CARTESIAN_POINT('Ctrl Pts',(-0.180114328175564,0.076719721605862,
-0.126677256451007));
#82840=CARTESIAN_POINT('Ctrl Pts',(-0.18415346816745,0.0653349842113701,
-0.125990763242284));
#82841=CARTESIAN_POINT('Ctrl Pts',(-0.188200722658696,0.0539273752540016,
-0.12530289089129));
#82842=CARTESIAN_POINT('Ctrl Pts',(-0.191180699002706,0.042151276700291,
-0.124615018540296));
#82843=CARTESIAN_POINT('Ctrl Pts',(-0.19304760334189,0.0302288412604957,
-0.123927146189302));
#82844=CARTESIAN_POINT('Ctrl Pts',(-0.19462189927786,0.0201750633213751,
-0.123347087198647));
#82845=CARTESIAN_POINT('Ctrl Pts',(-0.195405571471215,0.0100177805586885,
-0.122767028207992));
#82846=CARTESIAN_POINT('Ctrl Pts',(-0.195399970103672,-0.000108090166289968,
-0.122186969217338));
#82847=CARTESIAN_POINT('',(-0.195399922633752,0.000173881349547679,-0.0521869692124231));
#82848=CARTESIAN_POINT('Ctrl Pts',(-0.195399970103625,-0.00010809025208222,
-0.122186969212423));
#82849=CARTESIAN_POINT('Ctrl Pts',(-0.195396443756117,-0.00648283898595459,
-0.121821792684227));
#82850=CARTESIAN_POINT('Ctrl Pts',(-0.195080985395644,-0.0128487550321653,
-0.12145661615603));
#82851=CARTESIAN_POINT('Ctrl Pts',(-0.194456030652044,-0.0191836425907903,
-0.121091439627833));
#82852=CARTESIAN_POINT('Ctrl Pts',(-0.193263735271741,-0.0312694091974816,
-0.120394751920406));
#82853=CARTESIAN_POINT('Ctrl Pts',(-0.19093622320459,-0.0432860108823252,
-0.119698064212978));
#82854=CARTESIAN_POINT('Ctrl Pts',(-0.18749822409405,-0.0550052357651287,
-0.119001376505551));
#82855=CARTESIAN_POINT('Ctrl Pts',(-0.184067398541676,-0.066700007895429,
-0.118306142472087));
#82856=CARTESIAN_POINT('Ctrl Pts',(-0.179530858135104,-0.0780977827826907,
-0.117610908438624));
#82857=CARTESIAN_POINT('Ctrl Pts',(-0.173964186021277,-0.0889810203467823,
-0.11691567440516));
#82858=CARTESIAN_POINT('Ctrl Pts',(-0.168398283310568,-0.0998627536733787,
-0.11622053646416));
#82859=CARTESIAN_POINT('Ctrl Pts',(-0.161802889014412,-0.110229292410544,
-0.115525398523159));
#82860=CARTESIAN_POINT('Ctrl Pts',(-0.154300875937143,-0.11988494352933,
-0.114830260582159));
#82861=CARTESIAN_POINT('Ctrl Pts',(-0.146799252541534,-0.129540093098714,
-0.114135158749134));
#82862=CARTESIAN_POINT('Ctrl Pts',(-0.138391662039633,-0.138483754014547,
-0.11344005691611));
#82863=CARTESIAN_POINT('Ctrl Pts',(-0.129241397230523,-0.14655313453455,
-0.112744955083086));
#82864=CARTESIAN_POINT('Ctrl Pts',(-0.120070229188774,-0.154640949071688,
-0.112048265331501));
#82865=CARTESIAN_POINT('Ctrl Pts',(-0.110153698806983,-0.161849966760308,
-0.111351575579916));
#82866=CARTESIAN_POINT('Ctrl Pts',(-0.0996873061692639,-0.168058326151118,
-0.110654885828331));
#82867=CARTESIAN_POINT('Ctrl Pts',(-0.096442466608256,-0.169983070507416,
-0.110438894842139));
#82868=CARTESIAN_POINT('Ctrl Pts',(-0.0931449582544428,-0.171811968871328,
-0.110222903855947));
#82869=CARTESIAN_POINT('Ctrl Pts',(-0.0898010367685515,-0.173542311253749,
-0.110006912869755));
#82870=CARTESIAN_POINT('Ctrl Pts',(-0.0790149934579321,-0.179123646807751,
-0.109310219439123));
#82871=CARTESIAN_POINT('Ctrl Pts',(-0.0676687750586451,-0.183715158419008,
-0.108613526008491));
#82872=CARTESIAN_POINT('Ctrl Pts',(-0.05596726049107,-0.187213316174691,
-0.10791683257786));
#82873=CARTESIAN_POINT('Ctrl Pts',(-0.0442901596874042,-0.190704175456567,
-0.107221592711963));
#82874=CARTESIAN_POINT('Ctrl Pts',(-0.0322600429270558,-0.193105889868855,
-0.106526352846067));
#82875=CARTESIAN_POINT('Ctrl Pts',(-0.0201005299208599,-0.194363393407557,
-0.105831112980171));
#82876=CARTESIAN_POINT('Ctrl Pts',(-0.00794269636402312,-0.195620723262205,
-0.105135969139514));
#82877=CARTESIAN_POINT('Ctrl Pts',(0.00434363363409507,-0.195734021012792,
-0.104440825298858));
#82878=CARTESIAN_POINT('Ctrl Pts',(0.016527413097827,-0.194699780729958,
-0.103745681458201));
#82879=CARTESIAN_POINT('Ctrl Pts',(0.0287105604776149,-0.193665594102615,
-0.103050573681005));
#82880=CARTESIAN_POINT('Ctrl Pts',(0.0407902983536555,-0.191484088585282,
-0.10235546590381));
#82881=CARTESIAN_POINT('Ctrl Pts',(0.052541164632059,-0.188203575999785,
-0.101660358126615));
#82882=CARTESIAN_POINT('Ctrl Pts',(0.0643188740718153,-0.184915569555829,
-0.100963662475829));
#82883=CARTESIAN_POINT('Ctrl Pts',(0.0757653876272328,-0.180523842190735,
-0.100266966825044));
#82884=CARTESIAN_POINT('Ctrl Pts',(0.0866720342857299,-0.175126007414014,
-0.0995702711742589));
#82885=CARTESIAN_POINT('Ctrl Pts',(0.0900528761425629,-0.173452786824697,
-0.0993543094867303));
#82886=CARTESIAN_POINT('Ctrl Pts',(0.0933820236128782,-0.171683224940323,
-0.0991383477992016));
#82887=CARTESIAN_POINT('Ctrl Pts',(0.0966537995815988,-0.169821091229682,
-0.098922386111673));
#82888=CARTESIAN_POINT('Ctrl Pts',(0.107208132624148,-0.163814084778215,
-0.0982257211821669));
#82889=CARTESIAN_POINT('Ctrl Pts',(0.117237377398798,-0.156798305440679,
-0.0975290562526608));
#82890=CARTESIAN_POINT('Ctrl Pts',(0.126543142295318,-0.148889197519588,
-0.0968323913231549));
#82891=CARTESIAN_POINT('Ctrl Pts',(0.135829490272315,-0.140996592327043,
-0.0961371800180442));
#82892=CARTESIAN_POINT('Ctrl Pts',(0.144394646745838,-0.13221486312393,
-0.0954419687129335));
#82893=CARTESIAN_POINT('Ctrl Pts',(0.152070661114356,-0.122701564897285,
-0.0947467574078229));
#82894=CARTESIAN_POINT('Ctrl Pts',(0.159745619057451,-0.113189575955592,
-0.0940516417824312));
#82895=CARTESIAN_POINT('Ctrl Pts',(0.166531093883671,-0.102946869348848,
-0.0933565261570396));
#82896=CARTESIAN_POINT('Ctrl Pts',(0.172298334522415,-0.0921653075772113,
-0.0926614105316478));
#82897=CARTESIAN_POINT('Ctrl Pts',(0.178065277385181,-0.0813843024825551,
-0.0919663307966842));
#82898=CARTESIAN_POINT('Ctrl Pts',(0.182813701569087,-0.0700652818063663,
-0.0912712510617206));
#82899=CARTESIAN_POINT('Ctrl Pts',(0.186461358328499,-0.0584236411933643,
-0.090576171326757));
#82900=CARTESIAN_POINT('Ctrl Pts',(0.190117351977106,-0.0467553930692292,
-0.0898795029547274));
#82901=CARTESIAN_POINT('Ctrl Pts',(0.192667356649156,-0.0347639068879149,
-0.0891828345826979));
#82902=CARTESIAN_POINT('Ctrl Pts',(0.194079618128655,-0.0226773417100732,
-0.0884861662106683));
#82903=CARTESIAN_POINT('Ctrl Pts',(0.194517693037703,-0.0189281628095307,
-0.088270063924977));
#82904=CARTESIAN_POINT('Ctrl Pts',(0.194846671950056,-0.01516986575135,
-0.0880539616392856));
#82905=CARTESIAN_POINT('Ctrl Pts',(0.195066625456177,-0.0114092783794373,
-0.0878378593535943));
#82906=CARTESIAN_POINT('Ctrl Pts',(0.195775744890149,0.000714672884618461,
-0.087141156067469));
#82907=CARTESIAN_POINT('Ctrl Pts',(0.195352724954443,0.0129475304762241,
-0.0864444527813439));
#82908=CARTESIAN_POINT('Ctrl Pts',(0.193786366364896,0.0250600121925408,
-0.0857477494952185));
#82909=CARTESIAN_POINT('Ctrl Pts',(0.192223276489041,0.0371472172990852,
-0.0850525001057845));
#82910=CARTESIAN_POINT('Ctrl Pts',(0.189521621688646,0.0491136765680657,
-0.0843572507163504));
#82911=CARTESIAN_POINT('Ctrl Pts',(0.185722098668139,0.0607327100194129,
-0.0836620013269164));
#82912=CARTESIAN_POINT('Ctrl Pts',(0.181923103784017,0.0723501284168967,
-0.0829668485776389));
#82913=CARTESIAN_POINT('Ctrl Pts',(0.177026772057464,0.0836193724441967,
-0.0822716958283615));
#82914=CARTESIAN_POINT('Ctrl Pts',(0.171123920650509,0.0943279586400468,
-0.081576543079084));
#82915=CARTESIAN_POINT('Ctrl Pts',(0.165221378424207,0.105035983939569,
-0.0808814267406471));
#82916=CARTESIAN_POINT('Ctrl Pts',(0.158312867207656,0.115182656519121,
-0.0801863104022101));
#82917=CARTESIAN_POINT('Ctrl Pts',(0.150534265355772,0.124581679848194,
-0.0794911940637732));
#82918=CARTESIAN_POINT('Ctrl Pts',(0.142737901980521,0.134002164742685,
-0.0787944905088514));
#82919=CARTESIAN_POINT('Ctrl Pts',(0.134068089445645,0.142670960403978,
-0.0780977869539296));
#82920=CARTESIAN_POINT('Ctrl Pts',(0.124698909072924,0.150437169861782,
-0.0774010833990079));
#82921=CARTESIAN_POINT('Ctrl Pts',(0.121795285730477,0.152844012954446,
-0.0771851664645099));
#82922=CARTESIAN_POINT('Ctrl Pts',(0.118824722122236,0.155164466597326,
-0.0769692495300118));
#82923=CARTESIAN_POINT('Ctrl Pts',(0.11579296795291,0.157394881024309,-0.0767533325955138));
#82924=CARTESIAN_POINT('Ctrl Pts',(0.106010014886606,0.164592047561869,
-0.0760566055132901));
#82925=CARTESIAN_POINT('Ctrl Pts',(0.0955191818643613,0.170898866630626,
-0.0753598784310665));
#82926=CARTESIAN_POINT('Ctrl Pts',(0.0845066983866875,0.176181094126985,
-0.0746631513488428));
#82927=CARTESIAN_POINT('Ctrl Pts',(0.0735171828830057,0.181452304847336,
-0.0739678773820345));
#82928=CARTESIAN_POINT('Ctrl Pts',(0.0620089255354657,0.185702724447798,
-0.0732726034152262));
#82929=CARTESIAN_POINT('Ctrl Pts',(0.050194229633594,0.188843054708109,
-0.072577329448418));
#82930=CARTESIAN_POINT('Ctrl Pts',(0.0383811633695494,0.191982951812882,
-0.0718821513829149));
#82931=CARTESIAN_POINT('Ctrl Pts',(0.0262625750398239,0.194012795377422,
-0.0711869733174118));
#82932=CARTESIAN_POINT('Ctrl Pts',(0.0140661510316737,0.194893056303076,
-0.0704917952519087));
#82933=CARTESIAN_POINT('Ctrl Pts',(0.0018703579051073,0.195773271695679,
-0.0697966531457195));
#82934=CARTESIAN_POINT('Ctrl Pts',(-0.0104023883744724,0.195503986493105,
-0.0691015110395303));
#82935=CARTESIAN_POINT('Ctrl Pts',(-0.0225218293580419,0.194097725907253,
-0.0684063689333411));
#82936=CARTESIAN_POINT('Ctrl Pts',(-0.0346689457229234,0.192688254051345,
-0.0677096394335682));
#82937=CARTESIAN_POINT('Ctrl Pts',(-0.0466611970798801,0.190136789244532,
-0.0670129099337952));
#82938=CARTESIAN_POINT('Ctrl Pts',(-0.0582772135502686,0.186507175145667,
-0.0663161804340223));
#82939=CARTESIAN_POINT('Ctrl Pts',(-0.0618749340328637,0.185383008610548,
-0.0661003889018261));
#82940=CARTESIAN_POINT('Ctrl Pts',(-0.0654366891829184,0.184155775180138,
-0.06588459736963));
#82941=CARTESIAN_POINT('Ctrl Pts',(-0.0689562978851465,0.182828304652138,
-0.0656688058374338));
#82942=CARTESIAN_POINT('Ctrl Pts',(-0.0803170025061345,0.178543453170741,
-0.0649722670842936));
#82943=CARTESIAN_POINT('Ctrl Pts',(-0.0913167663370378,0.173180569663799,
-0.0642757283311535));
#82944=CARTESIAN_POINT('Ctrl Pts',(-0.101741656481082,0.166822646353801,
-0.0635791895780133));
#82945=CARTESIAN_POINT('Ctrl Pts',(-0.112144788823725,0.160477992673583,
-0.0628841045717855));
#82946=CARTESIAN_POINT('Ctrl Pts',(-0.121974650517319,0.153142809387216,
-0.0621890195655576));
#82947=CARTESIAN_POINT('Ctrl Pts',(-0.131040793938003,0.144946439501279,
-0.0614939345593297));
#82948=CARTESIAN_POINT('Ctrl Pts',(-0.140105711886504,0.136751177520083,
-0.060798943507863));
#82949=CARTESIAN_POINT('Ctrl Pts',(-0.14840643765987,0.127695512494498,
-0.0601039524563963));
#82950=CARTESIAN_POINT('Ctrl Pts',(-0.155785882235974,0.11794879777242,
-0.0594089614049295));
#82951=CARTESIAN_POINT('Ctrl Pts',(-0.163164955042303,0.108202574081056,
-0.0587140053664863));
#82952=CARTESIAN_POINT('Ctrl Pts',(-0.169622332052514,0.0977660841308201,
-0.0580190493280431));
#82953=CARTESIAN_POINT('Ctrl Pts',(-0.175043182851466,0.0868391854938099,
-0.0573240932895998));
#82954=CARTESIAN_POINT('Ctrl Pts',(-0.180476453002008,0.0758872529643354,
-0.0566275450834874));
#82955=CARTESIAN_POINT('Ctrl Pts',(-0.184868126208397,0.0644434814927237,
-0.0559309968773751));
#82956=CARTESIAN_POINT('Ctrl Pts',(-0.188151256341738,0.0527282157580304,
-0.0552344486712627));
#82957=CARTESIAN_POINT('Ctrl Pts',(-0.189172765626258,0.0490831416267694,
-0.0550177254739597));
#82958=CARTESIAN_POINT('Ctrl Pts',(-0.190087330366273,0.045411874308117,
-0.0548010022766568));
#82959=CARTESIAN_POINT('Ctrl Pts',(-0.190893947145442,0.0417212289276486,
-0.0545842790793538));
#82960=CARTESIAN_POINT('Ctrl Pts',(-0.193868110175516,0.0281130554663777,
-0.0537851757903769));
#82961=CARTESIAN_POINT('Ctrl Pts',(-0.195387462253079,0.0141762883117028,
-0.0529860725014));
#82962=CARTESIAN_POINT('Ctrl Pts',(-0.195399922633752,0.000173881349547679,
-0.0521869692124231));
#82963=CARTESIAN_POINT('',(0.00542534466917562,0.195638851078239,1.80411241501588E-16));
#82964=CARTESIAN_POINT('Ctrl Pts',(-0.195432320986697,0.000173604797042496,
-0.0521869517874278));
#82965=CARTESIAN_POINT('Ctrl Pts',(-0.19496687862426,-0.0505761822068533,
-0.0492912186320431));
#82966=CARTESIAN_POINT('Ctrl Pts',(-0.148879977450944,-0.166826599982022,
-0.0427006432239653));
#82967=CARTESIAN_POINT('Ctrl Pts',(0.0467197021695734,-0.225989356129055,
-0.032415225563194));
#82968=CARTESIAN_POINT('Ctrl Pts',(0.214983941469384,-0.0838177601457405,
-0.021330698805113));
#82969=CARTESIAN_POINT('Ctrl Pts',(0.18806769685446,0.129051521723346,-0.0105256236173826));
#82970=CARTESIAN_POINT('Ctrl Pts',(0.0650705990701268,0.193654330577805,
-0.0034153906823444));
#82971=CARTESIAN_POINT('Ctrl Pts',(0.00542534466917562,0.195638851078239,
1.80411241501588E-16));
#82972=CARTESIAN_POINT('',(0.157947475570094,0.115038058750287,0.));
#82973=CARTESIAN_POINT('Origin',(0.,0.,0.));
#82974=CARTESIAN_POINT('',(-0.195399925034678,0.000171162035267742,-0.0420130307875766));
#82975=CARTESIAN_POINT('Ctrl Pts',(0.157947475570094,0.115038058750287,
0.));
#82976=CARTESIAN_POINT('Ctrl Pts',(0.196099648170939,0.0626550525062515,
-0.0036948422526933));
#82977=CARTESIAN_POINT('Ctrl Pts',(0.2155636754795,-0.0821381146635345,
-0.0110845267580803));
#82978=CARTESIAN_POINT('Ctrl Pts',(0.0481663642357293,-0.22581952090303,
-0.0221690535161595));
#82979=CARTESIAN_POINT('Ctrl Pts',(-0.148247008667004,-0.167596420983037,
-0.0324785467239276));
#82980=CARTESIAN_POINT('Ctrl Pts',(-0.19497457278765,-0.0509793119047676,
-0.039093197679001));
#82981=CARTESIAN_POINT('Ctrl Pts',(-0.195445212794411,0.000170774153815293,
-0.0420130063813814));
#82982=CARTESIAN_POINT('',(-0.195399966640887,-0.00011417854461868,-0.112013030792447));
#82983=CARTESIAN_POINT('Ctrl Pts',(-0.195399925034678,0.000171162035267742,
-0.0420130307875766));
#82984=CARTESIAN_POINT('Ctrl Pts',(-0.195388034908535,0.0137450235125697,
-0.0427880562024912));
#82985=CARTESIAN_POINT('Ctrl Pts',(-0.193960346547734,0.0272581797347334,
-0.0435630816174058));
#82986=CARTESIAN_POINT('Ctrl Pts',(-0.191162448998049,0.0404731774520893,
-0.0443381070323203));
#82987=CARTESIAN_POINT('Ctrl Pts',(-0.18865081136394,0.0523361156091008,
-0.0450338376532321));
#82988=CARTESIAN_POINT('Ctrl Pts',(-0.185021626603632,0.0640071061046373,
-0.0457295682741437));
#82989=CARTESIAN_POINT('Ctrl Pts',(-0.180323926183208,0.0752624849833763,
-0.0464252988950553));
#82990=CARTESIAN_POINT('Ctrl Pts',(-0.175636184117986,0.0864940043030182,
-0.0471195546810419));
#82991=CARTESIAN_POINT('Ctrl Pts',(-0.169884686431536,0.0973108296489234,
-0.0478138104670284));
#82992=CARTESIAN_POINT('Ctrl Pts',(-0.163167874027577,0.107505371425435,
-0.0485080662530149));
#82993=CARTESIAN_POINT('Ctrl Pts',(-0.15645214632649,0.117698266878054,
-0.0492022099231346));
#82994=CARTESIAN_POINT('Ctrl Pts',(-0.148771856484054,0.127268320790351,
-0.049896353593254));
#82995=CARTESIAN_POINT('Ctrl Pts',(-0.140270093219887,0.136034778450528,
-0.0505904972633736));
#82996=CARTESIAN_POINT('Ctrl Pts',(-0.131768898910346,0.144800649442212,
-0.0512845944800411));
#82997=CARTESIAN_POINT('Ctrl Pts',(-0.122446970559794,0.152762419409819,
-0.0519786916967088));
#82998=CARTESIAN_POINT('Ctrl Pts',(-0.112483994582994,0.159776440574488,
-0.0526727889133763));
#82999=CARTESIAN_POINT('Ctrl Pts',(-0.102498182728351,0.166806538394453,
-0.0533684770522029));
#83000=CARTESIAN_POINT('Ctrl Pts',(-0.0918691449919437,0.172884099581189,
-0.0540641651910295));
#83001=CARTESIAN_POINT('Ctrl Pts',(-0.0808041029838316,0.177909687597327,
-0.0547598533298561));
#83002=CARTESIAN_POINT('Ctrl Pts',(-0.0772902231149733,0.179505642908308,
-0.0549807801500376));
#83003=CARTESIAN_POINT('Ctrl Pts',(-0.0737325233941246,0.180995874483825,
-0.0552017069702189));
#83004=CARTESIAN_POINT('Ctrl Pts',(-0.0701379921819701,0.182378238977905,
-0.0554226337904004));
#83005=CARTESIAN_POINT('Ctrl Pts',(-0.0587992620769335,0.186738823705104,
-0.0561195340088575));
#83006=CARTESIAN_POINT('Ctrl Pts',(-0.0470127009258709,0.190053187710039,
-0.0568164342273145));
#83007=CARTESIAN_POINT('Ctrl Pts',(-0.0349934860263581,0.192241036034773,
-0.0575133344457717));
#83008=CARTESIAN_POINT('Ctrl Pts',(-0.0229993172646902,0.194424325230548,
-0.058208782434688));
#83009=CARTESIAN_POINT('Ctrl Pts',(-0.0107742956381948,0.195485530924792,
-0.0589042304236042));
#83010=CARTESIAN_POINT('Ctrl Pts',(0.00145313166310702,0.195394596671376,
-0.0595996784125205));
#83011=CARTESIAN_POINT('Ctrl Pts',(0.0136788475491207,0.195303675145598,
-0.0602950290628641));
#83012=CARTESIAN_POINT('Ctrl Pts',(0.0259060951035811,0.194060895136054,
-0.0609903797132079));
#83013=CARTESIAN_POINT('Ctrl Pts',(0.0379047371236277,0.191688264908389,
-0.0616857303635516));
#83014=CARTESIAN_POINT('Ctrl Pts',(0.0499027469665529,0.189315759688416,
-0.062381044377685));
#83015=CARTESIAN_POINT('Ctrl Pts',(0.0616713226686245,0.18581371845615,
-0.0630763583918182));
#83016=CARTESIAN_POINT('Ctrl Pts',(0.0729915885107183,0.181255035810545,
-0.0637716724059516));
#83017=CARTESIAN_POINT('Ctrl Pts',(0.0843376302544334,0.176685973182965,
-0.0644685696289843));
#83018=CARTESIAN_POINT('Ctrl Pts',(0.095232538151035,0.171055852766036,
-0.0651654668520171));
#83019=CARTESIAN_POINT('Ctrl Pts',(0.105479553706685,0.164484721934405,
-0.0658623640750498));
#83020=CARTESIAN_POINT('Ctrl Pts',(0.108639866435306,0.162458099812495,
-0.06607729623286));
#83021=CARTESIAN_POINT('Ctrl Pts',(0.111738766308828,0.160342278569007,
-0.06629222839067));
#83022=CARTESIAN_POINT('Ctrl Pts',(0.114771100586274,0.158141564650839,
-0.0665071605484802));
#83023=CARTESIAN_POINT('Ctrl Pts',(0.12460217738225,0.151006669366897,-0.0672039882581008));
#83024=CARTESIAN_POINT('Ctrl Pts',(0.133799720311098,0.142926611734703,
-0.0679008159677215));
#83025=CARTESIAN_POINT('Ctrl Pts',(0.14217924747587,0.134038134824367,-0.0685976436773421));
#83026=CARTESIAN_POINT('Ctrl Pts',(0.150541356185308,0.125168134319085,
-0.0692930228968395));
#83027=CARTESIAN_POINT('Ctrl Pts',(0.158088176868394,0.115493629854552,
-0.0699884021163368));
#83028=CARTESIAN_POINT('Ctrl Pts',(0.164670142831369,0.105189847703552,
-0.0706837813358341));
#83029=CARTESIAN_POINT('Ctrl Pts',(0.17125124987678,0.094887410150733,-0.0713790698114066));
#83030=CARTESIAN_POINT('Ctrl Pts',(0.176867244078257,0.0839565695938618,
-0.0720743582869791));
#83031=CARTESIAN_POINT('Ctrl Pts',(0.18141131068929,0.0726023164506069,
-0.0727696467625515));
#83032=CARTESIAN_POINT('Ctrl Pts',(0.185955162558449,0.0612485998825829,
-0.07346490238043));
#83033=CARTESIAN_POINT('Ctrl Pts',(0.189426887723643,0.0494723325132606,
-0.0741601579983084));
#83034=CARTESIAN_POINT('Ctrl Pts',(0.191768488377404,0.0374967580658035,
-0.0748554136161869));
#83035=CARTESIAN_POINT('Ctrl Pts',(0.194115443834778,0.0254937977149432,
-0.0755522591538872));
#83036=CARTESIAN_POINT('Ctrl Pts',(0.195327011951379,0.0132914905823344,
-0.0762491046915876));
#83037=CARTESIAN_POINT('Ctrl Pts',(0.195396789033291,0.00112019439362784,
-0.0769459502292879));
#83038=CARTESIAN_POINT('Ctrl Pts',(0.195418342183163,-0.00263934618474026,
-0.0771611959217122));
#83039=CARTESIAN_POINT('Ctrl Pts',(0.195331332677064,-0.00639593946438014,
-0.0773764416141365));
#83040=CARTESIAN_POINT('Ctrl Pts',(0.195136572149948,-0.0101428896064249,
-0.0775916873065607));
#83041=CARTESIAN_POINT('Ctrl Pts',(0.194506316991174,-0.0222682144433514,
-0.07828823352187));
#83042=CARTESIAN_POINT('Ctrl Pts',(0.192739361234437,-0.0343772940435297,
-0.0789847797371793));
#83043=CARTESIAN_POINT('Ctrl Pts',(0.189849733125944,-0.0462410946238046,
-0.0796813259524885));
#83044=CARTESIAN_POINT('Ctrl Pts',(0.186966149150865,-0.0580800801099577,
-0.0803764152265944));
#83045=CARTESIAN_POINT('Ctrl Pts',(0.182964686843806,-0.069673945306825,
-0.0810715045007004));
#83046=CARTESIAN_POINT('Ctrl Pts',(0.177910671093355,-0.080801937545532,
-0.0817665937748063));
#83047=CARTESIAN_POINT('Ctrl Pts',(0.172857372559139,-0.0919283506089666,
-0.0824615844086751));
#83048=CARTESIAN_POINT('Ctrl Pts',(0.166752137064087,-0.102588207318666,
-0.0831565750425438));
#83049=CARTESIAN_POINT('Ctrl Pts',(0.159708547162265,-0.112580371128001,
-0.0838515656764126));
#83050=CARTESIAN_POINT('Ctrl Pts',(0.15266533965571,-0.122571992464507,
-0.0845465185793612));
#83051=CARTESIAN_POINT('Ctrl Pts',(0.144684405290716,-0.131895292923133,
-0.0852414714823097));
#83052=CARTESIAN_POINT('Ctrl Pts',(0.135921235042931,-0.140380119192157,
-0.0859364243852583));
#83053=CARTESIAN_POINT('Ctrl Pts',(0.127138037481661,-0.148884336648475,
-0.0866329655307324));
#83054=CARTESIAN_POINT('Ctrl Pts',(0.11756970903862,-0.156545692955718,
-0.0873295066762065));
#83055=CARTESIAN_POINT('Ctrl Pts',(0.107405816032028,-0.163233423913407,
-0.0880260478216805));
#83056=CARTESIAN_POINT('Ctrl Pts',(0.104243418436957,-0.16531424710619,
-0.0882427699026672));
#83057=CARTESIAN_POINT('Ctrl Pts',(0.101023563147127,-0.167301141092061,
-0.088459491983654));
#83058=CARTESIAN_POINT('Ctrl Pts',(0.0977524379413281,-0.169191078005097,
-0.0886762140646408));
#83059=CARTESIAN_POINT('Ctrl Pts',(0.0872362900268904,-0.175266924961737,
-0.0893729411284476));
#83060=CARTESIAN_POINT('Ctrl Pts',(0.0761146347337262,-0.180379874266155,
-0.0900696681922544));
#83061=CARTESIAN_POINT('Ctrl Pts',(0.064587354304539,-0.184417010234794,
-0.0907663952560613));
#83062=CARTESIAN_POINT('Ctrl Pts',(0.0530841161000037,-0.188445726027442,
-0.0914616691697785));
#83063=CARTESIAN_POINT('Ctrl Pts',(0.04117772512102,-0.191402726279639,
-0.0921569430834958));
#83064=CARTESIAN_POINT('Ctrl Pts',(0.0290890283688226,-0.193222639534186,
-0.092852216997213));
#83065=CARTESIAN_POINT('Ctrl Pts',(0.0170019999063227,-0.195042301633244,
-0.0935473949602805));
#83066=CARTESIAN_POINT('Ctrl Pts',(0.00473357266567613,-0.195725013420667,
-0.094242572923348));
#83067=CARTESIAN_POINT('Ctrl Pts',(-0.00748559849745745,-0.195256564076947,
-0.0949377508864155));
#83068=CARTESIAN_POINT('Ctrl Pts',(-0.0197041370974415,-0.194788138983954,
-0.0956328928614478));
#83069=CARTESIAN_POINT('Ctrl Pts',(-0.0318725515042455,-0.193168731601081,
-0.0963280348364801));
#83070=CARTESIAN_POINT('Ctrl Pts',(-0.0437633637775224,-0.190436152006063,
-0.0970231768115124));
#83071=CARTESIAN_POINT('Ctrl Pts',(-0.0556813286728416,-0.18769733257652,
-0.0977199061404512));
#83072=CARTESIAN_POINT('Ctrl Pts',(-0.067319588594467,-0.183840525811168,
-0.09841663546939));
#83073=CARTESIAN_POINT('Ctrl Pts',(-0.0784651523874021,-0.178953569008337,
-0.0991133647983288));
#83074=CARTESIAN_POINT('Ctrl Pts',(-0.0819171724082724,-0.177439973730619,
-0.0993291568064593));
#83075=CARTESIAN_POINT('Ctrl Pts',(-0.0853220936137374,-0.175827899478522,
-0.0995449488145898));
#83076=CARTESIAN_POINT('Ctrl Pts',(-0.0886740841316249,-0.174120839658605,
-0.0997607408227204));
#83077=CARTESIAN_POINT('Ctrl Pts',(-0.0994962453262731,-0.168609464718409,
-0.100457442046678));
#83078=CARTESIAN_POINT('Ctrl Pts',(-0.109840577283525,-0.162065955095513,
-0.101154143270635));
#83079=CARTESIAN_POINT('Ctrl Pts',(-0.119503538064972,-0.154596456589256,
-0.101850844494592));
#83080=CARTESIAN_POINT('Ctrl Pts',(-0.129146346415747,-0.147142535974105,
-0.102546092724645));
#83081=CARTESIAN_POINT('Ctrl Pts',(-0.138109873678078,-0.138766931092801,
-0.103241340954697));
#83082=CARTESIAN_POINT('Ctrl Pts',(-0.146219037064314,-0.12961926245734,
-0.10393658918475));
#83083=CARTESIAN_POINT('Ctrl Pts',(-0.154327088704783,-0.120472847944085,
-0.104631742098031));
#83084=CARTESIAN_POINT('Ctrl Pts',(-0.161580395584372,-0.110555203472283,
-0.105326895011312));
#83085=CARTESIAN_POINT('Ctrl Pts',(-0.167841443444275,-0.100052035774102,
-0.106022047924593));
#83086=CARTESIAN_POINT('Ctrl Pts',(-0.174102170277236,-0.0895494066119433,
-0.106717165194828));
#83087=CARTESIAN_POINT('Ctrl Pts',(-0.179370314350734,-0.0784620792201427,
-0.107412282465063));
#83088=CARTESIAN_POINT('Ctrl Pts',(-0.183553723170007,-0.0670014231970367,
-0.108107399735299));
#83089=CARTESIAN_POINT('Ctrl Pts',(-0.187746690965306,-0.0555145798848333,
-0.108804105329699));
#83090=CARTESIAN_POINT('Ctrl Pts',(-0.190849737003367,-0.0436535486320951,
-0.1095008109241));
#83091=CARTESIAN_POINT('Ctrl Pts',(-0.19282055720892,-0.0316447897392526,
-0.1101975165185));
#83092=CARTESIAN_POINT('Ctrl Pts',(-0.193431336899323,-0.0279231382065417,
-0.110413433539267));
#83093=CARTESIAN_POINT('Ctrl Pts',(-0.193933747380923,-0.0241873459357263,
-0.110629350560034));
#83094=CARTESIAN_POINT('Ctrl Pts',(-0.194327542883033,-0.0204442186703937,
-0.110845267580801));
#83095=CARTESIAN_POINT('Ctrl Pts',(-0.195037475950106,-0.0136961227534052,
-0.111234521983059));
#83096=CARTESIAN_POINT('Ctrl Pts',(-0.195395995378517,-0.00691041122818272,
-0.111623776385318));
#83097=CARTESIAN_POINT('Ctrl Pts',(-0.195399966640838,-0.000114178629661407,
-0.112013030787576));
#83098=CARTESIAN_POINT('',(-0.195399983188327,-8.10555470994038E-5,-0.182013030783586));
#83099=CARTESIAN_POINT('Ctrl Pts',(-0.195399966640887,-0.000114178544617379,
-0.112013030792447));
#83100=CARTESIAN_POINT('Ctrl Pts',(-0.195406979528763,0.0118873587108309,
-0.11270041915692));
#83101=CARTESIAN_POINT('Ctrl Pts',(-0.194303978816564,0.0239328297705788,
-0.113387807521392));
#83102=CARTESIAN_POINT('Ctrl Pts',(-0.192092962998488,0.0357973960849315,
-0.114075195885865));
#83103=CARTESIAN_POINT('Ctrl Pts',(-0.18988411234439,0.0476503438792405,
-0.114761911116969));
#83104=CARTESIAN_POINT('Ctrl Pts',(-0.186569478115567,0.0593218440159743,
-0.115448626348073));
#83105=CARTESIAN_POINT('Ctrl Pts',(-0.182202859798727,0.0705923358528781,
-0.116135341579177));
#83106=CARTESIAN_POINT('Ctrl Pts',(-0.177839396744258,0.0818546837769824,
-0.116821560598666));
#83107=CARTESIAN_POINT('Ctrl Pts',(-0.172425776388526,0.0927157563474014,
-0.117507779618155));
#83108=CARTESIAN_POINT('Ctrl Pts',(-0.166064658076759,0.102974216859605,
-0.118193998637643));
#83109=CARTESIAN_POINT('Ctrl Pts',(-0.159688758125428,0.113256515454729,
-0.118881812257595));
#83110=CARTESIAN_POINT('Ctrl Pts',(-0.152361462661492,0.122932650620025,
-0.119569625877548));
#83111=CARTESIAN_POINT('Ctrl Pts',(-0.14422923316195,0.131829770164087,
-0.1202574394975));
#83112=CARTESIAN_POINT('Ctrl Pts',(-0.137638313286628,0.139040609705612,
-0.120814891111293));
#83113=CARTESIAN_POINT('Ctrl Pts',(-0.130519651799363,0.145740203779063,
-0.121372342725087));
#83114=CARTESIAN_POINT('Ctrl Pts',(-0.122967811914694,0.151855448479508,
-0.121929794338881));
#83115=CARTESIAN_POINT('Ctrl Pts',(-0.113529653954175,0.159498174799379,
-0.122626487656891));
#83116=CARTESIAN_POINT('Ctrl Pts',(-0.103343136437121,0.16628445122242,
-0.1233231809749));
#83117=CARTESIAN_POINT('Ctrl Pts',(-0.09258803740114,0.172071541314086,
-0.12401987429291));
#83118=CARTESIAN_POINT('Ctrl Pts',(-0.0818553769234864,0.177846557694655,
-0.124715114087006));
#83119=CARTESIAN_POINT('Ctrl Pts',(-0.0705572173752286,0.182626050012364,
-0.125410353881101));
#83120=CARTESIAN_POINT('Ctrl Pts',(-0.058901470050085,0.186310968077403,
-0.126105593675196));
#83121=CARTESIAN_POINT('Ctrl Pts',(-0.0472473315871257,0.189995377507074,
-0.126800737504187));
#83122=CARTESIAN_POINT('Ctrl Pts',(-0.0352365226550576,0.192585206048322,
-0.127495881333177));
#83123=CARTESIAN_POINT('Ctrl Pts',(-0.0230946316147195,0.194030404809608,
-0.128191025162168));
#83124=CARTESIAN_POINT('Ctrl Pts',(-0.0109533698761371,0.195475528667725,
-0.128886132962567));
#83125=CARTESIAN_POINT('Ctrl Pts',(0.00131808846455855,0.195776063967537,
-0.129581240762965));
#83126=CARTESIAN_POINT('Ctrl Pts',(0.01348917058184,0.194933840769154,-0.130276348563364));
#83127=CARTESIAN_POINT('Ctrl Pts',(0.0256880566690686,0.194089693571881,
-0.130973044288009));
#83128=CARTESIAN_POINT('Ctrl Pts',(0.0377852410819525,0.192097701857036,
-0.131669740012654));
#83129=CARTESIAN_POINT('Ctrl Pts',(0.0495566499006659,0.189011371220418,
-0.132366435737299));
#83130=CARTESIAN_POINT('Ctrl Pts',(0.0532055519806167,0.18805467024666,
-0.132582397523853));
#83131=CARTESIAN_POINT('Ctrl Pts',(0.0568232602525872,0.186993179440627,
-0.132798359310407));
#83132=CARTESIAN_POINT('Ctrl Pts',(0.0604034538302661,0.185829445366914,
-0.133014321096962));
#83133=CARTESIAN_POINT('Ctrl Pts',(0.0719530707618956,0.182075267703038,
-0.133711008539261));
#83134=CARTESIAN_POINT('Ctrl Pts',(0.0831918879570605,0.177227057516715,
-0.134407695981561));
#83135=CARTESIAN_POINT('Ctrl Pts',(0.0939022926886606,0.171357869465669,
-0.135104383423861));
#83136=CARTESIAN_POINT('Ctrl Pts',(0.104590351401938,0.165500926795354,
-0.135799617308547));
#83137=CARTESIAN_POINT('Ctrl Pts',(0.114751390751995,0.158627585957298,
-0.136494851193232));
#83138=CARTESIAN_POINT('Ctrl Pts',(0.124189118482288,0.15085828731161,-0.137190085077917));
#83139=CARTESIAN_POINT('Ctrl Pts',(0.133625544082522,0.143090060601624,
-0.137885223040686));
#83140=CARTESIAN_POINT('Ctrl Pts',(0.142338152868517,0.134426641736287,
-0.138580361003454));
#83141=CARTESIAN_POINT('Ctrl Pts',(0.150162125068484,0.125029981184182,
-0.139275498966222));
#83142=CARTESIAN_POINT('Ctrl Pts',(0.157985691976748,0.115633807391036,
-0.139970600919961));
#83143=CARTESIAN_POINT('Ctrl Pts',(0.164920174608912,0.105505157029631,
-0.140665702873699));
#83144=CARTESIAN_POINT('Ctrl Pts',(0.170841551236229,0.0948384118972837,
-0.141360804827437));
#83145=CARTESIAN_POINT('Ctrl Pts',(0.176776456107866,0.0841472970375365,
-0.142057494842474));
#83146=CARTESIAN_POINT('Ctrl Pts',(0.181693267050085,0.0729164293198139,
-0.142754184857511));
#83147=CARTESIAN_POINT('Ctrl Pts',(0.185514843110899,0.0613628795407983,
-0.143450874872548));
#83148=CARTESIAN_POINT('Ctrl Pts',(0.186699625431348,0.0577809957057574,
-0.143666865866713));
#83149=CARTESIAN_POINT('Ctrl Pts',(0.187779502715479,0.0541682031150062,
-0.143882856860877));
#83150=CARTESIAN_POINT('Ctrl Pts',(0.188753168329718,0.0505311927970559,
-0.144098847855041));
#83151=CARTESIAN_POINT('Ctrl Pts',(0.191893746382104,0.0387999427520509,
-0.144795531157671));
#83152=CARTESIAN_POINT('Ctrl Pts',(0.193947498709438,0.0267336131564428,
-0.145492214460302));
#83153=CARTESIAN_POINT('Ctrl Pts',(0.194857195170143,0.0145545006930803,
-0.146188897762932));
#83154=CARTESIAN_POINT('Ctrl Pts',(0.195764993449915,0.00240080127686617,
-0.146884127359828));
#83155=CARTESIAN_POINT('Ctrl Pts',(0.195533336034077,-0.00986435549050084,
-0.147579356956725));
#83156=CARTESIAN_POINT('Ctrl Pts',(0.194156346448908,-0.0220107504100111,
-0.148274586553622));
#83157=CARTESIAN_POINT('Ctrl Pts',(0.19277954714799,-0.034155466836306,
-0.148969720077719));
#83158=CARTESIAN_POINT('Ctrl Pts',(0.190257783232272,-0.0461805807952212,
-0.149664853601817));
#83159=CARTESIAN_POINT('Ctrl Pts',(0.186637132307281,-0.0578596650881648,
-0.150359987125914));
#83160=CARTESIAN_POINT('Ctrl Pts',(0.18301666941663,-0.0695381428413006,
-0.151055084549052));
#83161=CARTESIAN_POINT('Ctrl Pts',(0.178297717738639,-0.0808697988692114,
-0.151750181972189));
#83162=CARTESIAN_POINT('Ctrl Pts',(0.172575772659037,-0.091644763577285,
-0.152445279395327));
#83163=CARTESIAN_POINT('Ctrl Pts',(0.166840755320049,-0.102444344588305,
-0.153141964826333));
#83164=CARTESIAN_POINT('Ctrl Pts',(0.160098637886572,-0.112683953777672,
-0.15383865025734));
#83165=CARTESIAN_POINT('Ctrl Pts',(0.152489474724976,-0.122180686272835,
-0.154535335688346));
#83166=CARTESIAN_POINT('Ctrl Pts',(0.150130191900801,-0.125125225295825,
-0.154751348663271));
#83167=CARTESIAN_POINT('Ctrl Pts',(0.147687841662342,-0.127998594515703,
-0.154967361638196));
#83168=CARTESIAN_POINT('Ctrl Pts',(0.14516732599168,-0.130796052939014,
-0.155183374613122));
#83169=CARTESIAN_POINT('Ctrl Pts',(0.137038132673913,-0.139818444898807,
-0.155880061903247));
#83170=CARTESIAN_POINT('Ctrl Pts',(0.128036060866306,-0.148111738733537,
-0.156576749193372));
#83171=CARTESIAN_POINT('Ctrl Pts',(0.118316396013281,-0.155506882273514,
-0.157273436483497));
#83172=CARTESIAN_POINT('Ctrl Pts',(0.108617010874177,-0.162886596125568,
-0.157968670161883));
#83173=CARTESIAN_POINT('Ctrl Pts',(0.0982036492653511,-0.169371295979603,
-0.158663903840268));
#83174=CARTESIAN_POINT('Ctrl Pts',(0.0872662056366348,-0.174830687677491,
-0.159359137518654));
#83175=CARTESIAN_POINT('Ctrl Pts',(0.0763302722588966,-0.180289325538201,
-0.160054275198616));
#83176=CARTESIAN_POINT('Ctrl Pts',(0.0648711619465925,-0.184722505559066,
-0.160749412878579));
#83177=CARTESIAN_POINT('Ctrl Pts',(0.0531038798602043,-0.188045574113812,
-0.161444550558541));
#83178=CARTESIAN_POINT('Ctrl Pts',(0.0413372080917684,-0.191368470315385,
-0.162139652184723));
#83179=CARTESIAN_POINT('Ctrl Pts',(0.0292632456717851,-0.193581157594719,
-0.162834753810905));
#83180=CARTESIAN_POINT('Ctrl Pts',(0.0171100205517335,-0.194649446946862,
-0.163529855437087));
#83181=CARTESIAN_POINT('Ctrl Pts',(0.0049290306725261,-0.195720176869,-0.164226545063906));
#83182=CARTESIAN_POINT('Ctrl Pts',(-0.00733070674353389,-0.195641278068855,
-0.164923234690725));
#83183=CARTESIAN_POINT('Ctrl Pts',(-0.0194395154429373,-0.194430618060386,
-0.165619924317545));
#83184=CARTESIAN_POINT('Ctrl Pts',(-0.0231935688416982,-0.194055281193452,
-0.165835916668764));
#83185=CARTESIAN_POINT('Ctrl Pts',(-0.0269331667609787,-0.193571538690036,
-0.166051909019983));
#83186=CARTESIAN_POINT('Ctrl Pts',(-0.0306516653744782,-0.192980919807558,
-0.166267901371201));
#83187=CARTESIAN_POINT('Ctrl Pts',(-0.0426457312406904,-0.191075870884705,
-0.166964587522357));
#83188=CARTESIAN_POINT('Ctrl Pts',(-0.0545036084208412,-0.188041687468554,
-0.167661273673513));
#83189=CARTESIAN_POINT('Ctrl Pts',(-0.0659989479753539,-0.183916554084037,
-0.168357959824668));
#83190=CARTESIAN_POINT('Ctrl Pts',(-0.0774703026853929,-0.179800027725193,
-0.16905319235117));
#83191=CARTESIAN_POINT('Ctrl Pts',(-0.0885797808718527,-0.174597292625729,
-0.169748424877671));
#83192=CARTESIAN_POINT('Ctrl Pts',(-0.0991146946313072,-0.16839666655888,
-0.170443657404173));
#83193=CARTESIAN_POINT('Ctrl Pts',(-0.109648153704876,-0.162196896689189,
-0.171138793931318));
#83194=CARTESIAN_POINT('Ctrl Pts',(-0.119606429941285,-0.154999913465743,
-0.171833930458463));
#83195=CARTESIAN_POINT('Ctrl Pts',(-0.128801441376143,-0.146939949297079,
-0.172529066985608));
#83196=CARTESIAN_POINT('Ctrl Pts',(-0.13799597588318,-0.138880403183484,
-0.173224167457339));
#83197=CARTESIAN_POINT('Ctrl Pts',(-0.146426684035344,-0.129958562083755,
-0.173919267929069));
#83198=CARTESIAN_POINT('Ctrl Pts',(-0.153940718427832,-0.12034706149268,
-0.1746143684008));
#83199=CARTESIAN_POINT('Ctrl Pts',(-0.161471919307272,-0.110713602564596,
-0.175311056892035));
#83200=CARTESIAN_POINT('Ctrl Pts',(-0.168081778633305,-0.10038806776869,
-0.176007745383271));
#83201=CARTESIAN_POINT('Ctrl Pts',(-0.173660212725031,-0.0895728224200685,
-0.176704433874507));
#83202=CARTESIAN_POINT('Ctrl Pts',(-0.175389724688914,-0.086219713659579,
-0.176920431959431));
#83203=CARTESIAN_POINT('Ctrl Pts',(-0.177020436780129,-0.082819694360548,
-0.177136430044356));
#83204=CARTESIAN_POINT('Ctrl Pts',(-0.178550013560408,-0.0793791701744119,
-0.177352428129281));
#83205=CARTESIAN_POINT('Ctrl Pts',(-0.184050640726163,-0.0670064399874064,
-0.178129195238332));
#83206=CARTESIAN_POINT('Ctrl Pts',(-0.188273338435027,-0.0540322449477344,
-0.178905962347383));
#83207=CARTESIAN_POINT('Ctrl Pts',(-0.1911093419295,-0.0407232050221174,
-0.179682729456434));
#83208=CARTESIAN_POINT('Ctrl Pts',(-0.193945345423973,-0.0274141650965003,
-0.180459496565485));
#83209=CARTESIAN_POINT('Ctrl Pts',(-0.195394304400981,-0.0137708644685566,
-0.181236263674536));
#83210=CARTESIAN_POINT('Ctrl Pts',(-0.195399983188326,-8.10555470994277E-5,
-0.182013030783586));
#83211=CARTESIAN_POINT('',(-0.195399922115002,0.00017446332273763,-0.252013030791491));
#83212=CARTESIAN_POINT('Ctrl Pts',(-0.195399983188356,-8.105547677933E-5,
-0.182013030787576));
#83213=CARTESIAN_POINT('Ctrl Pts',(-0.19540516234588,0.0124043105133673,
-0.182721457157962));
#83214=CARTESIAN_POINT('Ctrl Pts',(-0.194209352567215,0.0248838378421996,
-0.183429883528347));
#83215=CARTESIAN_POINT('Ctrl Pts',(-0.191841856825415,0.0371195631679168,
-0.184138309898733));
#83216=CARTESIAN_POINT('Ctrl Pts',(-0.189447577492252,0.0494937118332676,
-0.184854750730171));
#83217=CARTESIAN_POINT('Ctrl Pts',(-0.185855101489844,0.0616176612605396,
-0.185571191561609));
#83218=CARTESIAN_POINT('Ctrl Pts',(-0.18114698418511,0.0732593346996781,
-0.186287632393047));
#83219=CARTESIAN_POINT('Ctrl Pts',(-0.176438866880377,0.0849010081388166,
-0.187004073224486));
#83220=CARTESIAN_POINT('Ctrl Pts',(-0.17061556133838,0.0960596672418057,
-0.187720514055924));
#83221=CARTESIAN_POINT('Ctrl Pts',(-0.163806866578169,0.10652920004319,
-0.188436954887362));
#83222=CARTESIAN_POINT('Ctrl Pts',(-0.157185909241894,0.116710054443329,
-0.189133641160719));
#83223=CARTESIAN_POINT('Ctrl Pts',(-0.149588953930905,0.126307024607797,
-0.189830327434076));
#83224=CARTESIAN_POINT('Ctrl Pts',(-0.141142989352494,0.135128888682775,
-0.190527013707433));
#83225=CARTESIAN_POINT('Ctrl Pts',(-0.132714647195745,0.143932346025504,
-0.191222246351763));
#83226=CARTESIAN_POINT('Ctrl Pts',(-0.123441357672301,0.15196323053721,
-0.191917478996092));
#83227=CARTESIAN_POINT('Ctrl Pts',(-0.113490345006027,0.15906319998797,
-0.192612711640422));
#83228=CARTESIAN_POINT('Ctrl Pts',(-0.103540706517675,0.166162188973566,
-0.193307848277101));
#83229=CARTESIAN_POINT('Ctrl Pts',(-0.0929142155251427,0.172329973771519,
-0.194002984913779));
#83230=CARTESIAN_POINT('Ctrl Pts',(-0.0818100244084474,0.177449372797678,
-0.194698121550458));
#83231=CARTESIAN_POINT('Ctrl Pts',(-0.0707064093203941,0.182568506255599,
-0.195393222127003));
#83232=CARTESIAN_POINT('Ctrl Pts',(-0.059125949223413,0.186639020139161,
-0.196088322703549));
#83233=CARTESIAN_POINT('Ctrl Pts',(-0.0472885380461972,0.189591545617027,
-0.196783423280094));
#83234=CARTESIAN_POINT('Ctrl Pts',(-0.0354240833959644,0.19255081636562,
-0.197480111867177));
#83235=CARTESIAN_POINT('Ctrl Pts',(-0.0233023698885466,0.194386851599335,
-0.19817680045426));
#83236=CARTESIAN_POINT('Ctrl Pts',(-0.0111530464764509,0.195081443387868,
-0.198873489041343));
#83237=CARTESIAN_POINT('Ctrl Pts',(-0.00738633642272806,0.195296790842567,
-0.199089486576042));
#83238=CARTESIAN_POINT('Ctrl Pts',(-0.00361698042405993,0.195402799863082,
-0.199305484110742));
#83239=CARTESIAN_POINT('Ctrl Pts',(0.000148219910908216,0.195399943784173,
-0.199521481645441));
#83240=CARTESIAN_POINT('Ctrl Pts',(0.0122926299414716,0.195390731686473,
-0.200218167716198));
#83241=CARTESIAN_POINT('Ctrl Pts',(0.0244787985054029,0.194244968897385,
-0.200914853786955));
#83242=CARTESIAN_POINT('Ctrl Pts',(0.036477190826623,0.191965034705277,
-0.201611539857711));
#83243=CARTESIAN_POINT('Ctrl Pts',(0.0484505485620488,0.1896898575845,-0.202306772296453));
#83244=CARTESIAN_POINT('Ctrl Pts',(0.0602360428669622,0.186285295386219,
-0.203002004735195));
#83245=CARTESIAN_POINT('Ctrl Pts',(0.0716098058136541,0.181805378664468,
-0.203697237173936));
#83246=CARTESIAN_POINT('Ctrl Pts',(0.0829819980891168,0.177326080601322,
-0.204392373603855));
#83247=CARTESIAN_POINT('Ctrl Pts',(0.0939417424025054,0.171772000804235,
-0.205087510033774));
#83248=CARTESIAN_POINT('Ctrl Pts',(0.104282306981401,0.165246362896848,
-0.205782646463693));
#83249=CARTESIAN_POINT('Ctrl Pts',(0.114622335131479,0.15872106351452,-0.206477746832601));
#83250=CARTESIAN_POINT('Ctrl Pts',(0.124342521798727,0.151224795917388,
-0.207172847201508));
#83251=CARTESIAN_POINT('Ctrl Pts',(0.133264942347688,0.142904216666505,
-0.207867947570416));
#83252=CARTESIAN_POINT('Ctrl Pts',(0.142207746888664,0.134564628378771,
-0.208564635952385));
#83253=CARTESIAN_POINT('Ctrl Pts',(0.150348552004181,0.12539761298159,-0.209261324334354));
#83254=CARTESIAN_POINT('Ctrl Pts',(0.157547031093136,0.115585868486327,
-0.209958012716324));
#83255=CARTESIAN_POINT('Ctrl Pts',(0.15977881961569,0.112543873298155,-0.210174011278723));
#83256=CARTESIAN_POINT('Ctrl Pts',(0.16192034282866,0.109440118121617,-0.210390009841122));
#83257=CARTESIAN_POINT('Ctrl Pts',(0.163968293874172,0.106280565504674,
-0.210606008403521));
#83258=CARTESIAN_POINT('Ctrl Pts',(0.170573795625582,0.0960896820894549,
-0.211302694432885));
#83259=CARTESIAN_POINT('Ctrl Pts',(0.176248779215107,0.085244866852711,
-0.21199938046225));
#83260=CARTESIAN_POINT('Ctrl Pts',(0.180870247225192,0.0739399328421249,
-0.212696066491614));
#83261=CARTESIAN_POINT('Ctrl Pts',(0.185482072550167,0.062658586557045,
-0.213391298886768));
#83262=CARTESIAN_POINT('Ctrl Pts',(0.189044349253176,0.0509198010178098,
-0.214086531281921));
#83263=CARTESIAN_POINT('Ctrl Pts',(0.191480487199185,0.0389407629863966,
-0.214781763677075));
#83264=CARTESIAN_POINT('Ctrl Pts',(0.193916288715316,0.0269633792563398,
-0.215476900060855));
#83265=CARTESIAN_POINT('Ctrl Pts',(0.195226041671566,0.0147466559843934,
-0.216172036444636));
#83266=CARTESIAN_POINT('Ctrl Pts',(0.195383747059877,0.00252019539758848,
-0.216867172828416));
#83267=CARTESIAN_POINT('Ctrl Pts',(0.19554144426669,-0.00970563090046064,
-0.217562273149659));
#83268=CARTESIAN_POINT('Ctrl Pts',(0.194547228318338,-0.021940318258623,
-0.218257373470902));
#83269=CARTESIAN_POINT('Ctrl Pts',(0.192427215569999,-0.0339547744503923,
-0.218952473792144));
#83270=CARTESIAN_POINT('Ctrl Pts',(0.190302359484847,-0.0459966786176576,
-0.219649162125053));
#83271=CARTESIAN_POINT('Ctrl Pts',(0.187046788337536,-0.0578164975414096,
-0.220345850457961));
#83272=CARTESIAN_POINT('Ctrl Pts',(0.18273732146997,-0.0691970472056503,
-0.221042538790869));
#83273=CARTESIAN_POINT('Ctrl Pts',(0.181401229582072,-0.0727254326309214,
-0.221258537581113));
#83274=CARTESIAN_POINT('Ctrl Pts',(0.179964183686421,-0.076211741199239,
-0.221474536371357));
#83275=CARTESIAN_POINT('Ctrl Pts',(0.178429384007929,-0.0796499524328228,
-0.221690535161602));
#83276=CARTESIAN_POINT('Ctrl Pts',(0.173479015467716,-0.0907396164221063,
-0.222387221270501));
#83277=CARTESIAN_POINT('Ctrl Pts',(0.16747346226795,-0.101404925766471,
-0.2230839073794));
#83278=CARTESIAN_POINT('Ctrl Pts',(0.160508302936004,-0.111437178215369,
-0.2237805934883));
#83279=CARTESIAN_POINT('Ctrl Pts',(0.153557676374664,-0.121448498418995,
-0.224475825965068));
#83280=CARTESIAN_POINT('Ctrl Pts',(0.145651851269864,-0.130828629795998,
-0.225171058441836));
#83281=CARTESIAN_POINT('Ctrl Pts',(0.136931281400909,-0.139395065098822,
-0.225866290918604));
#83282=CARTESIAN_POINT('Ctrl Pts',(0.128211915817396,-0.147960317401744,
-0.226561427385781));
#83283=CARTESIAN_POINT('Ctrl Pts',(0.11867862030011,-0.155711452131251,
-0.227256563852957));
#83284=CARTESIAN_POINT('Ctrl Pts',(0.108509811188828,-0.162501633455682,
-0.227951700320134));
#83285=CARTESIAN_POINT('Ctrl Pts',(0.0983415296023409,-0.169291462527557,
-0.228646800725888));
#83286=CARTESIAN_POINT('Ctrl Pts',(0.0875385425542467,-0.175119973763597,
-0.229341901131642));
#83287=CARTESIAN_POINT('Ctrl Pts',(0.076307218005659,-0.179884319717525,
-0.230037001537397));
#83288=CARTESIAN_POINT('Ctrl Pts',(0.0650502346092214,-0.184659550196018,
-0.230733689954919));
#83289=CARTESIAN_POINT('Ctrl Pts',(0.0533637905445501,-0.188365480666791,
-0.231430378372441));
#83290=CARTESIAN_POINT('Ctrl Pts',(0.0414718762791761,-0.190948274351681,
-0.232127066789963));
#83291=CARTESIAN_POINT('Ctrl Pts',(0.0377849566877756,-0.19174903295327,
-0.232343065166536));
#83292=CARTESIAN_POINT('Ctrl Pts',(0.0340783538329179,-0.192442206005216,
-0.232559063543108));
#83293=CARTESIAN_POINT('Ctrl Pts',(0.0303588599030374,-0.193027199185472,
-0.232775061919681));
#83294=CARTESIAN_POINT('Ctrl Pts',(0.0183619196136292,-0.19491404948972,
-0.233471747994509));
#83295=CARTESIAN_POINT('Ctrl Pts',(0.00614629785945884,-0.195684804064974,
-0.234168434069336));
#83296=CARTESIAN_POINT('Ctrl Pts',(-0.00606091356201013,-0.195305978727723,
-0.234865120144164));
#83297=CARTESIAN_POINT('Ctrl Pts',(-0.0182426546855573,-0.194927943808026,
-0.235560352586276));
#83298=CARTESIAN_POINT('Ctrl Pts',(-0.0304151521306216,-0.19340504300487,
-0.236255585028388));
#83299=CARTESIAN_POINT('Ctrl Pts',(-0.0423488478193519,-0.190755694773114,
-0.2369508174705));
#83300=CARTESIAN_POINT('Ctrl Pts',(-0.0542808954937715,-0.188106712409896,
-0.237645953902706));
#83301=CARTESIAN_POINT('Ctrl Pts',(-0.065973344173134,-0.184331736513773,
-0.238341090334911));
#83302=CARTESIAN_POINT('Ctrl Pts',(-0.0772058819424711,-0.179500450677666,
-0.239036226767116));
#83303=CARTESIAN_POINT('Ctrl Pts',(-0.0884378370006978,-0.174669415474497,
-0.239731327137682));
#83304=CARTESIAN_POINT('Ctrl Pts',(-0.0992091354226222,-0.168782549685527,
-0.240426427508248));
#83305=CARTESIAN_POINT('Ctrl Pts',(-0.109321138589207,-0.16195693457694,
-0.241121527878815));
#83306=CARTESIAN_POINT('Ctrl Pts',(-0.119456243431465,-0.155115725807641,
-0.241818216261475));
#83307=CARTESIAN_POINT('Ctrl Pts',(-0.128928357995219,-0.147332029574057,
-0.242514904644135));
#83308=CARTESIAN_POINT('Ctrl Pts',(-0.13757035400327,-0.138764396368143,
-0.243211593026795));
#83309=CARTESIAN_POINT('Ctrl Pts',(-0.140249684757291,-0.136108120767414,
-0.243427591577117));
#83310=CARTESIAN_POINT('Ctrl Pts',(-0.142849498779866,-0.133376750497312,
-0.243643590127439));
#83311=CARTESIAN_POINT('Ctrl Pts',(-0.145365598904999,-0.130575658738492,
-0.243859588677762));
#83312=CARTESIAN_POINT('Ctrl Pts',(-0.15340020980029,-0.121630989907819,
-0.244549332415879));
#83313=CARTESIAN_POINT('Ctrl Pts',(-0.160637251305879,-0.111907083313971,
-0.245239076153997));
#83314=CARTESIAN_POINT('Ctrl Pts',(-0.166925987723204,-0.101572016927069,
-0.245928819892114));
#83315=CARTESIAN_POINT('Ctrl Pts',(-0.173201884280739,-0.0912580518862106,
-0.246617155364358));
#83316=CARTESIAN_POINT('Ctrl Pts',(-0.178532788468517,-0.0803361179447198,
-0.247305490836601));
#83317=CARTESIAN_POINT('Ctrl Pts',(-0.182809932098231,-0.0690049905893792,
-0.247993826308844));
#83318=CARTESIAN_POINT('Ctrl Pts',(-0.187088666891204,-0.0576696478802656,
-0.248682417852478));
#83319=CARTESIAN_POINT('Ctrl Pts',(-0.190312494068741,-0.0459256273125695,
-0.249371009396111));
#83320=CARTESIAN_POINT('Ctrl Pts',(-0.19242059217681,-0.033992288924488,
-0.250059600939744));
#83321=CARTESIAN_POINT('Ctrl Pts',(-0.194414043788067,-0.0227079314525326,
-0.250710744222355));
#83322=CARTESIAN_POINT('Ctrl Pts',(-0.195410127008499,-0.0112550804263115,
-0.251361887504965));
#83323=CARTESIAN_POINT('Ctrl Pts',(-0.195399922115064,0.000174463254022285,
-0.252013030787576));
#83324=CARTESIAN_POINT('',(-0.195399991113071,-5.89322641794126E-5,-0.322013030791099));
#83325=CARTESIAN_POINT('Ctrl Pts',(-0.195399922115002,0.00017446332273629,
-0.252013030791491));
#83326=CARTESIAN_POINT('Ctrl Pts',(-0.19538611251111,0.0156412988881714,
-0.252894179362555));
#83327=CARTESIAN_POINT('Ctrl Pts',(-0.193531985236505,0.031025722314354,
-0.253775327933618));
#83328=CARTESIAN_POINT('Ctrl Pts',(-0.189918199616712,0.0459590845681982,
-0.254656476504681));
#83329=CARTESIAN_POINT('Ctrl Pts',(-0.18952497594356,0.0475840153681317,
-0.254752356148401));
#83330=CARTESIAN_POINT('Ctrl Pts',(-0.189110963346523,0.0492036272310654,
-0.254848235792121));
#83331=CARTESIAN_POINT('Ctrl Pts',(-0.188676298791606,0.0508174603291092,
-0.254944115435841));
#83332=CARTESIAN_POINT('Ctrl Pts',(-0.185517914649659,0.0625439855471211,
-0.255640801519016));
#83333=CARTESIAN_POINT('Ctrl Pts',(-0.181251035015882,0.0740160916859001,
-0.256337487602192));
#83334=CARTESIAN_POINT('Ctrl Pts',(-0.175937484489621,0.0850127140577487,
-0.257034173685368));
#83335=CARTESIAN_POINT('Ctrl Pts',(-0.17063502066475,0.0959863920220958,
-0.257729406135886));
#83336=CARTESIAN_POINT('Ctrl Pts',(-0.164290531131562,0.106485743283834,
-0.258424638586405));
#83337=CARTESIAN_POINT('Ctrl Pts',(-0.157014254994016,0.116308571174588,
-0.259119871036924));
#83338=CARTESIAN_POINT('Ctrl Pts',(-0.149738983692955,0.126130042556097,
-0.25981500747749));
#83339=CARTESIAN_POINT('Ctrl Pts',(-0.141532664824672,0.135274447027259,
-0.260510143918056));
#83340=CARTESIAN_POINT('Ctrl Pts',(-0.132548603495651,0.143568895347678,
-0.261205280358622));
#83341=CARTESIAN_POINT('Ctrl Pts',(-0.123565008233616,0.15186291337623,
-0.26190038073753));
#83342=CARTESIAN_POINT('Ctrl Pts',(-0.113804411841073,0.159306489128976,
-0.262595481116438));
#83343=CARTESIAN_POINT('Ctrl Pts',(-0.103454595656893,0.16576581866437,
-0.263290581495346));
#83344=CARTESIAN_POINT('Ctrl Pts',(-0.0930811344972744,0.172239905050078,
-0.263987269886165));
#83345=CARTESIAN_POINT('Ctrl Pts',(-0.0821165425315173,0.17772484879732,
-0.264683958276985));
#83346=CARTESIAN_POINT('Ctrl Pts',(-0.0707736589292538,0.182132504517359,
-0.265380646667805));
#83347=CARTESIAN_POINT('Ctrl Pts',(-0.067256956232909,0.183499036635534,
-0.265596645176511));
#83348=CARTESIAN_POINT('Ctrl Pts',(-0.0637040156330268,0.184762375124595,
-0.265812643685216));
#83349=CARTESIAN_POINT('Ctrl Pts',(-0.0601214532647579,0.185920872570385,
-0.266028642193922));
#83350=CARTESIAN_POINT('Ctrl Pts',(-0.048566182168939,0.189657514301592,
-0.266725328271599));
#83351=CARTESIAN_POINT('Ctrl Pts',(-0.0366206693845789,0.192325885138425,
-0.267422014349276));
#83352=CARTESIAN_POINT('Ctrl Pts',(-0.024503994786874,0.193857458560368,
-0.268118700426954));
#83353=CARTESIAN_POINT('Ctrl Pts',(-0.012412601583059,0.19538583636039,
-0.26881393287187));
#83354=CARTESIAN_POINT('Ctrl Pts',(-0.000151605633977037,0.195781942874476,
-0.269509165316787));
#83355=CARTESIAN_POINT('Ctrl Pts',(0.0120493742582722,0.195028132791103,
-0.270204397761704));
#83356=CARTESIAN_POINT('Ctrl Pts',(0.0242486692229536,0.194274426807188,
-0.270899534196601));
#83357=CARTESIAN_POINT('Ctrl Pts',(0.0363870898065443,0.192371128093905,
-0.271594670631498));
#83358=CARTESIAN_POINT('Ctrl Pts',(0.0482361466365246,0.189352671377141,
-0.272289807066396));
#83359=CARTESIAN_POINT('Ctrl Pts',(0.0600845887711323,0.186334371249329,
-0.272984907439592));
#83360=CARTESIAN_POINT('Ctrl Pts',(0.0716428557342279,0.182201270174255,
-0.273680007812788));
#83361=CARTESIAN_POINT('Ctrl Pts',(0.0826964661184239,0.177038002958473,
-0.274375108185984));
#83362=CARTESIAN_POINT('Ctrl Pts',(0.0937753293525448,0.171862939849079,
-0.275071796571132));
#83363=CARTESIAN_POINT('Ctrl Pts',(0.104346469879209,0.16565344143362,-0.27576848495628));
#83364=CARTESIAN_POINT('Ctrl Pts',(0.114220056217435,0.158540022573753,
-0.276465173341428));
#83365=CARTESIAN_POINT('Ctrl Pts',(0.117281224234673,0.156334606065393,
-0.276681171878286));
#83366=CARTESIAN_POINT('Ctrl Pts',(0.120275574076283,0.154042601749538,
-0.276897170415144));
#83367=CARTESIAN_POINT('Ctrl Pts',(0.123198121195366,0.151668661673834,
-0.277113168952002));
#83368=CARTESIAN_POINT('Ctrl Pts',(0.132624564167303,0.144011707027558,
-0.277809855029848));
#83369=CARTESIAN_POINT('Ctrl Pts',(0.141367523257338,0.135445719343915,
-0.278506541107693));
#83370=CARTESIAN_POINT('Ctrl Pts',(0.149250223522671,0.12611713118539,-0.279203227185539));
#83371=CARTESIAN_POINT('Ctrl Pts',(0.157116476564654,0.116808007089663,
-0.279898459630601));
#83372=CARTESIAN_POINT('Ctrl Pts',(0.164125417987913,0.106740054854432,
-0.280593692075663));
#83373=CARTESIAN_POINT('Ctrl Pts',(0.170137209426213,0.096096253666108,
-0.281288924520725));
#83374=CARTESIAN_POINT('Ctrl Pts',(0.176148170649486,0.0854539223630562,
-0.281984060955733));
#83375=CARTESIAN_POINT('Ctrl Pts',(0.18116178612565,0.0742366383704422,
-0.28267919739074));
#83376=CARTESIAN_POINT('Ctrl Pts',(0.185082513551193,0.0626547937317849,
-0.283374333825748));
#83377=CARTESIAN_POINT('Ctrl Pts',(0.189003037580431,0.0510735499266331,
-0.284069434199034));
#83378=CARTESIAN_POINT('Ctrl Pts',(0.191830531175522,0.0391286204697831,
-0.28476453457232));
#83379=CARTESIAN_POINT('Ctrl Pts',(0.193519184317751,0.0270459849329323,
-0.285459634945605));
#83380=CARTESIAN_POINT('Ctrl Pts',(0.195211695321984,0.0149357456571146,
-0.286156323330811));
#83381=CARTESIAN_POINT('Ctrl Pts',(0.195760115543239,0.00268804718140895,
-0.286853011716017));
#83382=CARTESIAN_POINT('Ctrl Pts',(0.195170538988722,-0.00946682158127442,
-0.287549700101223));
#83383=CARTESIAN_POINT('Ctrl Pts',(0.194987748984599,-0.0132352694515691,
-0.287765698637509));
#83384=CARTESIAN_POINT('Ctrl Pts',(0.194695949500409,-0.0169948263072403,
-0.287981697173795));
#83385=CARTESIAN_POINT('Ctrl Pts',(0.194296328011977,-0.020738778195985,
-0.288197695710081));
#83386=CARTESIAN_POINT('Ctrl Pts',(0.193007380722087,-0.0328145968898343,
-0.288894381789347));
#83387=CARTESIAN_POINT('Ctrl Pts',(0.190583810546708,-0.0448121710990928,
-0.289591067868612));
#83388=CARTESIAN_POINT('Ctrl Pts',(0.187052172057487,-0.0565034948350653,
-0.290287753947877));
#83389=CARTESIAN_POINT('Ctrl Pts',(0.18352790231797,-0.0681704246704228,
-0.290982986394401));
#83390=CARTESIAN_POINT('Ctrl Pts',(0.178900333129847,-0.0795315217171349,
-0.291678218840924));
#83391=CARTESIAN_POINT('Ctrl Pts',(0.173246785557543,-0.0903698583266489,
-0.292373451287448));
#83392=CARTESIAN_POINT('Ctrl Pts',(0.167594018727271,-0.101206698186584,
-0.293068587723955));
#83393=CARTESIAN_POINT('Ctrl Pts',(0.160915918632716,-0.111520125358314,
-0.293763724160463));
#83394=CARTESIAN_POINT('Ctrl Pts',(0.153336919679044,-0.121115436932467,
-0.29445886059697));
#83395=CARTESIAN_POINT('Ctrl Pts',(0.14575831390225,-0.130710250729187,
-0.295153960971779));
#83396=CARTESIAN_POINT('Ctrl Pts',(0.137279465614492,-0.139586353029643,
-0.295849061346588));
#83397=CARTESIAN_POINT('Ctrl Pts',(0.128064964606821,-0.147582264653493,
-0.296544161721397));
#83398=CARTESIAN_POINT('Ctrl Pts',(0.118829412340891,-0.15559644357152,
-0.297240850108134));
#83399=CARTESIAN_POINT('Ctrl Pts',(0.108855555357494,-0.162725893770916,
-0.297937538494871));
#83400=CARTESIAN_POINT('Ctrl Pts',(0.0983398621120382,-0.168850322829971,
-0.298634226881607));
#83401=CARTESIAN_POINT('Ctrl Pts',(0.09507961791375,-0.170749116741274,
-0.298850225410459));
#83402=CARTESIAN_POINT('Ctrl Pts',(0.0917674698458486,-0.172551639662424,
-0.299066223939311));
#83403=CARTESIAN_POINT('Ctrl Pts',(0.0884096957325332,-0.174255231486693,
-0.299282222468162));
#83404=CARTESIAN_POINT('Ctrl Pts',(0.0775794623433502,-0.179750031444668,
-0.299978908546569));
#83405=CARTESIAN_POINT('Ctrl Pts',(0.066196996889879,-0.184250582423813,
-0.300675594624976));
#83406=CARTESIAN_POINT('Ctrl Pts',(0.0544679948553741,-0.187654996033772,
-0.301372280703383));
#83407=CARTESIAN_POINT('Ctrl Pts',(0.0427634653374316,-0.191052306348138,
-0.302067513149031));
#83408=CARTESIAN_POINT('Ctrl Pts',(0.0307146457960079,-0.193357706528318,
-0.302762745594679));
#83409=CARTESIAN_POINT('Ctrl Pts',(0.0185455848429963,-0.194517920210019,
-0.303457978040326));
#83410=CARTESIAN_POINT('Ctrl Pts',(0.00637820440977671,-0.195677973668835,
-0.304153114475946));
#83411=CARTESIAN_POINT('Ctrl Pts',(-0.00590851907373053,-0.195693026527156,
-0.304848250911565));
#83412=CARTESIAN_POINT('Ctrl Pts',(-0.0180835219950757,-0.194561420205172,
-0.305543387347185));
#83413=CARTESIAN_POINT('Ctrl Pts',(-0.0302578933118102,-0.193429872587714,
-0.306238487721098));
#83414=CARTESIAN_POINT('Ctrl Pts',(-0.0423196868550718,-0.191151891791996,
-0.306933588095011));
#83415=CARTESIAN_POINT('Ctrl Pts',(-0.0540438381313047,-0.187777590675877,
-0.307628688468925));
#83416=CARTESIAN_POINT('Ctrl Pts',(-0.0657947741609637,-0.184395580701245,
-0.30832537685477));
#83417=CARTESIAN_POINT('Ctrl Pts',(-0.0772057058796961,-0.179912554912077,
-0.309022065240616));
#83418=CARTESIAN_POINT('Ctrl Pts',(-0.0880687538179938,-0.174427791939661,
-0.309718753626461));
#83419=CARTESIAN_POINT('Ctrl Pts',(-0.0914366905729014,-0.17272731755055,
-0.309934752159721));
#83420=CARTESIAN_POINT('Ctrl Pts',(-0.0947521462737708,-0.170930885591786,
-0.310150750692981));
#83421=CARTESIAN_POINT('Ctrl Pts',(-0.0980094712277496,-0.169042312897265,
-0.310366749226242));
#83422=CARTESIAN_POINT('Ctrl Pts',(-0.108515713628368,-0.162950871975601,
-0.311063435304748));
#83423=CARTESIAN_POINT('Ctrl Pts',(-0.118488768195282,-0.155854840580449,
-0.311760121383255));
#83424=CARTESIAN_POINT('Ctrl Pts',(-0.127731166881062,-0.147871258218771,
-0.312456807461761));
#83425=CARTESIAN_POINT('Ctrl Pts',(-0.136954281338361,-0.139904333570267,
-0.313152039907507));
#83426=CARTESIAN_POINT('Ctrl Pts',(-0.145449062057614,-0.131054044145402,
-0.313847272353253));
#83427=CARTESIAN_POINT('Ctrl Pts',(-0.153048819121446,-0.12147929439016,
-0.314542504798999));
#83428=CARTESIAN_POINT('Ctrl Pts',(-0.160647526675976,-0.111905866886252,
-0.315237641234713));
#83429=CARTESIAN_POINT('Ctrl Pts',(-0.167350877291185,-0.101608833764162,
-0.315932777670427));
#83430=CARTESIAN_POINT('Ctrl Pts',(-0.173031654364707,-0.0907810915764546,
-0.316627914106141));
#83431=CARTESIAN_POINT('Ctrl Pts',(-0.178712136735613,-0.0799539111013252,
-0.317323014480146));
#83432=CARTESIAN_POINT('Ctrl Pts',(-0.183369768325558,-0.0685968635977168,
-0.318018114854152));
#83433=CARTESIAN_POINT('Ctrl Pts',(-0.186924021548781,-0.056926006078336,
-0.318713215228158));
#83434=CARTESIAN_POINT('Ctrl Pts',(-0.190486394745354,-0.0452284855594271,
-0.319409903614091));
#83435=CARTESIAN_POINT('Ctrl Pts',(-0.192940165079464,-0.0332165792117047,
-0.320106592000024));
#83436=CARTESIAN_POINT('Ctrl Pts',(-0.194255399811661,-0.0211187036536718,
-0.320803280385958));
#83437=CARTESIAN_POINT('Ctrl Pts',(-0.194663170025953,-0.0173679257978144,
-0.321019278918746));
#83438=CARTESIAN_POINT('Ctrl Pts',(-0.194961879337744,-0.0136089117019791,
-0.321235277451534));
#83439=CARTESIAN_POINT('Ctrl Pts',(-0.19515165250027,-0.0098484783806397,
-0.321451275984323));
#83440=CARTESIAN_POINT('Ctrl Pts',(-0.195316169027614,-0.00658851568041518,
-0.321638527585407));
#83441=CARTESIAN_POINT('Ctrl Pts',(-0.19539900625428,-0.00332439645530177,
-0.321825779186492));
#83442=CARTESIAN_POINT('Ctrl Pts',(-0.195399991113052,-5.89323256041572E-5,
-0.322013030787577));
#83443=CARTESIAN_POINT('',(-0.195399958457515,-0.000127415860640841,-0.392013030782495));
#83444=CARTESIAN_POINT('Ctrl Pts',(-0.195399991113071,-5.89322641801936E-5,
-0.322013030791099));
#83445=CARTESIAN_POINT('Ctrl Pts',(-0.195403626754625,0.0119956584972156,
-0.322704277526881));
#83446=CARTESIAN_POINT('Ctrl Pts',(-0.194287443259356,0.0240951078562085,
-0.323395524262662));
#83447=CARTESIAN_POINT('Ctrl Pts',(-0.192052701434784,0.0360127737282426,
-0.324086770998444));
#83448=CARTESIAN_POINT('Ctrl Pts',(-0.189776451431471,0.0481517987746372,
-0.324790856977107));
#83449=CARTESIAN_POINT('Ctrl Pts',(-0.186339582668901,0.0601012590536241,
-0.32549494295577));
#83450=CARTESIAN_POINT('Ctrl Pts',(-0.181798927369129,0.0716261824156088,
-0.326199028934434));
#83451=CARTESIAN_POINT('Ctrl Pts',(-0.177350367924567,0.0829173514837377,
-0.326888834287049));
#83452=CARTESIAN_POINT('Ctrl Pts',(-0.171842810096671,0.0938002223460869,
-0.327578639639665));
#83453=CARTESIAN_POINT('Ctrl Pts',(-0.165379301193847,0.104071354063618,
-0.328268444992281));
#83454=CARTESIAN_POINT('Ctrl Pts',(-0.158715077074959,0.114661441390694,
-0.328979671283968));
#83455=CARTESIAN_POINT('Ctrl Pts',(-0.151034936542069,0.124600231003395,
-0.329690897575655));
#83456=CARTESIAN_POINT('Ctrl Pts',(-0.14249967734951,0.133697426883562,
-0.330402123867342));
#83457=CARTESIAN_POINT('Ctrl Pts',(-0.133964418156952,0.142794622763729,
-0.331113350159029));
#83458=CARTESIAN_POINT('Ctrl Pts',(-0.124574843318938,0.151049580247938,
-0.331824576450716));
#83459=CARTESIAN_POINT('Ctrl Pts',(-0.114529878220969,0.15831635100232,
-0.332535802742403));
#83460=CARTESIAN_POINT('Ctrl Pts',(-0.104690271017,0.165434560888274,-0.333232488820959));
#83461=CARTESIAN_POINT('Ctrl Pts',(-0.0941499836913328,0.171656925557161,
-0.333929174899515));
#83462=CARTESIAN_POINT('Ctrl Pts',(-0.0830962830901262,0.176850693344995,
-0.334625860978071));
#83463=CARTESIAN_POINT('Ctrl Pts',(-0.0720656459916771,0.182033624356801,
-0.335321093423868));
#83464=CARTESIAN_POINT('Ctrl Pts',(-0.0605244745726656,0.186191783164639,
-0.336016325869666));
#83465=CARTESIAN_POINT('Ctrl Pts',(-0.048685752938174,0.189237568840976,
-0.336711558315464));
#83466=CARTESIAN_POINT('Ctrl Pts',(-0.0368486662043658,0.192282933901199,
-0.337406694751233));
#83467=CARTESIAN_POINT('Ctrl Pts',(-0.0247149456230209,0.194215969199016,
-0.338101831187002));
#83468=CARTESIAN_POINT('Ctrl Pts',(-0.0125125627019548,0.194998963521937,
-0.338796967622772));
#83469=CARTESIAN_POINT('Ctrl Pts',(-0.000310812805895387,0.195781917225334,
-0.339492067996835));
#83470=CARTESIAN_POINT('Ctrl Pts',(0.0119587174464459,0.195414919359468,
-0.340187168370898));
#83471=CARTESIAN_POINT('Ctrl Pts',(0.0240658997042646,0.193912331921991,
-0.340882268744961));
#83472=CARTESIAN_POINT('Ctrl Pts',(0.0362007417801083,0.19240631170435,
-0.341578957130953));
#83473=CARTESIAN_POINT('Ctrl Pts',(0.0481716358262746,0.189759695239158,
-0.342275645516946));
#83474=CARTESIAN_POINT('Ctrl Pts',(0.0597577521874501,0.186038090329651,
-0.342972333902938));
#83475=CARTESIAN_POINT('Ctrl Pts',(0.0633498662256263,0.18488425855175,
-0.343188332435453));
#83476=CARTESIAN_POINT('Ctrl Pts',(0.0669051233157821,0.183627452595414,
-0.343404330967968));
#83477=CARTESIAN_POINT('Ctrl Pts',(0.0704173471656434,0.182270560481262,
-0.343620329500482));
#83478=CARTESIAN_POINT('Ctrl Pts',(0.0817457457087745,0.177894012941515,
-0.344317015579063));
#83479=CARTESIAN_POINT('Ctrl Pts',(0.0927043277675154,0.172441952940687,
-0.345013701657644));
#83480=CARTESIAN_POINT('Ctrl Pts',(0.10307977467419,0.165999156784359,-0.345710387736224));
#83481=CARTESIAN_POINT('Ctrl Pts',(0.113433573251774,0.159569803496826,
-0.346405620182047));
#83482=CARTESIAN_POINT('Ctrl Pts',(0.12320587681191,0.152154211441365,-0.34710085262787));
#83483=CARTESIAN_POINT('Ctrl Pts',(0.132207231602128,0.143883313529059,
-0.347796085073693));
#83484=CARTESIAN_POINT('Ctrl Pts',(0.141207343325602,0.135613557809052,
-0.348491221509487));
#83485=CARTESIAN_POINT('Ctrl Pts',(0.149436043646649,0.126489288433088,
-0.349186357945281));
#83486=CARTESIAN_POINT('Ctrl Pts',(0.156737561380853,0.116681176084163,
-0.349881494381075));
#83487=CARTESIAN_POINT('Ctrl Pts',(0.164038700333029,0.106873572552284,
-0.350576594755162));
#83488=CARTESIAN_POINT('Ctrl Pts',(0.170412251402083,0.0963829144782153,
-0.35127169512925));
#83489=CARTESIAN_POINT('Ctrl Pts',(0.175744944203048,0.0854100379760329,
-0.351966795503338));
#83490=CARTESIAN_POINT('Ctrl Pts',(0.181089819963621,0.0744120930672893,
-0.352663483889354));
#83491=CARTESIAN_POINT('Ctrl Pts',(0.185388766914424,0.0629305453448282,
-0.353360172275371));
#83492=CARTESIAN_POINT('Ctrl Pts',(0.188576559606052,0.0511863377000667,
-0.354056860661387));
#83493=CARTESIAN_POINT('Ctrl Pts',(0.189564890338673,0.0475452096630725,
-0.354272859193779));
#83494=CARTESIAN_POINT('Ctrl Pts',(0.190446783230149,0.0438789201081062,
-0.35448885772617));
#83495=CARTESIAN_POINT('Ctrl Pts',(0.191221297251884,0.0401942219393102,
-0.354704856258562));
#83496=CARTESIAN_POINT('Ctrl Pts',(0.193719430598673,0.0283095211979321,
-0.355401542337165));
#83497=CARTESIAN_POINT('Ctrl Pts',(0.195114117287976,0.0161493267899574,
-0.356098228415768));
#83498=CARTESIAN_POINT('Ctrl Pts',(0.195360299149651,0.00393872011683205,
-0.35679491449437));
#83499=CARTESIAN_POINT('Ctrl Pts',(0.195605967353843,-0.00824640917358917,
-0.357490146940215));
#83500=CARTESIAN_POINT('Ctrl Pts',(0.194707795953346,-0.0204808773087043,
-0.35818537938606));
#83501=CARTESIAN_POINT('Ctrl Pts',(0.192672435277541,-0.0325344845390488,
-0.358880611831906));
#83502=CARTESIAN_POINT('Ctrl Pts',(0.190637355680441,-0.0445864271935094,
-0.359575748267723));
#83503=CARTESIAN_POINT('Ctrl Pts',(0.187465499323653,-0.0564566895275863,
-0.360270884703541));
#83504=CARTESIAN_POINT('Ctrl Pts',(0.183215187569739,-0.0679216831636653,
-0.360966021139358));
#83505=CARTESIAN_POINT('Ctrl Pts',(0.17896509630994,-0.0793860820284035,
-0.36166112151347));
#83506=CARTESIAN_POINT('Ctrl Pts',(0.17363699022893,-0.0904444429220991,
-0.362356221887581));
#83507=CARTESIAN_POINT('Ctrl Pts',(0.167337635084274,-0.10089239755503,
-0.363051322261693));
#83508=CARTESIAN_POINT('Ctrl Pts',(0.161023888563226,-0.111364221368887,
-0.363748010647733));
#83509=CARTESIAN_POINT('Ctrl Pts',(0.153734970694931,-0.121222139978164,
-0.364444699033774));
#83510=CARTESIAN_POINT('Ctrl Pts',(0.145620674203163,-0.130291132640009,
-0.365141387419814));
#83511=CARTESIAN_POINT('Ctrl Pts',(0.143104949572476,-0.133102847523494,
-0.36535738595209));
#83512=CARTESIAN_POINT('Ctrl Pts',(0.140510160609027,-0.135838991597314,
-0.365573384484366));
#83513=CARTESIAN_POINT('Ctrl Pts',(0.137841458732347,-0.138495098305097,
-0.365789383016642));
#83514=CARTESIAN_POINT('Ctrl Pts',(0.129233773181065,-0.147062159141318,
-0.366486069095226));
#83515=CARTESIAN_POINT('Ctrl Pts',(0.119794142142335,-0.154853747223658,
-0.367182755173809));
#83516=CARTESIAN_POINT('Ctrl Pts',(0.109686811503521,-0.161709503067046,
-0.367879441252392));
#83517=CARTESIAN_POINT('Ctrl Pts',(0.0996005697702513,-0.168550954402887,
-0.368574673698218));
#83518=CARTESIAN_POINT('Ctrl Pts',(0.088850069189045,-0.174459901826862,
-0.369269906144044));
#83519=CARTESIAN_POINT('Ctrl Pts',(0.0776320063753439,-0.17931656807484,
-0.36996513858987));
#83520=CARTESIAN_POINT('Ctrl Pts',(0.0664154927507509,-0.18417256362819,
-0.370660275025667));
#83521=CARTESIAN_POINT('Ctrl Pts',(0.054732328796273,-0.187976177782212,
-0.371355411461464));
#83522=CARTESIAN_POINT('Ctrl Pts',(0.0428018033980549,-0.190654571479087,
-0.372050547897261));
#83523=CARTESIAN_POINT('Ctrl Pts',(0.0308718969216478,-0.193332826228496,
-0.372745648271352));
#83524=CARTESIAN_POINT('Ctrl Pts',(0.0186955141282983,-0.194885811137499,
-0.373440748645443));
#83525=CARTESIAN_POINT('Ctrl Pts',(0.00650220381703275,-0.195291785146026,
-0.374135849019534));
#83526=CARTESIAN_POINT('Ctrl Pts',(-0.00571896307862414,-0.195698686634372,
-0.374832537405554));
#83527=CARTESIAN_POINT('Ctrl Pts',(-0.0179562587032461,-0.19495338214258,
-0.375529225791574));
#83528=CARTESIAN_POINT('Ctrl Pts',(-0.0299813185939873,-0.193086199753804,
-0.376225914177595));
#83529=CARTESIAN_POINT('Ctrl Pts',(-0.0337095209585613,-0.192507305855547,
-0.376441912709971));
#83530=CARTESIAN_POINT('Ctrl Pts',(-0.0374173943191617,-0.191820946392533,
-0.376657911242346));
#83531=CARTESIAN_POINT('Ctrl Pts',(-0.0410983872444957,-0.19102900974957,
-0.376873909774722));
#83532=CARTESIAN_POINT('Ctrl Pts',(-0.0529711370185562,-0.188474681124243,
-0.377570595853311));
#83533=CARTESIAN_POINT('Ctrl Pts',(-0.0646465106214749,-0.184800292708903,
-0.378267281931899));
#83534=CARTESIAN_POINT('Ctrl Pts',(-0.0759005699525302,-0.180056278648874,
-0.378963968010487));
#83535=CARTESIAN_POINT('Ctrl Pts',(-0.0871311477331368,-0.175322162955489,
-0.379659200456318));
#83536=CARTESIAN_POINT('Ctrl Pts',(-0.0979413291472134,-0.169523119913525,
-0.380354432902149));
#83537=CARTESIAN_POINT('Ctrl Pts',(-0.108123542558037,-0.162758900047587,
-0.38104966534798));
#83538=CARTESIAN_POINT('Ctrl Pts',(-0.118304349828217,-0.155995614305113,
-0.381744801783782));
#83539=CARTESIAN_POINT('Ctrl Pts',(-0.127856608459109,-0.148267862001208,
-0.382439938219584));
#83540=CARTESIAN_POINT('Ctrl Pts',(-0.136599812641646,-0.13971990261329,
-0.383135074655386));
#83541=CARTESIAN_POINT('Ctrl Pts',(-0.145342563251557,-0.131172386669253,
-0.383830175029483));
#83542=CARTESIAN_POINT('Ctrl Pts',(-0.153275735998863,-0.121805379131019,
-0.384525275403579));
#83543=CARTESIAN_POINT('Ctrl Pts',(-0.160256095414963,-0.111799570134908,
-0.385220375777675));
#83544=CARTESIAN_POINT('Ctrl Pts',(-0.16725240201572,-0.101770902074644,
-0.3859170641637));
#83545=CARTESIAN_POINT('Ctrl Pts',(-0.173291103041914,-0.0911012735474523,
-0.386613752549726));
#83546=CARTESIAN_POINT('Ctrl Pts',(-0.178273279849769,-0.0799987355625439,
-0.387310440935751));
#83547=CARTESIAN_POINT('Ctrl Pts',(-0.179817934389725,-0.0765565482687536,
-0.387526439468101));
#83548=CARTESIAN_POINT('Ctrl Pts',(-0.181261384311482,-0.0730728912117539,
-0.387742438000452));
#83549=CARTESIAN_POINT('Ctrl Pts',(-0.182601645881345,-0.0695542875847618,
-0.387958436532803));
#83550=CARTESIAN_POINT('Ctrl Pts',(-0.187506976567928,-0.056676268298449,
-0.388748986864783));
#83551=CARTESIAN_POINT('Ctrl Pts',(-0.191054998852211,-0.0432541867438378,
-0.389539537196764));
#83552=CARTESIAN_POINT('Ctrl Pts',(-0.193150344420641,-0.0295652574855622,
-0.390330087528744));
#83553=CARTESIAN_POINT('Ctrl Pts',(-0.194637219047094,-0.0198514795369075,
-0.390891068613328));
#83554=CARTESIAN_POINT('Ctrl Pts',(-0.195393518260447,-0.010003849086555,
-0.391452049697911));
#83555=CARTESIAN_POINT('Ctrl Pts',(-0.195399958457515,-0.000127415860641863,
-0.392013030782495));
#83556=CARTESIAN_POINT('',(-0.195399937376808,0.000156438931572747,-0.462013030791968));
#83557=CARTESIAN_POINT('Ctrl Pts',(-0.195399958457573,-0.000127415771186929,
-0.392013030787576));
#83558=CARTESIAN_POINT('Ctrl Pts',(-0.195407982922204,0.0121785965931462,
-0.392712011887839));
#83559=CARTESIAN_POINT('Ctrl Pts',(-0.194249139815125,0.0244910033759845,
-0.393410992988102));
#83560=CARTESIAN_POINT('Ctrl Pts',(-0.191946026930775,0.0365770795101272,
-0.394109974088365));
#83561=CARTESIAN_POINT('Ctrl Pts',(-0.189642503287119,0.0486653111913485,
-0.394809079851642));
#83562=CARTESIAN_POINT('Ctrl Pts',(-0.1861945007376,0.0605262928072483,
-0.395508185614918));
#83563=CARTESIAN_POINT('Ctrl Pts',(-0.181675493516228,0.0719386895601725,
-0.396207291378194));
#83564=CARTESIAN_POINT('Ctrl Pts',(-0.177144780405295,0.0833806486150532,
-0.396908208082337));
#83565=CARTESIAN_POINT('Ctrl Pts',(-0.171537904050401,0.0943709278614005,
-0.397609124786481));
#83566=CARTESIAN_POINT('Ctrl Pts',(-0.164975564812825,0.104710185821101,
-0.398310041490624));
#83567=CARTESIAN_POINT('Ctrl Pts',(-0.162688235729128,0.108313974741315,
-0.398554348757377));
#83568=CARTESIAN_POINT('Ctrl Pts',(-0.160285211847533,0.111838934565166,
-0.39879865602413));
#83569=CARTESIAN_POINT('Ctrl Pts',(-0.157772770271872,0.115277547513551,
-0.399042963290883));
#83570=CARTESIAN_POINT('Ctrl Pts',(-0.150608091577316,0.125083370331001,
-0.39973964936947));
#83571=CARTESIAN_POINT('Ctrl Pts',(-0.142500603725442,0.134253109679862,
-0.400436335448058));
#83572=CARTESIAN_POINT('Ctrl Pts',(-0.133587503863308,0.142602730729712,
-0.401133021526646));
#83573=CARTESIAN_POINT('Ctrl Pts',(-0.12469300114891,0.150934930328147,
-0.401828253972477));
#83574=CARTESIAN_POINT('Ctrl Pts',(-0.114996804596432,0.158449761984512,
-0.402523486418308));
#83575=CARTESIAN_POINT('Ctrl Pts',(-0.10467449976499,0.164998209381039,
-0.403218718864138));
#83576=CARTESIAN_POINT('Ctrl Pts',(-0.0943536204205046,0.171545752451788,
-0.40391385529994));
#83577=CARTESIAN_POINT('Ctrl Pts',(-0.0834075178718574,0.177126669904706,
-0.404608991735742));
#83578=CARTESIAN_POINT('Ctrl Pts',(-0.0720414207893906,0.181634781059812,
-0.405304128171544));
#83579=CARTESIAN_POINT('Ctrl Pts',(-0.0606759133477934,0.186142658346902,
-0.40599922854564));
#83580=CARTESIAN_POINT('Ctrl Pts',(-0.0488912779366786,0.189577542375047,
-0.406694328919736));
#83581=CARTESIAN_POINT('Ctrl Pts',(-0.0369108546065943,0.191882122179767,
-0.407389429293832));
#83582=CARTESIAN_POINT('Ctrl Pts',(-0.0249030610493165,0.194191966979812,
-0.408086117679857));
#83583=CARTESIAN_POINT('Ctrl Pts',(-0.0126994575272143,0.195366251471346,
-0.408782806065882));
#83584=CARTESIAN_POINT('Ctrl Pts',(-0.000530343157295054,0.195399280285613,
-0.409479494451907));
#83585=CARTESIAN_POINT('Ctrl Pts',(0.00324252129208505,0.195409520409534,
-0.409695492984259));
#83586=CARTESIAN_POINT('Ctrl Pts',(0.00701208320713229,0.195310438946965,
-0.409911491516611));
#83587=CARTESIAN_POINT('Ctrl Pts',(0.0107715766774621,0.19510287833828,
-0.410127490048963));
#83588=CARTESIAN_POINT('Ctrl Pts',(0.022897523714242,0.194433408111054,
-0.410824176127552));
#83589=CARTESIAN_POINT('Ctrl Pts',(0.0350033751244801,0.192626797852022,
-0.411520862206141));
#83590=CARTESIAN_POINT('Ctrl Pts',(0.046860064980641,0.189697902755961,
-0.41221754828473));
#83591=CARTESIAN_POINT('Ctrl Pts',(0.0586920159001438,0.186775118787975,
-0.412912780730562));
#83592=CARTESIAN_POINT('Ctrl Pts',(0.0702749784319402,0.182734833971876,
-0.413608013176394));
#83593=CARTESIAN_POINT('Ctrl Pts',(0.0813883533085182,0.177643170276056,
-0.414303245622225));
#83594=CARTESIAN_POINT('Ctrl Pts',(0.0925001934531584,0.172552209727478,
-0.414998382058028));
#83595=CARTESIAN_POINT('Ctrl Pts',(0.103141761541885,0.166410481205699,
-0.415693518493831));
#83596=CARTESIAN_POINT('Ctrl Pts',(0.113112243662521,0.159332295325306,
-0.416388654929634));
#83597=CARTESIAN_POINT('Ctrl Pts',(0.123082208542832,0.152254476641114,
-0.417083755303731));
#83598=CARTESIAN_POINT('Ctrl Pts',(0.132380458758455,0.144240825601304,
-0.417778855677828));
#83599=CARTESIAN_POINT('Ctrl Pts',(0.140837306302754,0.135447455322661,
-0.418473956051925));
#83600=CARTESIAN_POINT('Ctrl Pts',(0.149313474185928,0.126633995892269,
-0.419170644437951));
#83601=CARTESIAN_POINT('Ctrl Pts',(0.156943842972338,0.11703793653566,-0.419867332823977));
#83602=CARTESIAN_POINT('Ctrl Pts',(0.163598226593451,0.106849334370776,
-0.420564021210002));
#83603=CARTESIAN_POINT('Ctrl Pts',(0.165661325569498,0.103690500151024,
-0.420780019742349));
#83604=CARTESIAN_POINT('Ctrl Pts',(0.16763093497854,0.10047490488067,-0.420996018274696));
#83605=CARTESIAN_POINT('Ctrl Pts',(0.169504077028634,0.0972086820745506,
-0.421212016807043));
#83606=CARTESIAN_POINT('Ctrl Pts',(0.175545747661026,0.086673740314212,
-0.421908702885632));
#83607=CARTESIAN_POINT('Ctrl Pts',(0.180622723021697,0.0755364246510001,
-0.422605388964221));
#83608=CARTESIAN_POINT('Ctrl Pts',(0.184622724926109,0.0639969486839681,
-0.42330207504281));
#83609=CARTESIAN_POINT('Ctrl Pts',(0.188614380842308,0.0524815497880715,
-0.423997307488642));
#83610=CARTESIAN_POINT('Ctrl Pts',(0.191533170069643,0.0405664504660143,
-0.424692539934473));
#83611=CARTESIAN_POINT('Ctrl Pts',(0.193314423861388,0.028472680364513,
-0.425387772380304));
#83612=CARTESIAN_POINT('Ctrl Pts',(0.195095431666012,0.016380580385307,
-0.426082908816108));
#83613=CARTESIAN_POINT('Ctrl Pts',(0.195739043730156,0.00411071632195411,
-0.426778045251911));
#83614=CARTESIAN_POINT('Ctrl Pts',(0.195231782616843,-0.00810623563990015,
-0.427473181687714));
#83615=CARTESIAN_POINT('Ctrl Pts',(0.194724547818799,-0.0203225538209459,
-0.428168282061811));
#83616=CARTESIAN_POINT('Ctrl Pts',(0.193066621695153,-0.0324850922496084,
-0.428863382435908));
#83617=CARTESIAN_POINT('Ctrl Pts',(0.190296537362577,-0.0443665174181312,
-0.429558482810005));
#83618=CARTESIAN_POINT('Ctrl Pts',(0.187520124552663,-0.0562750866447022,
-0.430255171196031));
#83619=CARTESIAN_POINT('Ctrl Pts',(0.18362674334812,-0.0679004238780226,
-0.430951859582057));
#83620=CARTESIAN_POINT('Ctrl Pts',(0.178704907429044,-0.0790298428492471,
-0.431648547968084));
#83621=CARTESIAN_POINT('Ctrl Pts',(0.177178960741411,-0.082480364218438,
-0.43186454650043));
#83622=CARTESIAN_POINT('Ctrl Pts',(0.175554497251728,-0.0858833823696525,
-0.432080545032776));
#83623=CARTESIAN_POINT('Ctrl Pts',(0.173835039761986,-0.089233059742164,
-0.432296543565122));
#83624=CARTESIAN_POINT('Ctrl Pts',(0.168289066449964,-0.10003717756576,
-0.432993229643711));
#83625=CARTESIAN_POINT('Ctrl Pts',(0.161712540702625,-0.11036019980197,
-0.4336899157223));
#83626=CARTESIAN_POINT('Ctrl Pts',(0.15421224645812,-0.119998929338307,
-0.434386601800889));
#83627=CARTESIAN_POINT('Ctrl Pts',(0.146727601547996,-0.129617547703455,
-0.43508183424672));
#83628=CARTESIAN_POINT('Ctrl Pts',(0.138323487648071,-0.138553978308862,
-0.435777066692552));
#83629=CARTESIAN_POINT('Ctrl Pts',(0.129150073398274,-0.14663362009178,
-0.436472299138383));
#83630=CARTESIAN_POINT('Ctrl Pts',(0.119977925976243,-0.154712146094437,
-0.437167435574186));
#83631=CARTESIAN_POINT('Ctrl Pts',(0.110037314746755,-0.161933506700741,
-0.437862572009989));
#83632=CARTESIAN_POINT('Ctrl Pts',(0.0995143753671538,-0.168160783464175,
-0.438557708445792));
#83633=CARTESIAN_POINT('Ctrl Pts',(0.0889919818877899,-0.174387737174161,
-0.439252808819889));
#83634=CARTESIAN_POINT('Ctrl Pts',(0.07788808700947,-0.179620287087094,
-0.439947909193986));
#83635=CARTESIAN_POINT('Ctrl Pts',(0.0664143450939421,-0.183766957763747,
-0.440643009568083));
#83636=CARTESIAN_POINT('Ctrl Pts',(0.0549143905050947,-0.187923101838409,
-0.441339697954108));
#83637=CARTESIAN_POINT('Ctrl Pts',(0.0430437465390059,-0.190988178480599,
-0.442036386340134));
#83638=CARTESIAN_POINT('Ctrl Pts',(0.0310289993702008,-0.192920608536476,
-0.44273307472616));
#83639=CARTESIAN_POINT('Ctrl Pts',(0.027303994321965,-0.193519731565231,
-0.442949073258508));
#83640=CARTESIAN_POINT('Ctrl Pts',(0.0235651843507864,-0.194010357865431,
-0.443165071790856));
#83641=CARTESIAN_POINT('Ctrl Pts',(0.0198193839265638,-0.194392263273957,
-0.443381070323204));
#83642=CARTESIAN_POINT('Ctrl Pts',(0.00773760272017369,-0.195624068780068,
-0.444077756401793));
#83643=CARTESIAN_POINT('Ctrl Pts',(-0.00450185620683019,-0.195729539956344,
-0.444774442480382));
#83644=CARTESIAN_POINT('Ctrl Pts',(-0.0166704164553885,-0.194687588754918,
-0.445471128558971));
#83645=CARTESIAN_POINT('Ctrl Pts',(-0.0288135870509505,-0.193647811580566,
-0.446166361004803));
#83646=CARTESIAN_POINT('Ctrl Pts',(-0.0408852831489385,-0.191465364393067,
-0.446861593450635));
#83647=CARTESIAN_POINT('Ctrl Pts',(-0.0526572875794893,-0.188171119103785,
-0.447556825896467));
#83648=CARTESIAN_POINT('Ctrl Pts',(-0.0644276663228442,-0.18487732874233,
-0.44825196233227));
#83649=CARTESIAN_POINT('Ctrl Pts',(-0.0758975820168812,-0.180472236848403,
-0.448947098768073));
#83650=CARTESIAN_POINT('Ctrl Pts',(-0.0868508371809369,-0.175037401948756,
-0.449642235203876));
#83651=CARTESIAN_POINT('Ctrl Pts',(-0.0978035241211859,-0.169602848992926,
-0.450337335577973));
#83652=CARTESIAN_POINT('Ctrl Pts',(-0.108238831969957,-0.163139072220679,
-0.45103243595207));
#83653=CARTESIAN_POINT('Ctrl Pts',(-0.117964781420494,-0.155773779386696,
-0.451727536326167));
#83654=CARTESIAN_POINT('Ctrl Pts',(-0.127712950573862,-0.148391659957133,
-0.452424224712193));
#83655=CARTESIAN_POINT('Ctrl Pts',(-0.136747868534464,-0.140104492742853,
-0.453120913098219));
#83656=CARTESIAN_POINT('Ctrl Pts',(-0.144911274345799,-0.13107968022343,
-0.453817601484244));
#83657=CARTESIAN_POINT('Ctrl Pts',(-0.147442224638013,-0.1282816627769,
-0.454033600016591));
#83658=CARTESIAN_POINT('Ctrl Pts',(-0.149889693047452,-0.125412984936567,
-0.454249598548937));
#83659=CARTESIAN_POINT('Ctrl Pts',(-0.152249780747947,-0.122479240127468,
-0.454465597081283));
#83660=CARTESIAN_POINT('Ctrl Pts',(-0.159839932411845,-0.113044180557622,
-0.455160258393802));
#83661=CARTESIAN_POINT('Ctrl Pts',(-0.166577789997525,-0.102865895547722,
-0.455854919706322));
#83662=CARTESIAN_POINT('Ctrl Pts',(-0.172320935541128,-0.092123043665689,
-0.456549581018841));
#83663=CARTESIAN_POINT('Ctrl Pts',(-0.178051864918719,-0.0814030427563561,
-0.457242764726823));
#83664=CARTESIAN_POINT('Ctrl Pts',(-0.182791800687757,-0.0701215888384119,
-0.457935948434805));
#83665=CARTESIAN_POINT('Ctrl Pts',(-0.186441932507934,-0.0584856033798669,
-0.458629132142786));
#83666=CARTESIAN_POINT('Ctrl Pts',(-0.190090870931465,-0.0468534222622858,
-0.459322089217005));
#83667=CARTESIAN_POINT('Ctrl Pts',(-0.192650406516594,-0.034867764431544,
-0.460015046291223));
#83668=CARTESIAN_POINT('Ctrl Pts',(-0.194070739924089,-0.0227531954968199,
-0.460708003365442));
#83669=CARTESIAN_POINT('Ctrl Pts',(-0.194962365160494,-0.0151481815378657,
-0.461143012506153));
#83670=CARTESIAN_POINT('Ctrl Pts',(-0.195406061327982,-0.00749268174718338,
-0.461578021646865));
#83671=CARTESIAN_POINT('Ctrl Pts',(-0.19539993737687,0.00015643885435388,
-0.462013030787577));
#83672=CARTESIAN_POINT('',(-0.195399999942242,4.75099905391278E-6,-0.532013030784479));
#83673=CARTESIAN_POINT('Ctrl Pts',(-0.195399937376808,0.000156438931571927,
-0.462013030791968));
#83674=CARTESIAN_POINT('Ctrl Pts',(-0.195388329591929,0.0146551344658182,
-0.462837578529473));
#83675=CARTESIAN_POINT('Ctrl Pts',(-0.193758956620724,0.0290846302221516,
-0.463662126266977));
#83676=CARTESIAN_POINT('Ctrl Pts',(-0.190581249380799,0.0431271073045003,
-0.464486674004482));
#83677=CARTESIAN_POINT('Ctrl Pts',(-0.189215113705894,0.0491641420146828,
-0.464841157282775));
#83678=CARTESIAN_POINT('Ctrl Pts',(-0.187563420811457,0.0551299029508943,
-0.465195640561069));
#83679=CARTESIAN_POINT('Ctrl Pts',(-0.185634374162934,0.0610003207297784,
-0.465550123839363));
#83680=CARTESIAN_POINT('Ctrl Pts',(-0.181843109448154,0.0725377855200353,
-0.466246809917952));
#83681=CARTESIAN_POINT('Ctrl Pts',(-0.176958821129432,0.0837609404514446,
-0.466943495996541));
#83682=CARTESIAN_POINT('Ctrl Pts',(-0.171055261286761,0.0944524091070096,
-0.46764018207513));
#83683=CARTESIAN_POINT('Ctrl Pts',(-0.165164019198436,0.105121570055359,
-0.468335414520962));
#83684=CARTESIAN_POINT('Ctrl Pts',(-0.158258080992425,0.115260452632001,
-0.469030646966793));
#83685=CARTESIAN_POINT('Ctrl Pts',(-0.150458515822565,0.124673152749383,
-0.469725879412625));
#83686=CARTESIAN_POINT('Ctrl Pts',(-0.142660027755015,0.134084552994167,
-0.470421015848428));
#83687=CARTESIAN_POINT('Ctrl Pts',(-0.133968680219217,0.14276926822463,
-0.471116152284231));
#83688=CARTESIAN_POINT('Ctrl Pts',(-0.124546951277911,0.150562999861777,
-0.471811288720034));
#83689=CARTESIAN_POINT('Ctrl Pts',(-0.11512571110917,0.158356327182241,
-0.472506389094131));
#83690=CARTESIAN_POINT('Ctrl Pts',(-0.104974856198617,0.165258225808353,
-0.473201489468229));
#83691=CARTESIAN_POINT('Ctrl Pts',(-0.0942891648455739,0.171145299066975,
-0.473896589842326));
#83692=CARTESIAN_POINT('Ctrl Pts',(-0.0835790611832178,0.177045821811324,
-0.474593278228352));
#83693=CARTESIAN_POINT('Ctrl Pts',(-0.0723324791007605,0.181926526110376,
-0.475289966614378));
#83694=CARTESIAN_POINT('Ctrl Pts',(-0.0607667352856288,0.185710968665629,
-0.475986655000404));
#83695=CARTESIAN_POINT('Ctrl Pts',(-0.0571809374746232,0.186884282379595,
-0.47620265353275));
#83696=CARTESIAN_POINT('Ctrl Pts',(-0.0535645658198097,0.187952584874734,
-0.476418652065097));
#83697=CARTESIAN_POINT('Ctrl Pts',(-0.0499243162402038,0.188914590881562,
-0.476634650597444));
#83698=CARTESIAN_POINT('Ctrl Pts',(-0.0381829808841359,0.192017464707577,
-0.477331336676032));
#83699=CARTESIAN_POINT('Ctrl Pts',(-0.0261100611714576,0.194032430862605,
-0.478028022754621));
#83700=CARTESIAN_POINT('Ctrl Pts',(-0.0139280386221067,0.194902975195714,
-0.47872470883321));
#83701=CARTESIAN_POINT('Ctrl Pts',(-0.00177143381479845,0.195771703141503,
-0.479419941279041));
#83702=CARTESIAN_POINT('Ctrl Pts',(0.0104929631452944,0.195500613463922,
-0.480115173724872));
#83703=CARTESIAN_POINT('Ctrl Pts',(0.0226349137272716,0.194084570949262,
-0.480810406170703));
#83704=CARTESIAN_POINT('Ctrl Pts',(0.0347751875333354,0.192668723986869,
-0.481505542606506));
#83705=CARTESIAN_POINT('Ctrl Pts',(0.0467921755147186,0.19010829424219,
-0.482200679042309));
#83706=CARTESIAN_POINT('Ctrl Pts',(0.0584595984062355,0.186450088104516,
-0.482895815478112));
#83707=CARTESIAN_POINT('Ctrl Pts',(0.0701264160249562,0.182792071744197,
-0.483590915852209));
#83708=CARTESIAN_POINT('Ctrl Pts',(0.08144287774861,0.178036679634478,-0.484286016226306));
#83709=CARTESIAN_POINT('Ctrl Pts',(0.092199420855013,0.172280082406528,
-0.484981116600402));
#83710=CARTESIAN_POINT('Ctrl Pts',(0.10298053813718,0.16651033377569,-0.485677804986428));
#83711=CARTESIAN_POINT('Ctrl Pts',(0.113198443100993,0.15973528387605,-0.486374493372454));
#83712=CARTESIAN_POINT('Ctrl Pts',(0.122670680915762,0.152095575358599,
-0.48707118175848));
#83713=CARTESIAN_POINT('Ctrl Pts',(0.125607416344511,0.149726990119582,
-0.487287180290827));
#83714=CARTESIAN_POINT('Ctrl Pts',(0.128472724790555,0.147275577939621,
-0.487503178823175));
#83715=CARTESIAN_POINT('Ctrl Pts',(0.131261882003931,0.144746254987084,
-0.487719177355523));
#83716=CARTESIAN_POINT('Ctrl Pts',(0.140258086656035,0.136588125067709,
-0.488415863434112));
#83717=CARTESIAN_POINT('Ctrl Pts',(0.14852239569127,0.127559466520344,-0.489112549512701));
#83718=CARTESIAN_POINT('Ctrl Pts',(0.155886256925708,0.117816106291509,
-0.48980923559129));
#83719=CARTESIAN_POINT('Ctrl Pts',(0.163234753492699,0.108093075545396,
-0.490504468037121));
#83720=CARTESIAN_POINT('Ctrl Pts',(0.169685950201453,0.0976589496388772,
-0.491199700482953));
#83721=CARTESIAN_POINT('Ctrl Pts',(0.175110163793777,0.08670403990655,-0.491894932928784));
#83722=CARTESIAN_POINT('Ctrl Pts',(0.180533628314472,0.0757506430224801,
-0.492590069364587));
#83723=CARTESIAN_POINT('Ctrl Pts',(0.184929962974441,0.0642773678937392,
-0.49328520580039));
#83724=CARTESIAN_POINT('Ctrl Pts',(0.188215205454289,0.0524994898622816,
-0.493980342236193));
#83725=CARTESIAN_POINT('Ctrl Pts',(0.191500277505078,0.0407222228337199,
-0.49467544261029));
#83726=CARTESIAN_POINT('Ctrl Pts',(0.193674162774775,0.0286412343437673,
-0.495370542984387));
#83727=CARTESIAN_POINT('Ctrl Pts',(0.194703405140545,0.0164846603445962,
-0.496065643358484));
#83728=CARTESIAN_POINT('Ctrl Pts',(0.195734998892123,0.00430031368805828,
-0.49676233174451));
#83729=CARTESIAN_POINT('Ctrl Pts',(0.195616720597611,-0.00795908651086126,
-0.497459020130536));
#83730=CARTESIAN_POINT('Ctrl Pts',(0.194367175683108,-0.0200639232696899,
-0.498155708516562));
#83731=CARTESIAN_POINT('Ctrl Pts',(0.193979771682914,-0.0238168593407548,
-0.498371707048909));
#83732=CARTESIAN_POINT('Ctrl Pts',(0.193484002827447,-0.0275549908805594,
-0.498587705581256));
#83733=CARTESIAN_POINT('Ctrl Pts',(0.19288141986272,-0.0312716784285904,
-0.498803704113604));
#83734=CARTESIAN_POINT('Ctrl Pts',(0.190937836458897,-0.0432595583694434,
-0.499500390192193));
#83735=CARTESIAN_POINT('Ctrl Pts',(0.187865562364591,-0.0551076219616193,
-0.500197076270781));
#83736=CARTESIAN_POINT('Ctrl Pts',(0.183703509188537,-0.0665896441784849,
-0.50089376234937));
#83737=CARTESIAN_POINT('Ctrl Pts',(0.179550140120032,-0.0780477092012426,
-0.501588994795202));
#83738=CARTESIAN_POINT('Ctrl Pts',(0.174311731072823,-0.0891404091909756,
-0.502284227241033));
#83739=CARTESIAN_POINT('Ctrl Pts',(0.16807728275083,-0.0996553411669321,
-0.502979459686865));
#83740=CARTESIAN_POINT('Ctrl Pts',(0.161843695392049,-0.110168821054565,
-0.503674596122668));
#83741=CARTESIAN_POINT('Ctrl Pts',(0.154614748386074,-0.12010391671626,
-0.504369732558471));
#83742=CARTESIAN_POINT('Ctrl Pts',(0.146525277771686,-0.12927297851419,
-0.505064868994274));
#83743=CARTESIAN_POINT('Ctrl Pts',(0.138436226816083,-0.138441564647208,
-0.505759969368371));
#83744=CARTESIAN_POINT('Ctrl Pts',(0.129487340027504,-0.14684355758373,
-0.506455069742468));
#83745=CARTESIAN_POINT('Ctrl Pts',(0.119851743118805,-0.154326665457995,
-0.507150170116565));
#83746=CARTESIAN_POINT('Ctrl Pts',(0.110194132924826,-0.16182686908564,
-0.507846858502591));
#83747=CARTESIAN_POINT('Ctrl Pts',(0.0998474112615499,-0.168403512136232,
-0.508543546888617));
#83748=CARTESIAN_POINT('Ctrl Pts',(0.0890142960991703,-0.173947161776125,
-0.509240235274643));
#83749=CARTESIAN_POINT('Ctrl Pts',(0.0856556395997188,-0.175665893148829,
-0.50945623380699));
#83750=CARTESIAN_POINT('Ctrl Pts',(0.0822503900941689,-0.177285673989513,
-0.509672232339337));
#83751=CARTESIAN_POINT('Ctrl Pts',(0.0788049607474615,-0.178804189440827,
-0.509888230871684));
#83752=CARTESIAN_POINT('Ctrl Pts',(0.0676920025503313,-0.183702040197298,
-0.510584916950272));
#83753=CARTESIAN_POINT('Ctrl Pts',(0.0560816847625869,-0.187577088566324,
-0.511281603028861));
#83754=CARTESIAN_POINT('Ctrl Pts',(0.0441849381383652,-0.190338780183411,
-0.51197828910745));
#83755=CARTESIAN_POINT('Ctrl Pts',(0.0323130140290933,-0.193094709541822,
-0.512673521553281));
#83756=CARTESIAN_POINT('Ctrl Pts',(0.0201566744902528,-0.194741625272648,
-0.513368753999112));
#83757=CARTESIAN_POINT('Ctrl Pts',(0.00794253330288551,-0.19523851096731,
-0.514063986444944));
#83758=CARTESIAN_POINT('Ctrl Pts',(-0.0042699211392091,-0.195735328043182,
-0.514759122880747));
#83759=CARTESIAN_POINT('Ctrl Pts',(-0.0165392903042251,-0.195082349548358,
-0.51545425931655));
#83760=CARTESIAN_POINT('Ctrl Pts',(-0.0286347621607715,-0.193290481907403,
-0.516149395752352));
#83761=CARTESIAN_POINT('Ctrl Pts',(-0.0407296065385554,-0.191498707223457,
-0.516844496126449));
#83762=CARTESIAN_POINT('Ctrl Pts',(-0.0526497099517824,-0.188568315666333,
-0.517539596500546));
#83763=CARTESIAN_POINT('Ctrl Pts',(-0.0641730653434497,-0.184561582363246,
-0.518234696874643));
#83764=CARTESIAN_POINT('Ctrl Pts',(-0.0757227467543576,-0.180545695360178,
-0.518931385260669));
#83765=CARTESIAN_POINT('Ctrl Pts',(-0.0868730663070533,-0.175448906482376,
-0.519628073646694));
#83766=CARTESIAN_POINT('Ctrl Pts',(-0.0974218496138087,-0.169381649589985,
-0.52032476203272));
#83767=CARTESIAN_POINT('Ctrl Pts',(-0.100692352980909,-0.16750058108013,
-0.520540760565068));
#83768=CARTESIAN_POINT('Ctrl Pts',(-0.103905235860399,-0.165526550236975,
-0.520756759097416));
#83769=CARTESIAN_POINT('Ctrl Pts',(-0.10705506443072,-0.163463675413635,
-0.520972757629764));
#83770=CARTESIAN_POINT('Ctrl Pts',(-0.117207367848539,-0.156814764004024,
-0.521668948736437));
#83771=CARTESIAN_POINT('Ctrl Pts',(-0.1267737660995,-0.149192930854621,
-0.522365139843109));
#83772=CARTESIAN_POINT('Ctrl Pts',(-0.135563601880418,-0.140725512417641,
-0.523061330949781));
#83773=CARTESIAN_POINT('Ctrl Pts',(-0.144335100214774,-0.132275758796816,
-0.523756069655347));
#83774=CARTESIAN_POINT('Ctrl Pts',(-0.152332575326338,-0.122984469850852,
-0.524450808360913));
#83775=CARTESIAN_POINT('Ctrl Pts',(-0.159398358528159,-0.113019128020563,
-0.525145547066479));
#83776=CARTESIAN_POINT('Ctrl Pts',(-0.16646317386283,-0.103055151237392,
-0.525840190607114));
#83777=CARTESIAN_POINT('Ctrl Pts',(-0.172596007680861,-0.0924179925879917,
-0.526534834147748));
#83778=CARTESIAN_POINT('Ctrl Pts',(-0.17768045116012,-0.081306932518306,
-0.527229477688383));
#83779=CARTESIAN_POINT('Ctrl Pts',(-0.18276467250458,-0.0701963578809189,
-0.527924090880662));
#83780=CARTESIAN_POINT('Ctrl Pts',(-0.186800254976389,-0.0586127313267355,
-0.52861870407294));
#83781=CARTESIAN_POINT('Ctrl Pts',(-0.189718671700916,-0.0467759084149099,
-0.529313317265219));
#83782=CARTESIAN_POINT('Ctrl Pts',(-0.192643733322442,-0.034912134427736,
-0.530009512011316));
#83783=CARTESIAN_POINT('Ctrl Pts',(-0.194446406647556,-0.0227948792513746,
-0.530705706757414));
#83784=CARTESIAN_POINT('Ctrl Pts',(-0.195109359192541,-0.010653541921629,
-0.531401901503512));
#83785=CARTESIAN_POINT('Ctrl Pts',(-0.195303342133092,-0.00710093120272025,
-0.531605611263834));
#83786=CARTESIAN_POINT('Ctrl Pts',(-0.195400086282404,-0.00354626374671888,
-0.531809321024156));
#83787=CARTESIAN_POINT('Ctrl Pts',(-0.195399999942242,4.75099905375869E-6,
-0.532013030784479));
#83788=CARTESIAN_POINT('',(-0.195399934316705,-0.000160215565585998,-0.602013030783437));
#83789=CARTESIAN_POINT('Ctrl Pts',(-0.19539999994224,4.75105306059038E-6,
-0.532013030787577));
#83790=CARTESIAN_POINT('Ctrl Pts',(-0.195399704441082,0.0121580412039381,
-0.532710224125548));
#83791=CARTESIAN_POINT('Ctrl Pts',(-0.194261233336228,0.0243536335351822,
-0.533407417463518));
#83792=CARTESIAN_POINT('Ctrl Pts',(-0.19198694281045,0.0363617077472572,
-0.534104610801489));
#83793=CARTESIAN_POINT('Ctrl Pts',(-0.189717397132364,0.0483447295385626,
-0.534800349586419));
#83794=CARTESIAN_POINT('Ctrl Pts',(-0.186316824434827,0.0601401463011918,
-0.535496088371348));
#83795=CARTESIAN_POINT('Ctrl Pts',(-0.181839233487673,0.0715237943947003,
-0.536191827156278));
#83796=CARTESIAN_POINT('Ctrl Pts',(-0.177362265235332,0.0829058593738311,
-0.536887469185399));
#83797=CARTESIAN_POINT('Ctrl Pts',(-0.171808852972938,0.0938754410502758,
-0.537583111214521));
#83798=CARTESIAN_POINT('Ctrl Pts',(-0.165282210432941,0.104225481118587,
-0.538278753243642));
#83799=CARTESIAN_POINT('Ctrl Pts',(-0.158755959389981,0.114574900345479,
-0.538974353545062));
#83800=CARTESIAN_POINT('Ctrl Pts',(-0.151257082255755,0.124304126911855,
-0.539669953846481));
#83801=CARTESIAN_POINT('Ctrl Pts',(-0.1429322553959,0.133234869187616,-0.540365554147901));
#83802=CARTESIAN_POINT('Ctrl Pts',(-0.134588349521748,0.142186079127443,
-0.541062748640806));
#83803=CARTESIAN_POINT('Ctrl Pts',(-0.12541535689199,0.150334556288951,
-0.541759943133711));
#83804=CARTESIAN_POINT('Ctrl Pts',(-0.115596060566579,0.157539553069976,
-0.542457137626616));
#83805=CARTESIAN_POINT('Ctrl Pts',(-0.112381743643222,0.159898086952496,
-0.542685362133052));
#83806=CARTESIAN_POINT('Ctrl Pts',(-0.109098407206999,0.162155865510001,
-0.542913586639488));
#83807=CARTESIAN_POINT('Ctrl Pts',(-0.105753080990153,0.164308995070538,
-0.543141811145924));
#83808=CARTESIAN_POINT('Ctrl Pts',(-0.0955410216455612,0.170881713371695,
-0.543838497224512));
#83809=CARTESIAN_POINT('Ctrl Pts',(-0.0846780241638187,0.17652181662486,
-0.544535183303101));
#83810=CARTESIAN_POINT('Ctrl Pts',(-0.0733582959045753,0.181106930905409,
-0.54523186938169));
#83811=CARTESIAN_POINT('Ctrl Pts',(-0.062062186213738,0.185682478363081,
-0.545927101827521));
#83812=CARTESIAN_POINT('Ctrl Pts',(-0.050312012500802,0.1892070123924,-0.546622334273352));
#83813=CARTESIAN_POINT('Ctrl Pts',(-0.0383252065753447,0.191604641230209,
-0.547317566719184));
#83814=CARTESIAN_POINT('Ctrl Pts',(-0.0263400560006732,0.194001938960899,
-0.548012703154987));
#83815=CARTESIAN_POINT('Ctrl Pts',(-0.0141191858681597,0.195272424626458,
-0.548707839590789));
#83816=CARTESIAN_POINT('Ctrl Pts',(-0.00189228080062207,0.195390837229824,
-0.549402976026592));
#83817=CARTESIAN_POINT('Ctrl Pts',(0.0103339899697718,0.195509243690281,
-0.550098076400689));
#83818=CARTESIAN_POINT('Ctrl Pts',(0.0225654198570891,0.194475714313942,
-0.550793176774786));
#83819=CARTESIAN_POINT('Ctrl Pts',(0.0345730017209927,0.192317101558858,
-0.551488277148883));
#83820=CARTESIAN_POINT('Ctrl Pts',(0.0466080158579125,0.190153557281749,
-0.552184965534909));
#83821=CARTESIAN_POINT('Ctrl Pts',(0.0584173120980081,0.186860017346395,
-0.552881653920935));
#83822=CARTESIAN_POINT('Ctrl Pts',(0.0697839543939136,0.182513998666262,
-0.55357834230696));
#83823=CARTESIAN_POINT('Ctrl Pts',(0.0733080235514968,0.181166576095002,
-0.553794340839308));
#83824=CARTESIAN_POINT('Ctrl Pts',(0.0767896917366288,0.179718335501842,
-0.554010339371656));
#83825=CARTESIAN_POINT('Ctrl Pts',(0.0802229488090808,0.178172496430778,
-0.554226337904004));
#83826=CARTESIAN_POINT('Ctrl Pts',(0.0912966463041234,0.173186515513026,
-0.554923023982593));
#83827=CARTESIAN_POINT('Ctrl Pts',(0.101942600437265,0.167146719192801,
-0.555619710061182));
#83828=CARTESIAN_POINT('Ctrl Pts',(0.111952417199804,0.160149356174544,
-0.556316396139771));
#83829=CARTESIAN_POINT('Ctrl Pts',(0.121941348519114,0.15316659312665,-0.557011628585602));
#83830=CARTESIAN_POINT('Ctrl Pts',(0.131296024692209,0.145230664944981,
-0.557706861031433));
#83831=CARTESIAN_POINT('Ctrl Pts',(0.139834390787362,0.136482611174931,
-0.558402093477264));
#83832=CARTESIAN_POINT('Ctrl Pts',(0.14837157775347,0.127735765491319,-0.559097229913067));
#83833=CARTESIAN_POINT('Ctrl Pts',(0.156092035764051,0.11817761040108,-0.55979236634887));
#83834=CARTESIAN_POINT('Ctrl Pts',(0.16284950311487,0.107987033181026,-0.560487502784673));
#83835=CARTESIAN_POINT('Ctrl Pts',(0.169606619907455,0.0977969846192045,
-0.56118260315877));
#83836=CARTESIAN_POINT('Ctrl Pts',(0.175400384209146,0.0869753232275042,
-0.561877703532867));
#83837=CARTESIAN_POINT('Ctrl Pts',(0.18012861229942,0.0757287463984798,
-0.562572803906964));
#83838=CARTESIAN_POINT('Ctrl Pts',(0.184867642401734,0.0644564758727907,
-0.56326949229299));
#83839=CARTESIAN_POINT('Ctrl Pts',(0.188535997983766,0.0527581832488236,
-0.563966180679016));
#83840=CARTESIAN_POINT('Ctrl Pts',(0.191080562372172,0.0408580308328046,
-0.564662869065041));
#83841=CARTESIAN_POINT('Ctrl Pts',(0.191869469126445,0.0371685542918895,
-0.564878867597389));
#83842=CARTESIAN_POINT('Ctrl Pts',(0.192550727476237,0.0334597402998151,
-0.565094866129736));
#83843=CARTESIAN_POINT('Ctrl Pts',(0.193123764929154,0.0297383829350012,
-0.565310864662084));
#83844=CARTESIAN_POINT('Ctrl Pts',(0.194972051635638,0.017735440871715,
-0.566007550740673));
#83845=CARTESIAN_POINT('Ctrl Pts',(0.19570354560059,0.00551740520414245,
-0.566704236819262));
#83846=CARTESIAN_POINT('Ctrl Pts',(0.195285492605467,-0.00668852583458686,
-0.567400922897851));
#83847=CARTESIAN_POINT('Ctrl Pts',(0.194868311876272,-0.0188689892463043,
-0.568096155343683));
#83848=CARTESIAN_POINT('Ctrl Pts',(0.193306300869942,-0.0310365298369193,
-0.568791387789514));
#83849=CARTESIAN_POINT('Ctrl Pts',(0.190618615664043,-0.0429616499022531,
-0.569486620235346));
#83850=CARTESIAN_POINT('Ctrl Pts',(0.187931301621392,-0.0548851231354774,
-0.570181756671149));
#83851=CARTESIAN_POINT('Ctrl Pts',(0.184118769834951,-0.0665653800675682,
-0.570876893106952));
#83852=CARTESIAN_POINT('Ctrl Pts',(0.179251411541754,-0.0777823338573007,
-0.571572029542756));
#83853=CARTESIAN_POINT('Ctrl Pts',(0.174384305753297,-0.0889987057432954,
-0.572267129916853));
#83854=CARTESIAN_POINT('Ctrl Pts',(0.168462855206484,-0.0997510303050761,
-0.57296223029095));
#83855=CARTESIAN_POINT('Ctrl Pts',(0.161604778916721,-0.109841046204403,
-0.573657330665048));
#83856=CARTESIAN_POINT('Ctrl Pts',(0.154731034807801,-0.119954113545231,
-0.574354019051074));
#83857=CARTESIAN_POINT('Ctrl Pts',(0.146916938705459,-0.129401165206762,
-0.5750507074371));
#83858=CARTESIAN_POINT('Ctrl Pts',(0.138321577373936,-0.138015583296909,
-0.575747395823126));
#83859=CARTESIAN_POINT('Ctrl Pts',(0.13565670528789,-0.140686363665592,
-0.575963394355472));
#83860=CARTESIAN_POINT('Ctrl Pts',(0.132916994470893,-0.143277386399193,
-0.576179392887818));
#83861=CARTESIAN_POINT('Ctrl Pts',(0.130107831562634,-0.145784471621875,
-0.576395391420164));
#83862=CARTESIAN_POINT('Ctrl Pts',(0.121047100133513,-0.153870875513176,
-0.577092077498753));
#83863=CARTESIAN_POINT('Ctrl Pts',(0.111197814895793,-0.161137722098923,
-0.577788763577342));
#83864=CARTESIAN_POINT('Ctrl Pts',(0.100732697291677,-0.167433818854923,
-0.578485449655931));
#83865=CARTESIAN_POINT('Ctrl Pts',(0.0902894151142026,-0.173716778829853,
-0.579180682101762));
#83866=CARTESIAN_POINT('Ctrl Pts',(0.0792335552777163,-0.179032499447423,
-0.579875914547594));
#83867=CARTESIAN_POINT('Ctrl Pts',(0.0677680355670711,-0.183272074674185,
-0.580571146993425));
#83868=CARTESIAN_POINT('Ctrl Pts',(0.0563040992187653,-0.187511064425198,
-0.581266283429228));
#83869=CARTESIAN_POINT('Ctrl Pts',(0.0444314189991363,-0.19067385828896,
-0.581961419865031));
#83870=CARTESIAN_POINT('Ctrl Pts',(0.0323729195949517,-0.192699647319083,
-0.582656556300834));
#83871=CARTESIAN_POINT('Ctrl Pts',(0.0203150457515041,-0.194725331257018,
-0.583351656674931));
#83872=CARTESIAN_POINT('Ctrl Pts',(0.00807223922603621,-0.195614009173991,
-0.584046757049028));
#83873=CARTESIAN_POINT('Ctrl Pts',(-0.00412510867143945,-0.195356452359396,
-0.584741857423125));
#83874=CARTESIAN_POINT('Ctrl Pts',(-0.0163503223774861,-0.195098307135831,
-0.58543854580915));
#83875=CARTESIAN_POINT('Ctrl Pts',(-0.0285289974000453,-0.193688783213689,
-0.586135234195176));
#83876=CARTESIAN_POINT('Ctrl Pts',(-0.0404347559278585,-0.191170579622113,
-0.586831922581202));
#83877=CARTESIAN_POINT('Ctrl Pts',(-0.0441259705656679,-0.190389845665809,
-0.58704792111355));
#83878=CARTESIAN_POINT('Ctrl Pts',(-0.0477910435399655,-0.189502910346834,
-0.587263919645897));
#83879=CARTESIAN_POINT('Ctrl Pts',(-0.051423535777776,-0.188512015447588,
-0.587479918178244));
#83880=CARTESIAN_POINT('Ctrl Pts',(-0.0631398504450944,-0.185315962797851,
-0.588176604256832));
#83881=CARTESIAN_POINT('Ctrl Pts',(-0.0745981850498335,-0.181012238006438,
-0.58887329033542));
#83882=CARTESIAN_POINT('Ctrl Pts',(-0.0855776747297964,-0.175663375772644,
-0.589569976414008));
#83883=CARTESIAN_POINT('Ctrl Pts',(-0.0965342557478107,-0.170325673918822,
-0.590265208859839));
#83884=CARTESIAN_POINT('Ctrl Pts',(-0.107013163827437,-0.163947476064685,
-0.590960441305669));
#83885=CARTESIAN_POINT('Ctrl Pts',(-0.116812557614591,-0.156639670529332,
-0.5916556737515));
#83886=CARTESIAN_POINT('Ctrl Pts',(-0.126610598127626,-0.149332874185397,
-0.592350810187302));
#83887=CARTESIAN_POINT('Ctrl Pts',(-0.135728583186761,-0.141097210940505,
-0.593045946623104));
#83888=CARTESIAN_POINT('Ctrl Pts',(-0.143994117112832,-0.132086540710611,
-0.593741083058906));
#83889=CARTESIAN_POINT('Ctrl Pts',(-0.152259222246454,-0.123076337928724,
-0.594436183433003));
#83890=CARTESIAN_POINT('Ctrl Pts',(-0.159671392506933,-0.113291871050581,
-0.595131283807099));
#83891=CARTESIAN_POINT('Ctrl Pts',(-0.166097428106162,-0.102921350440607,
-0.595826384181195));
#83892=CARTESIAN_POINT('Ctrl Pts',(-0.172538144493329,-0.0925271375538757,
-0.59652307256722));
#83893=CARTESIAN_POINT('Ctrl Pts',(-0.177987823682078,-0.0815449756659985,
-0.597219760953245));
#83894=CARTESIAN_POINT('Ctrl Pts',(-0.182359004728149,-0.0701879861127176,
-0.59791644933927));
#83895=CARTESIAN_POINT('Ctrl Pts',(-0.183714228540592,-0.0666669096535048,
-0.598132447871621));
#83896=CARTESIAN_POINT('Ctrl Pts',(-0.184966142778584,-0.0631099270968684,
-0.598348446403973));
#83897=CARTESIAN_POINT('Ctrl Pts',(-0.186113121297839,-0.0595236598402349,
-0.598564444936324));
#83898=CARTESIAN_POINT('Ctrl Pts',(-0.190528317054616,-0.0457186306192422,
-0.599395912821293));
#83899=CARTESIAN_POINT('Ctrl Pts',(-0.193410026225108,-0.0314006634720892,
-0.600227380706261));
#83900=CARTESIAN_POINT('Ctrl Pts',(-0.194669066429944,-0.0168853361024844,
-0.601058848591229));
#83901=CARTESIAN_POINT('Ctrl Pts',(-0.195150686050878,-0.0113327997826631,
-0.601376909321965));
#83902=CARTESIAN_POINT('Ctrl Pts',(-0.19539534973394,-0.00575160219395176,
-0.601694970052701));
#83903=CARTESIAN_POINT('Ctrl Pts',(-0.195399934316705,-0.000160215565585217,
-0.602013030783437));
#83904=CARTESIAN_POINT('',(-0.19539996230052,0.000121379385344387,-0.672013030792617));
#83905=CARTESIAN_POINT('Ctrl Pts',(-0.195399934316764,-0.000160215492812403,
-0.602013030787577));
#83906=CARTESIAN_POINT('Ctrl Pts',(-0.195409913750772,0.0120107719400208,
-0.602705365876152));
#83907=CARTESIAN_POINT('Ctrl Pts',(-0.194278398116146,0.0241993431608203,
-0.603397700964727));
#83908=CARTESIAN_POINT('Ctrl Pts',(-0.19202192620965,0.0361765097091413,
-0.604090036053301));
#83909=CARTESIAN_POINT('Ctrl Pts',(-0.189766351259512,0.0481489152871848,
-0.604782095935986));
#83910=CARTESIAN_POINT('Ctrl Pts',(-0.186386880787103,0.0599092164680677,
-0.605474155818671));
#83911=CARTESIAN_POINT('Ctrl Pts',(-0.181951258354798,0.0712383294519561,
-0.606166215701356));
#83912=CARTESIAN_POINT('Ctrl Pts',(-0.177504766240249,0.082595204911151,
-0.606859971506346));
#83913=CARTESIAN_POINT('Ctrl Pts',(-0.171997315619093,0.0935179720006077,
-0.607553727311336));
#83914=CARTESIAN_POINT('Ctrl Pts',(-0.165544577333922,0.103808250709339,
-0.608247483116325));
#83915=CARTESIAN_POINT('Ctrl Pts',(-0.161199417774438,0.110737541953609,
-0.608714645975685));
#83916=CARTESIAN_POINT('Ctrl Pts',(-0.156426621585289,0.117380524878914,
-0.609181808835044));
#83917=CARTESIAN_POINT('Ctrl Pts',(-0.151271963941549,0.123684893682562,
-0.609648971694404));
#83918=CARTESIAN_POINT('Ctrl Pts',(-0.143584755619367,0.133086681285734,
-0.610345657772992));
#83919=CARTESIAN_POINT('Ctrl Pts',(-0.134990715424245,0.141802067227806,
-0.611042343851581));
#83920=CARTESIAN_POINT('Ctrl Pts',(-0.125636843254467,0.149654748060502,
-0.611739029930169));
#83921=CARTESIAN_POINT('Ctrl Pts',(-0.116302487902111,0.157491044305586,
-0.612434262376));
#83922=CARTESIAN_POINT('Ctrl Pts',(-0.106212063419679,0.164467594754932,
-0.613129494821831));
#83923=CARTESIAN_POINT('Ctrl Pts',(-0.0955489974396641,0.17044514979393,
-0.613824727267662));
#83924=CARTESIAN_POINT('Ctrl Pts',(-0.0848874040049419,0.176421879346097,
-0.614519863703464));
#83925=CARTESIAN_POINT('Ctrl Pts',(-0.0736540659606052,0.181399420606974,
-0.615215000139267));
#83926=CARTESIAN_POINT('Ctrl Pts',(-0.0620596813029653,0.18528290789108,
-0.615910136575069));
#83927=CARTESIAN_POINT('Ctrl Pts',(-0.050465898129107,0.189166193710883,
-0.616605236949166));
#83928=CARTESIAN_POINT('Ctrl Pts',(-0.0385119437893241,0.191955285982993,
-0.617300337323262));
#83929=CARTESIAN_POINT('Ctrl Pts',(-0.0264239439058242,0.193605101142666,
-0.617995437697359));
#83930=CARTESIAN_POINT('Ctrl Pts',(-0.0143083280279611,0.195258685435908,
-0.618692126083384));
#83931=CARTESIAN_POINT('Ctrl Pts',(-0.00205893035789418,0.195767743107061,
-0.61938881446941));
#83932=CARTESIAN_POINT('Ctrl Pts',(0.0100939809641747,0.195139108197959,
-0.620085502855435));
#83933=CARTESIAN_POINT('Ctrl Pts',(0.0138618218841569,0.194944208698451,
-0.620301501387785));
#83934=CARTESIAN_POINT('Ctrl Pts',(0.0176204215183335,0.194640328858322,
-0.620517499920135));
#83935=CARTESIAN_POINT('Ctrl Pts',(0.0213630697655697,0.194228677723428,
-0.620733498452485));
#83936=CARTESIAN_POINT('Ctrl Pts',(0.0334346838757103,0.192900929743878,
-0.621430184531068));
#83937=CARTESIAN_POINT('Ctrl Pts',(0.0454244076356298,0.190438816189816,
-0.622126870609651));
#83938=CARTESIAN_POINT('Ctrl Pts',(0.0571043215712217,0.186869624224727,
-0.622823556688234));
#83939=CARTESIAN_POINT('Ctrl Pts',(0.0687598654124098,0.183307879364608,
-0.623518789134059));
#83940=CARTESIAN_POINT('Ctrl Pts',(0.0801060324371824,0.178643823591831,
-0.624214021579884));
#83941=CARTESIAN_POINT('Ctrl Pts',(0.0909261445995594,0.172955474698721,
-0.62490925402571));
#83942=CARTESIAN_POINT('Ctrl Pts',(0.101744762528922,0.167267911353726,
-0.625604390461507));
#83943=CARTESIAN_POINT('Ctrl Pts',(0.112036675421449,0.160556702101101,
-0.626299526897304));
#83944=CARTESIAN_POINT('Ctrl Pts',(0.12160758126088,0.15294690640833,-0.626994663333101));
#83945=CARTESIAN_POINT('Ctrl Pts',(0.131177990588873,0.145337505490166,
-0.627689763707192));
#83946=CARTESIAN_POINT('Ctrl Pts',(0.14002679907744,0.136830176391645,-0.628384864081283));
#83947=CARTESIAN_POINT('Ctrl Pts',(0.147993057312752,0.127590026989669,
-0.629079964455375));
#83948=CARTESIAN_POINT('Ctrl Pts',(0.155977515096758,0.118328767733604,
-0.629776652841395));
#83949=CARTESIAN_POINT('Ctrl Pts',(0.16307487608635,0.108332050773861,-0.630473341227415));
#83950=CARTESIAN_POINT('Ctrl Pts',(0.169165479860222,0.0977967301276523,
-0.631170029613435));
#83951=CARTESIAN_POINT('Ctrl Pts',(0.171053786745825,0.0945304006705272,
-0.631386028145812));
#83952=CARTESIAN_POINT('Ctrl Pts',(0.172845656334852,0.0912124769904705,
-0.631602026678188));
#83953=CARTESIAN_POINT('Ctrl Pts',(0.174538448708856,0.0878492454282104,
-0.631818025210564));
#83954=CARTESIAN_POINT('Ctrl Pts',(0.179998415811227,0.0770014096453982,
-0.632514711289167));
#83955=CARTESIAN_POINT('Ctrl Pts',(0.184462364392482,0.0656045398091443,
-0.633211397367771));
#83956=CARTESIAN_POINT('Ctrl Pts',(0.187829067619882,0.053864657773402,
-0.633908083446374));
#83957=CARTESIAN_POINT('Ctrl Pts',(0.191188746234265,0.0421492709552665,
-0.63460331589222));
#83958=CARTESIAN_POINT('Ctrl Pts',(0.19345541392759,0.0300931048987756,
-0.635298548338066));
#83959=CARTESIAN_POINT('Ctrl Pts',(0.19457651462254,0.017920378270127,-0.635993780783911));
#83960=CARTESIAN_POINT('Ctrl Pts',(0.19569746049602,0.00574933266749327,
-0.636688917219729));
#83961=CARTESIAN_POINT('Ctrl Pts',(0.195673028155159,-0.00653737574804703,
-0.637384053655546));
#83962=CARTESIAN_POINT('Ctrl Pts',(0.194502301584276,-0.018708679227013,
-0.638079190091363));
#83963=CARTESIAN_POINT('Ctrl Pts',(0.193331635747367,-0.0308793512932791,
-0.638774290465474));
#83964=CARTESIAN_POINT('Ctrl Pts',(0.191014904436083,-0.0429337619423767,
-0.639469390839585));
#83965=CARTESIAN_POINT('Ctrl Pts',(0.187602943526061,-0.0546470088875656,
-0.640164491213696));
#83966=CARTESIAN_POINT('Ctrl Pts',(0.184183187720758,-0.0663870156743068,
-0.640861179599736));
#83967=CARTESIAN_POINT('Ctrl Pts',(0.179663514437599,-0.0777834816358084,
-0.641557867985775));
#83968=CARTESIAN_POINT('Ctrl Pts',(0.174143869845266,-0.0886288474217898,
-0.642254556371815));
#83969=CARTESIAN_POINT('Ctrl Pts',(0.172432580903867,-0.0919913020553304,
-0.642470554904092));
#83970=CARTESIAN_POINT('Ctrl Pts',(0.170625503544467,-0.0953009675331104,
-0.642686553436368));
#83971=CARTESIAN_POINT('Ctrl Pts',(0.168726472737284,-0.0985522064574634,
-0.642902551968645));
#83972=CARTESIAN_POINT('Ctrl Pts',(0.162601299977015,-0.109038818902745,
-0.643599238047224));
#83973=CARTESIAN_POINT('Ctrl Pts',(0.155473255404872,-0.118989017874075,
-0.644295924125804));
#83974=CARTESIAN_POINT('Ctrl Pts',(0.147460012514969,-0.128205712466665,
-0.644992610204383));
#83975=CARTESIAN_POINT('Ctrl Pts',(0.139463489224775,-0.137403176462311,
-0.645687842650206));
#83976=CARTESIAN_POINT('Ctrl Pts',(0.130585946322826,-0.145869471663221,
-0.646383075096028));
#83977=CARTESIAN_POINT('Ctrl Pts',(0.120986823116204,-0.153438419674632,
-0.64707830754185));
#83978=CARTESIAN_POINT('Ctrl Pts',(0.111389025526781,-0.161006322431444,
-0.647773443977645));
#83979=CARTESIAN_POINT('Ctrl Pts',(0.101070503411513,-0.167676547463309,
-0.648468580413439));
#83980=CARTESIAN_POINT('Ctrl Pts',(0.0902245611554579,-0.173322498725079,
-0.649163716849233));
#83981=CARTESIAN_POINT('Ctrl Pts',(0.0793791815561055,-0.178968157090921,
-0.649858817223322));
#83982=CARTESIAN_POINT('Ctrl Pts',(0.0680072247396998,-0.183589267154824,
-0.650553917597411));
#83983=CARTESIAN_POINT('Ctrl Pts',(0.0563250053900924,-0.187105996076572,
-0.6512490179715));
#83984=CARTESIAN_POINT('Ctrl Pts',(0.0446160970839333,-0.190630759244432,
-0.651945706357518));
#83985=CARTESIAN_POINT('Ctrl Pts',(0.032596367224158,-0.193045914950913,
-0.652642394743536));
#83986=CARTESIAN_POINT('Ctrl Pts',(0.0204943274429066,-0.194322264660185,
-0.653339083129553));
#83987=CARTESIAN_POINT('Ctrl Pts',(0.0167422585349957,-0.194717979113809,
-0.653555081661944));
#83988=CARTESIAN_POINT('Ctrl Pts',(0.0129823039122766,-0.195004606760184,
-0.653771080194334));
#83989=CARTESIAN_POINT('Ctrl Pts',(0.00922128015307064,-0.195182294259337,
-0.653987078726724));
#83990=CARTESIAN_POINT('Ctrl Pts',(-0.0029096027059849,-0.195755411148715,
-0.65468376480528));
#83991=CARTESIAN_POINT('Ctrl Pts',(-0.0151366931140761,-0.195195286936917,
-0.655380450883835));
#83992=CARTESIAN_POINT('Ctrl Pts',(-0.0272306062261563,-0.193493292091886,
-0.656077136962391));
#83993=CARTESIAN_POINT('Ctrl Pts',(-0.039299285436176,-0.191794848452394,
-0.656772369408188));
#83994=CARTESIAN_POINT('Ctrl Pts',(-0.0512344707610213,-0.188959310821571,
-0.657467601853986));
#83995=CARTESIAN_POINT('Ctrl Pts',(-0.0628099610316357,-0.18502991324433,
-0.658162834299783));
#83996=CARTESIAN_POINT('Ctrl Pts',(-0.0743838527532299,-0.181101058308006,
-0.658857970735553));
#83997=CARTESIAN_POINT('Ctrl Pts',(-0.0855973061772885,-0.176078881198892,
-0.659553107171322));
#83998=CARTESIAN_POINT('Ctrl Pts',(-0.0962388777946769,-0.170056574118207,
-0.660248243607091));
#83999=CARTESIAN_POINT('Ctrl Pts',(-0.106879897357519,-0.164034579457729,
-0.660943343981155));
#84000=CARTESIAN_POINT('Ctrl Pts',(-0.11694834584246,-0.157013012314087,
-0.661638444355218));
#84001=CARTESIAN_POINT('Ctrl Pts',(-0.126259471152442,-0.149129829156697,
-0.662333544729281));
#84002=CARTESIAN_POINT('Ctrl Pts',(-0.135591868466614,-0.141228636242208,
-0.663030233115274));
#84003=CARTESIAN_POINT('Ctrl Pts',(-0.144162863554939,-0.132462512459477,
-0.663726921501266));
#84004=CARTESIAN_POINT('Ctrl Pts',(-0.151823530936729,-0.123007217080561,
-0.664423609887259));
#84005=CARTESIAN_POINT('Ctrl Pts',(-0.154198614181723,-0.120075734415706,
-0.664639608419774));
#84006=CARTESIAN_POINT('Ctrl Pts',(-0.156486497327773,-0.117078234641055,
-0.664855606952289));
#84007=CARTESIAN_POINT('Ctrl Pts',(-0.158683591420661,-0.114020514881493,
-0.665071605484804));
#84008=CARTESIAN_POINT('Ctrl Pts',(-0.165825731652837,-0.104080720594039,
-0.665773756482416));
#84009=CARTESIAN_POINT('Ctrl Pts',(-0.172055164421404,-0.0934329165091907,
-0.666475907480027));
#84010=CARTESIAN_POINT('Ctrl Pts',(-0.177237810842229,-0.0822673593100837,
-0.667178058477638));
#84011=CARTESIAN_POINT('Ctrl Pts',(-0.182408615182921,-0.0711273148340792,
-0.667878605096386));
#84012=CARTESIAN_POINT('Ctrl Pts',(-0.186536952766617,-0.0594726009180445,
-0.668579151715133));
#84013=CARTESIAN_POINT('Ctrl Pts',(-0.189533861475579,-0.0475192103696621,
-0.66927969833388));
#84014=CARTESIAN_POINT('Ctrl Pts',(-0.192527619210319,-0.0355783877134433,
-0.669979508392207));
#84015=CARTESIAN_POINT('Ctrl Pts',(-0.194392063214706,-0.0233403297780268,
-0.670679318450535));
#84016=CARTESIAN_POINT('Ctrl Pts',(-0.195088109560349,-0.011035828386175,
-0.671379128508862));
#84017=CARTESIAN_POINT('Ctrl Pts',(-0.195298273903919,-0.00732060529198014,
-0.671590429268434));
#84018=CARTESIAN_POINT('Ctrl Pts',(-0.195402273579095,-0.0035993848560569,
-0.671801730028005));
#84019=CARTESIAN_POINT('Ctrl Pts',(-0.195399962300576,0.000121379296588555,
-0.672013030787577));
#84020=CARTESIAN_POINT('',(-0.195399988273324,6.76962695950741E-5,-0.742013030783604));
#84021=CARTESIAN_POINT('Ctrl Pts',(-0.19539996230052,0.000121379385344218,
-0.672013030792617));
#84022=CARTESIAN_POINT('Ctrl Pts',(-0.195391368601875,0.0139557581525191,
-0.672798679821104));
#84023=CARTESIAN_POINT('Ctrl Pts',(-0.193909385686024,0.0277341230872606,
-0.673584328849591));
#84024=CARTESIAN_POINT('Ctrl Pts',(-0.191013872295133,0.0411686845893673,
-0.674369977878078));
#84025=CARTESIAN_POINT('Ctrl Pts',(-0.188819578705173,0.0513497365163667,
-0.674965362666347));
#84026=CARTESIAN_POINT('Ctrl Pts',(-0.185814593619475,0.061333606866596,
-0.675560747454616));
#84027=CARTESIAN_POINT('Ctrl Pts',(-0.182043323198772,0.0710027357131215,
-0.676156132242885));
#84028=CARTESIAN_POINT('Ctrl Pts',(-0.177630392851685,0.0823170111049079,
-0.676852818321381));
#84029=CARTESIAN_POINT('Ctrl Pts',(-0.172143144054868,0.0932580156109927,
-0.677549504399877));
#84030=CARTESIAN_POINT('Ctrl Pts',(-0.165667038205755,0.103612704105882,
-0.678246190478373));
#84031=CARTESIAN_POINT('Ctrl Pts',(-0.159204444725966,0.113945787584046,
-0.678941422924112));
#84032=CARTESIAN_POINT('Ctrl Pts',(-0.151757486287423,0.12369420963015,
-0.679636655369852));
#84033=CARTESIAN_POINT('Ctrl Pts',(-0.143457703961445,0.132668938241437,
-0.680331887815592));
#84034=CARTESIAN_POINT('Ctrl Pts',(-0.135159067816597,0.141642427463043,
-0.681027024251306));
#84035=CARTESIAN_POINT('Ctrl Pts',(-0.126008401467838,0.149841763165552,
-0.681722160687021));
#84036=CARTESIAN_POINT('Ctrl Pts',(-0.116176875309522,0.157111723443274,
-0.682417297122735));
#84037=CARTESIAN_POINT('Ctrl Pts',(-0.106345859182866,0.1643813065761,-0.683112397496745));
#84038=CARTESIAN_POINT('Ctrl Pts',(-0.095834772975827,0.170721111523679,
-0.683807497870755));
#84039=CARTESIAN_POINT('Ctrl Pts',(-0.0848448157757491,0.176018513901178,
-0.684502598244765));
#84040=CARTESIAN_POINT('Ctrl Pts',(-0.0738297511468309,0.181328018614547,
-0.685199286630709));
#84041=CARTESIAN_POINT('Ctrl Pts',(-0.0623344474413148,0.185590045793406,
-0.685895975016652));
#84042=CARTESIAN_POINT('Ctrl Pts',(-0.0505800560208747,0.18874008035636,
-0.686592663402595));
#84043=CARTESIAN_POINT('Ctrl Pts',(-0.0469357706389397,0.189716704708889,
-0.686808661935385));
#84044=CARTESIAN_POINT('Ctrl Pts',(-0.0432666659218911,0.190586810909412,
-0.687024660468175));
#84045=CARTESIAN_POINT('Ctrl Pts',(-0.0395794977631675,0.191349479635601,
-0.687240659000965));
#84046=CARTESIAN_POINT('Ctrl Pts',(-0.0276868302910744,0.193809406918948,
-0.687937345079373));
#84047=CARTESIAN_POINT('Ctrl Pts',(-0.0155222166564679,0.195165007905675,
-0.688634031157782));
#84048=CARTESIAN_POINT('Ctrl Pts',(-0.00331088189918468,0.195371947989085,
-0.68933071723619));
#84049=CARTESIAN_POINT('Ctrl Pts',(0.00887497395619728,0.195578456292825,
-0.690025949681839));
#84050=CARTESIAN_POINT('Ctrl Pts',(0.0211064925116929,0.194640972341691,
-0.690721182127487));
#84051=CARTESIAN_POINT('Ctrl Pts',(0.0331534965784134,0.192566886210026,
-0.691416414573135));
#84052=CARTESIAN_POINT('Ctrl Pts',(0.0451988369811046,0.190493086504967,
-0.692111551008754));
#84053=CARTESIAN_POINT('Ctrl Pts',(0.0570588448093164,0.18728309976618,
-0.692806687444373));
#84054=CARTESIAN_POINT('Ctrl Pts',(0.068510120264012,0.182995965587798,
-0.693501823879992));
#84055=CARTESIAN_POINT('Ctrl Pts',(0.0799608016590144,0.178709053813778,
-0.694196924253904));
#84056=CARTESIAN_POINT('Ctrl Pts',(0.0910019828272812,0.173345437645973,
-0.694892024627817));
#84057=CARTESIAN_POINT('Ctrl Pts',(0.101429639641313,0.167012539056903,
-0.695587125001729));
#84058=CARTESIAN_POINT('Ctrl Pts',(0.111881119264334,0.160665172458755,
-0.696283813387573));
#84059=CARTESIAN_POINT('Ctrl Pts',(0.121715563002558,0.153344612420341,
-0.696980501773416));
#84060=CARTESIAN_POINT('Ctrl Pts',(0.130758432397035,0.145201213345723,
-0.69767719015926));
#84061=CARTESIAN_POINT('Ctrl Pts',(0.133562048138837,0.142676465852265,
-0.697893188692521));
#84062=CARTESIAN_POINT('Ctrl Pts',(0.136289839376129,0.140072897291044,
-0.698109187225783));
#84063=CARTESIAN_POINT('Ctrl Pts',(0.138937356130358,0.137395673408976,
-0.698325185759044));
#84064=CARTESIAN_POINT('Ctrl Pts',(0.147476710724727,0.128760500837933,
-0.699021871838344));
#84065=CARTESIAN_POINT('Ctrl Pts',(0.15523792299337,0.119295879165266,-0.699718557917643));
#84066=CARTESIAN_POINT('Ctrl Pts',(0.162061162106512,0.109166568768497,
-0.700415243996942));
#84067=CARTESIAN_POINT('Ctrl Pts',(0.168870164558155,0.0990583931379199,
-0.701110476443485));
#84068=CARTESIAN_POINT('Ctrl Pts',(0.174744533221545,0.0882889588215705,
-0.701805708890027));
#84069=CARTESIAN_POINT('Ctrl Pts',(0.179565123563313,0.0770553463407453,
-0.70250094133657));
#84070=CARTESIAN_POINT('Ctrl Pts',(0.184385048192392,0.0658232851965483,
-0.703196077773075));
#84071=CARTESIAN_POINT('Ctrl Pts',(0.188151097207593,0.0541279581078693,
-0.70389121420958));
#84072=CARTESIAN_POINT('Ctrl Pts',(0.19079113664295,0.0421888869074672,
-0.704586350646084));
#84073=CARTESIAN_POINT('Ctrl Pts',(0.193431039120533,0.0302504350722879,
-0.705281451020878));
#84074=CARTESIAN_POINT('Ctrl Pts',(0.194944885479764,0.0180691244063143,
-0.705976551395672));
#84075=CARTESIAN_POINT('Ctrl Pts',(0.19531167246024,0.00587457239158232,
-0.706671651770466));
#84076=CARTESIAN_POINT('Ctrl Pts',(0.19567929739465,-0.00634783904393062,
-0.707368340157169));
#84077=CARTESIAN_POINT('Ctrl Pts',(0.194894670464553,-0.0185826763482537,
-0.708065028543872));
#84078=CARTESIAN_POINT('Ctrl Pts',(0.192988853477866,-0.0306016737009374,
-0.708761716930575));
#84079=CARTESIAN_POINT('Ctrl Pts',(0.192397981470756,-0.0343279963955332,
-0.708977715459425));
#84080=CARTESIAN_POINT('Ctrl Pts',(0.191699709787446,-0.0380336448360147,
-0.709193713988275));
#84081=CARTESIAN_POINT('Ctrl Pts',(0.190895947856836,-0.0417120736938359,
-0.709409712517125));
#84082=CARTESIAN_POINT('Ctrl Pts',(0.188303477667904,-0.0535765534518853,
-0.710106398594895));
#84083=CARTESIAN_POINT('Ctrl Pts',(0.184591587771128,-0.0652400585887095,
-0.710803084672665));
#84084=CARTESIAN_POINT('Ctrl Pts',(0.179811431707822,-0.0764788142375607,
-0.711499770750434));
#84085=CARTESIAN_POINT('Ctrl Pts',(0.175041249421265,-0.0876941202671337,
-0.712195003195454));
#84086=CARTESIAN_POINT('Ctrl Pts',(0.169207496290184,-0.0984856098079502,
-0.712890235640474));
#84087=CARTESIAN_POINT('Ctrl Pts',(0.162410589384586,-0.108646032857861,
-0.713585468085493));
#84088=CARTESIAN_POINT('Ctrl Pts',(0.155614621116236,-0.118805052776662,
-0.714280604520508));
#84089=CARTESIAN_POINT('Ctrl Pts',(0.147856211198137,-0.128332427854005,
-0.714975740955522));
#84090=CARTESIAN_POINT('Ctrl Pts',(0.139280198443431,-0.137048116811427,
-0.715670877390536));
#84091=CARTESIAN_POINT('Ctrl Pts',(0.130704630587781,-0.14576335362379,
-0.716365977763857));
#84092=CARTESIAN_POINT('Ctrl Pts',(0.121312177063685,-0.153666383203982,
-0.717061078137178));
#84093=CARTESIAN_POINT('Ctrl Pts',(0.111283987381547,-0.16061455149663,
-0.717756178510498));
#84094=CARTESIAN_POINT('Ctrl Pts',(0.101232887504312,-0.167578593431102,
-0.71845286689578));
#84095=CARTESIAN_POINT('Ctrl Pts',(0.0905439078716308,-0.173582974921055,
-0.719149555281062));
#84096=CARTESIAN_POINT('Ctrl Pts',(0.0794254163071088,-0.178529446435154,
-0.719846243666344));
#84097=CARTESIAN_POINT('Ctrl Pts',(0.0759782827616286,-0.180063031075576,
-0.720062242202631));
#84098=CARTESIAN_POINT('Ctrl Pts',(0.0724900049008866,-0.181495278347787,
-0.720278240738918));
#84099=CARTESIAN_POINT('Ctrl Pts',(0.0689671122597918,-0.182824225491441,
-0.720494239275204));
#84100=CARTESIAN_POINT('Ctrl Pts',(0.0576043025921026,-0.187110638672362,
-0.721190925352916));
#84101=CARTESIAN_POINT('Ctrl Pts',(0.045800477050706,-0.19034872162001,
-0.721887611430628));
#84102=CARTESIAN_POINT('Ctrl Pts',(0.033771177704092,-0.192459521864933,
-0.72258429750834));
#84103=CARTESIAN_POINT('Ctrl Pts',(0.021766977443515,-0.194565917933401,
-0.723279529953276));
#84104=CARTESIAN_POINT('Ctrl Pts',(0.00953907767813231,-0.19554947746548,
-0.723974762398212));
#84105=CARTESIAN_POINT('Ctrl Pts',(-0.00268401299032918,-0.195381565338872,
-0.724669994843147));
#84106=CARTESIAN_POINT('Ctrl Pts',(-0.0149054156773831,-0.195213676400551,
-0.725365131278042));
#84107=CARTESIAN_POINT('Ctrl Pts',(-0.0271211364012227,-0.193894598142963,
-0.726060267712936));
#84108=CARTESIAN_POINT('Ctrl Pts',(-0.0391012974787524,-0.191447769732317,
-0.72675540414783));
#84109=CARTESIAN_POINT('Ctrl Pts',(-0.0510808370593697,-0.189001068256216,
-0.72745050452101));
#84110=CARTESIAN_POINT('Ctrl Pts',(-0.0628239893884408,-0.185426934365536,
-0.72814560489419));
#84111=CARTESIAN_POINT('Ctrl Pts',(-0.0741124615666403,-0.180799621240016,
-0.72884070526737));
#84112=CARTESIAN_POINT('Ctrl Pts',(-0.0854267231548624,-0.176161736650651,
-0.729537393652484));
#84113=CARTESIAN_POINT('Ctrl Pts',(-0.0962834466948086,-0.170466261552371,
-0.730234082037597));
#84114=CARTESIAN_POINT('Ctrl Pts',(-0.106486760934479,-0.163834458358683,
-0.730930770422711));
#84115=CARTESIAN_POINT('Ctrl Pts',(-0.10965015649836,-0.161778360084078,
-0.731146768959569));
#84116=CARTESIAN_POINT('Ctrl Pts',(-0.112750962585627,-0.159632569700436,
-0.731362767496427));
#84117=CARTESIAN_POINT('Ctrl Pts',(-0.115783977319435,-0.157401494897896,
-0.731578766033286));
#84118=CARTESIAN_POINT('Ctrl Pts',(-0.125482540042977,-0.150267266807228,
-0.732269456828343));
#84119=CARTESIAN_POINT('Ctrl Pts',(-0.134556120011492,-0.1422059751907,
-0.7329601476234));
#84120=CARTESIAN_POINT('Ctrl Pts',(-0.142822838970763,-0.133352152844758,
-0.733650838418457));
#84121=CARTESIAN_POINT('Ctrl Pts',(-0.15116326841965,-0.124419385081255,
-0.734347687782219));
#84122=CARTESIAN_POINT('Ctrl Pts',(-0.158681612033931,-0.114680408755922,
-0.735044537145981));
#84123=CARTESIAN_POINT('Ctrl Pts',(-0.165226227850539,-0.104314206272596,
-0.735741386509744));
#84124=CARTESIAN_POINT('Ctrl Pts',(-0.17169835600434,-0.0940628190528786,
-0.736430517623402));
#84125=CARTESIAN_POINT('Ctrl Pts',(-0.177217764800105,-0.0831988186608179,
-0.73711964873706));
#84126=CARTESIAN_POINT('Ctrl Pts',(-0.181680927325022,-0.0719249653897735,
-0.737808779850718));
#84127=CARTESIAN_POINT('Ctrl Pts',(-0.186219070801908,-0.0604617118345347,
-0.738509488339532));
#84128=CARTESIAN_POINT('Ctrl Pts',(-0.189664727549586,-0.0485755602974442,
-0.739210196828347));
#84129=CARTESIAN_POINT('Ctrl Pts',(-0.191961028025369,-0.0364982700883675,
-0.739910905317161));
#84130=CARTESIAN_POINT('Ctrl Pts',(-0.194257328501152,-0.0244209798792907,
-0.740611613805975));
#84131=CARTESIAN_POINT('Ctrl Pts',(-0.195404222307629,-0.012153512645485,
-0.74131232229479));
#84132=CARTESIAN_POINT('Ctrl Pts',(-0.195399988273324,6.76962695950502E-5,
-0.742013030783604));
#84133=CARTESIAN_POINT('',(-0.195399921197426,-0.00017548800484569,-0.812013030784603));
#84134=CARTESIAN_POINT('Ctrl Pts',(-0.1953999882733,6.76963388894689E-5,
-0.742013030787577));
#84135=CARTESIAN_POINT('Ctrl Pts',(-0.195398678534898,0.00384814994386311,
-0.742229784788839));
#84136=CARTESIAN_POINT('Ctrl Pts',(-0.195287664303936,0.00762655792512721,
-0.742446538790102));
#84137=CARTESIAN_POINT('Ctrl Pts',(-0.195067254895793,0.0113985116317773,
-0.742663292791365));
#84138=CARTESIAN_POINT('Ctrl Pts',(-0.194358819693395,0.0235222445074034,
-0.743359978863201));
#84139=CARTESIAN_POINT('Ctrl Pts',(-0.192513314931336,0.0356222275051059,
-0.744056664935038));
#84140=CARTESIAN_POINT('Ctrl Pts',(-0.189546331861466,0.0474694436228498,
-0.744753351006874));
#84141=CARTESIAN_POINT('Ctrl Pts',(-0.186585539389951,0.0592919405713621,
-0.745448583445996));
#84142=CARTESIAN_POINT('Ctrl Pts',(-0.182508052018168,0.0708618591793415,
-0.746143815885119));
#84143=CARTESIAN_POINT('Ctrl Pts',(-0.1773807002981,0.0819588138137424,
-0.746839048324241));
#84144=CARTESIAN_POINT('Ctrl Pts',(-0.172254056652507,0.0930542359864036,
-0.747534184753499));
#84145=CARTESIAN_POINT('Ctrl Pts',(-0.166078161760922,0.103676011751318,
-0.748229321182757));
#84146=CARTESIAN_POINT('Ctrl Pts',(-0.158967970989733,0.113623695589465,
-0.748924457612014));
#84147=CARTESIAN_POINT('Ctrl Pts',(-0.151858149074166,0.123570863371261,
-0.749619557979654));
#84148=CARTESIAN_POINT('Ctrl Pts',(-0.143814658298944,0.13284331254129,
-0.750314658347294));
#84149=CARTESIAN_POINT('Ctrl Pts',(-0.134994156289213,0.141271857663738,
-0.751009758714934));
#84150=CARTESIAN_POINT('Ctrl Pts',(-0.126153503139833,0.149719658469096,
-0.751706447094748));
#84151=CARTESIAN_POINT('Ctrl Pts',(-0.11653297221146,0.157319149566077,
-0.752403135474563));
#84152=CARTESIAN_POINT('Ctrl Pts',(-0.106323038009839,0.163940756337033,
-0.753099823854378));
#84153=CARTESIAN_POINT('Ctrl Pts',(-0.103157589582081,0.165993693635985,
-0.7533158224194));
#84154=CARTESIAN_POINT('Ctrl Pts',(-0.0999356808215271,0.167952959412892,
-0.753531820984422));
#84155=CARTESIAN_POINT('Ctrl Pts',(-0.0966634547837876,0.169815595600824,
-0.753747819549444));
#84156=CARTESIAN_POINT('Ctrl Pts',(-0.0861091517251182,0.17582337947295,
-0.75444450562467));
#84157=CARTESIAN_POINT('Ctrl Pts',(-0.0749555780612429,0.180864537255721,
-0.755141191699895));
#84158=CARTESIAN_POINT('Ctrl Pts',(-0.0634033071758778,0.184827434757834,
-0.75583787777512));
#84159=CARTESIAN_POINT('Ctrl Pts',(-0.0518751400605106,0.188782063689129,
-0.756533110217455));
#84160=CARTESIAN_POINT('Ctrl Pts',(-0.0399507223910989,0.19166254699148,
-0.75722834265979));
#84161=CARTESIAN_POINT('Ctrl Pts',(-0.0278512904924889,0.193404926560579,
-0.757923575102125));
#84162=CARTESIAN_POINT('Ctrl Pts',(-0.0157535295004372,0.195147065510658,
-0.758618711534295));
#84163=CARTESIAN_POINT('Ctrl Pts',(-0.00348166052095019,0.195751243336099,
-0.759313847966465));
#84164=CARTESIAN_POINT('Ctrl Pts',(0.0087335981420215,0.195204723978427,
-0.760008984398636));
#84165=CARTESIAN_POINT('Ctrl Pts',(0.0209482231105826,0.194658232972693,
-0.760704084769018));
#84166=CARTESIAN_POINT('Ctrl Pts',(0.0331053707006321,0.192961229423343,
-0.7613991851394));
#84167=CARTESIAN_POINT('Ctrl Pts',(0.0449778324117177,0.190152976814836,
-0.762094285509782));
#84168=CARTESIAN_POINT('Ctrl Pts',(0.0568774177024041,0.187338308530707,
-0.762790973892043));
#84169=CARTESIAN_POINT('Ctrl Pts',(0.0684901829337995,0.183407587835583,
-0.763487662274304));
#84170=CARTESIAN_POINT('Ctrl Pts',(0.0796037273880817,0.178450011448372,
-0.764184350656565));
#84171=CARTESIAN_POINT('Ctrl Pts',(0.0830493273897015,0.176912983790087,
-0.764400349206885));
#84172=CARTESIAN_POINT('Ctrl Pts',(0.0864471078133341,0.175277592480136,
-0.764616347757206));
#84173=CARTESIAN_POINT('Ctrl Pts',(0.0897912424479248,0.173547379063062,
-0.764832346307526));
#84174=CARTESIAN_POINT('Ctrl Pts',(0.100577482201028,0.167966713575625,
-0.765529032417583));
#84175=CARTESIAN_POINT('Ctrl Pts',(0.110879316957741,0.161357046962324,
-0.766225718527639));
#84176=CARTESIAN_POINT('Ctrl Pts',(0.120493893810033,0.153825815630851,
-0.766922404637696));
#84177=CARTESIAN_POINT('Ctrl Pts',(0.130088409888116,0.14631029818191,-0.767617637115111));
#84178=CARTESIAN_POINT('Ctrl Pts',(0.138997786808178,0.137877508735213,
-0.768312869592525));
#84179=CARTESIAN_POINT('Ctrl Pts',(0.147047906989292,0.128678176277365,
-0.76900810206994));
#84180=CARTESIAN_POINT('Ctrl Pts',(0.155096915463461,0.119480114230585,
-0.769703238537015));
#84181=CARTESIAN_POINT('Ctrl Pts',(0.162286293315973,0.109516346921563,
-0.77039837500409));
#84182=CARTESIAN_POINT('Ctrl Pts',(0.168479720973745,0.0989734490689751,
-0.771093511471166));
#84183=CARTESIAN_POINT('Ctrl Pts',(0.174672827332737,0.0884310981542712,
-0.771788611876384));
#84184=CARTESIAN_POINT('Ctrl Pts',(0.179869666201818,0.0773104444712772,
-0.772483712281603));
#84185=CARTESIAN_POINT('Ctrl Pts',(0.183979442788537,0.065823435273613,
-0.773178812686822));
#84186=CARTESIAN_POINT('Ctrl Pts',(0.188098608480714,0.0543101831066573,
-0.773875501103182));
#84187=CARTESIAN_POINT('Ctrl Pts',(0.191125521016396,0.0424297497631005,
-0.774572189519542));
#84188=CARTESIAN_POINT('Ctrl Pts',(0.19301932961613,0.0304088538840238,
-0.775268877935902));
#84189=CARTESIAN_POINT('Ctrl Pts',(0.193606478151208,0.0266819453639537,
-0.77548487631247));
#84190=CARTESIAN_POINT('Ctrl Pts',(0.194085086310145,0.0229415806826977,
-0.775700874689037));
#84191=CARTESIAN_POINT('Ctrl Pts',(0.194454951830309,0.0191945749802449,
-0.775916873065605));
#84192=CARTESIAN_POINT('Ctrl Pts',(0.195647924404063,0.00710889844909368,
-0.776613559091126));
#84193=CARTESIAN_POINT('Ctrl Pts',(0.195714061909135,-0.00513083536851569,
-0.777310245116648));
#84194=CARTESIAN_POINT('Ctrl Pts',(0.194633010957284,-0.0172959835135673,
-0.778006931142169));
#84195=CARTESIAN_POINT('Ctrl Pts',(0.193554215613781,-0.0294357491272439,
-0.778702163535175));
#84196=CARTESIAN_POINT('Ctrl Pts',(0.191332986002734,-0.0415003685242515,
-0.779397395928181));
#84197=CARTESIAN_POINT('Ctrl Pts',(0.188000927272401,-0.053261724950639,
-0.780092628321187));
#84198=CARTESIAN_POINT('Ctrl Pts',(0.184669328686416,-0.0650214571794575,
-0.780787764705304));
#84199=CARTESIAN_POINT('Ctrl Pts',(0.180227400023203,-0.0764771566544016,
-0.781482901089421));
#84200=CARTESIAN_POINT('Ctrl Pts',(0.17475739415817,-0.0874128891356764,
-0.782178037473538));
#84201=CARTESIAN_POINT('Ctrl Pts',(0.169287672056742,-0.0983480543117332,
-0.782873137796559));
#84202=CARTESIAN_POINT('Ctrl Pts',(0.162790394247606,-0.108762535603792,
-0.78356823811958));
#84203=CARTESIAN_POINT('Ctrl Pts',(0.155393884766881,-0.118464765128949,
-0.784263338442601));
#84204=CARTESIAN_POINT('Ctrl Pts',(0.147980477353117,-0.128189160193849,
-0.784960026779367));
#84205=CARTESIAN_POINT('Ctrl Pts',(0.139664319068716,-0.13719739936423,
-0.785656715116132));
#84206=CARTESIAN_POINT('Ctrl Pts',(0.13061332010973,-0.1453317604996,-0.786353403452897));
#84207=CARTESIAN_POINT('Ctrl Pts',(0.127807180373147,-0.147853709084183,
-0.78656940224316));
#84208=CARTESIAN_POINT('Ctrl Pts',(0.124930648719368,-0.150291948941695,
-0.786785401033423));
#84209=CARTESIAN_POINT('Ctrl Pts',(0.121989331094927,-0.152642599227779,
-0.787001399823686));
#84210=CARTESIAN_POINT('Ctrl Pts',(0.112502356527963,-0.160224425581584,
-0.787698085898216));
#84211=CARTESIAN_POINT('Ctrl Pts',(0.102272552464107,-0.166945034456582,
-0.788394771972746));
#84212=CARTESIAN_POINT('Ctrl Pts',(0.0914806049602737,-0.172662847526914,
-0.789091458047276));
#84213=CARTESIAN_POINT('Ctrl Pts',(0.0807111748267906,-0.178368730395172,
-0.789786690488127));
#84214=CARTESIAN_POINT('Ctrl Pts',(0.06938266028967,-0.183075499694555,
-0.790481922928977));
#84215=CARTESIAN_POINT('Ctrl Pts',(0.0577036000417347,-0.18668544276998,
-0.791177155369828));
#84216=CARTESIAN_POINT('Ctrl Pts',(0.0460261526663467,-0.19029488731402,
-0.791872291799416));
#84217=CARTESIAN_POINT('Ctrl Pts',(0.0339990769748144,-0.192807505017742,
-0.792567428229004));
#84218=CARTESIAN_POINT('Ctrl Pts',(0.0218482740129643,-0.194174696916602,
-0.793262564658592));
#84219=CARTESIAN_POINT('Ctrl Pts',(0.00969810141288971,-0.195541817888009,
-0.793957665025755));
#84220=CARTESIAN_POINT('Ctrl Pts',(-0.00257491320132761,-0.195763560068986,
-0.794652765392917));
#84221=CARTESIAN_POINT('Ctrl Pts',(-0.0147402175345476,-0.19484323438866,
-0.795347865760079));
#84222=CARTESIAN_POINT('Ctrl Pts',(-0.0269333144546391,-0.193920806152515,
-0.796044554138261));
#84223=CARTESIAN_POINT('Ctrl Pts',(-0.0390173429669599,-0.191851232420075,
-0.796741242516443));
#84224=CARTESIAN_POINT('Ctrl Pts',(-0.0507685815630807,-0.188689456849271,
-0.797437930894624));
#84225=CARTESIAN_POINT('Ctrl Pts',(-0.0544118899954307,-0.18770919221554,
-0.797653929457005));
#84226=CARTESIAN_POINT('Ctrl Pts',(-0.058023321427186,-0.186624304545733,
-0.797869928019385));
#84227=CARTESIAN_POINT('Ctrl Pts',(-0.0615965681883146,-0.185437382389372,
-0.798085926581765));
#84228=CARTESIAN_POINT('Ctrl Pts',(-0.073121793005532,-0.181609058848606,
-0.798782612861233));
#84229=CARTESIAN_POINT('Ctrl Pts',(-0.0843291966479146,-0.176688726846239,
-0.7994792991407));
#84230=CARTESIAN_POINT('Ctrl Pts',(-0.0950016407521072,-0.17075083676049,
-0.800175985420167));
#84231=CARTESIAN_POINT('Ctrl Pts',(-0.105651816866004,-0.164825336046615,
-0.800871218067911));
#84232=CARTESIAN_POINT('Ctrl Pts',(-0.115768456042509,-0.157886848105303,
-0.801566450715655));
#84233=CARTESIAN_POINT('Ctrl Pts',(-0.125156044212862,-0.150057071132913,
-0.8022616833634));
#84234=CARTESIAN_POINT('Ctrl Pts',(-0.13454233595766,-0.142228375452412,
-0.802956819999543));
#84235=CARTESIAN_POINT('Ctrl Pts',(-0.143199076614239,-0.133509159851367,
-0.803651956635686));
#84236=CARTESIAN_POINT('Ctrl Pts',(-0.150962490541431,-0.124062429645434,
-0.80434709327183));
#84237=CARTESIAN_POINT('Ctrl Pts',(-0.158725501716818,-0.114616189518696,
-0.805042193845547));
#84238=CARTESIAN_POINT('Ctrl Pts',(-0.165594743530101,-0.104443202878264,
-0.805737294419265));
#84239=CARTESIAN_POINT('Ctrl Pts',(-0.171447445837107,-0.093738643663818,
-0.806432394992983));
#84240=CARTESIAN_POINT('Ctrl Pts',(-0.177313519063283,-0.0830096291142981,
-0.807129083573933));
#84241=CARTESIAN_POINT('Ctrl Pts',(-0.182158054466896,-0.0717474160740974,
-0.807825772154882));
#84242=CARTESIAN_POINT('Ctrl Pts',(-0.185905307464628,-0.0601695658658265,
-0.808522460735831));
#84243=CARTESIAN_POINT('Ctrl Pts',(-0.187067085382959,-0.0565800322202864,
-0.808738458270502));
#84244=CARTESIAN_POINT('Ctrl Pts',(-0.188123755338865,-0.0529602626463094,
-0.808954455805174));
#84245=CARTESIAN_POINT('Ctrl Pts',(-0.189074053603399,-0.0493169570632572,
-0.809170453339845));
#84246=CARTESIAN_POINT('Ctrl Pts',(-0.192997021238052,-0.03427686868377,
-0.810062122165628));
#84247=CARTESIAN_POINT('Ctrl Pts',(-0.195125884706412,-0.0187503439611592,
-0.810953790991411));
#84248=CARTESIAN_POINT('Ctrl Pts',(-0.195375169370054,-0.00311499496350872,
-0.811845459817194));
#84249=CARTESIAN_POINT('Ctrl Pts',(-0.195390785359249,-0.00213554665955173,
-0.81190131680633));
#84250=CARTESIAN_POINT('Ctrl Pts',(-0.195399040891236,-0.00115567898833329,
-0.811957173795467));
#84251=CARTESIAN_POINT('Ctrl Pts',(-0.195399921197426,-0.00017548800484569,
-0.812013030784603));
#84252=CARTESIAN_POINT('',(-0.195379220633989,7.37186862735708E-5,-0.882013034935241));
#84253=CARTESIAN_POINT('Ctrl Pts',(-0.195399921197473,-0.000175487952656256,
-0.812013030787577));
#84254=CARTESIAN_POINT('Ctrl Pts',(-0.19541076648611,0.0119003754503791,
-0.812701183792726));
#84255=CARTESIAN_POINT('Ctrl Pts',(-0.19429783114136,0.0240036113255929,
-0.813389336797875));
#84256=CARTESIAN_POINT('Ctrl Pts',(-0.192072370349911,0.0359077226814327,
-0.814077489803025));
#84257=CARTESIAN_POINT('Ctrl Pts',(-0.18984883478061,0.0478015359188242,
-0.814765047494425));
#84258=CARTESIAN_POINT('Ctrl Pts',(-0.186514832957703,0.059495682482877,
-0.815452605185825));
#84259=CARTESIAN_POINT('Ctrl Pts',(-0.182133079421123,0.070772179425102,
-0.816140162877225));
#84260=CARTESIAN_POINT('Ctrl Pts',(-0.177740715773814,0.0820759816185671,
-0.816829385441645));
#84261=CARTESIAN_POINT('Ctrl Pts',(-0.172295871312637,0.0929592772620382,
-0.817518608006064));
#84262=CARTESIAN_POINT('Ctrl Pts',(-0.16590985247905,0.103223451067962,
-0.818207830570483));
#84263=CARTESIAN_POINT('Ctrl Pts',(-0.159587204270127,0.113385770005823,
-0.818890213746297));
#84264=CARTESIAN_POINT('Ctrl Pts',(-0.152342595762826,0.122940581824888,
-0.819572596922112));
#84265=CARTESIAN_POINT('Ctrl Pts',(-0.144323676122428,0.131726369837283,
-0.820254980097926));
#84266=CARTESIAN_POINT('Ctrl Pts',(-0.136136676912347,0.140696311268674,
-0.820951666281588));
#84267=CARTESIAN_POINT('Ctrl Pts',(-0.127081505453031,0.14893156321025,
-0.821648352465251));
#84268=CARTESIAN_POINT('Ctrl Pts',(-0.117314529548643,0.156264075067754,
-0.822345038648913));
#84269=CARTESIAN_POINT('Ctrl Pts',(-0.107567932485336,0.16358128760484,
-0.823040271193582));
#84270=CARTESIAN_POINT('Ctrl Pts',(-0.0971131273755955,0.169998919590237,
-0.823735503738251));
#84271=CARTESIAN_POINT('Ctrl Pts',(-0.0861408413320165,0.175387899966367,
-0.82443073628292));
#84272=CARTESIAN_POINT('Ctrl Pts',(-0.0751700706993675,0.180776136056418,
-0.825125872807216));
#84273=CARTESIAN_POINT('Ctrl Pts',(-0.0636827251959411,0.185135576734265,
-0.825821009331513));
#84274=CARTESIAN_POINT('Ctrl Pts',(-0.0518943488922855,0.188382951864137,
-0.826516145855809));
#84275=CARTESIAN_POINT('Ctrl Pts',(-0.0401065842361512,0.191630158501852,
-0.827211246312497));
#84276=CARTESIAN_POINT('Ctrl Pts',(-0.0280186705253376,0.193765207842195,
-0.827906346769186));
#84277=CARTESIAN_POINT('Ctrl Pts',(-0.0158588500843532,0.194755377009216,
-0.828601447225874));
#84278=CARTESIAN_POINT('Ctrl Pts',(-0.0036712497476722,0.195747808281696,
-0.829298135684481));
#84279=CARTESIAN_POINT('Ctrl Pts',(0.00858770854901134,0.195590132007127,
-0.829994824143088));
#84280=CARTESIAN_POINT('Ctrl Pts',(0.0206884687465203,0.194301691348594,
-0.830691512601694));
#84281=CARTESIAN_POINT('Ctrl Pts',(0.0244401327717179,0.193902229133962,
-0.830907510686465));
#84282=CARTESIAN_POINT('Ctrl Pts',(0.0281766441647945,0.193394450641261,
-0.831123508771235));
#84283=CARTESIAN_POINT('Ctrl Pts',(0.0318913685240223,0.192779927932513,
-0.831339506856005));
#84284=CARTESIAN_POINT('Ctrl Pts',(0.0438729625033843,0.190797826200248,
-0.8320361941743));
#84285=CARTESIAN_POINT('Ctrl Pts',(0.0557111120044502,0.18768748499762,
-0.832732881492595));
#84286=CARTESIAN_POINT('Ctrl Pts',(0.0671797176113246,0.18348854335261,
-0.83342956881089));
#84287=CARTESIAN_POINT('Ctrl Pts',(0.0786243942018095,0.179298362715423,
-0.83412480250502));
#84288=CARTESIAN_POINT('Ctrl Pts',(0.0897002184680624,0.174024318521112,
-0.834820036199149));
#84289=CARTESIAN_POINT('Ctrl Pts',(0.100195074047842,0.167756094186016,
-0.835515269893279));
#84290=CARTESIAN_POINT('Ctrl Pts',(0.110688480214663,0.161488735536542,
-0.836210407570773));
#84291=CARTESIAN_POINT('Ctrl Pts',(0.120600303685354,0.154227878369273,
-0.836905545248266));
#84292=CARTESIAN_POINT('Ctrl Pts',(0.129743328677118,0.146108961613521,
-0.83760068292576));
#84293=CARTESIAN_POINT('Ctrl Pts',(0.138885879320792,0.137990466074233,
-0.838295784538906));
#84294=CARTESIAN_POINT('Ctrl Pts',(0.147259074374735,0.129014600520134,
-0.838990886152053));
#84295=CARTESIAN_POINT('Ctrl Pts',(0.154711178707542,0.119354979715649,
-0.839685987765199));
#84296=CARTESIAN_POINT('Ctrl Pts',(0.162180307648888,0.10967329114943,-0.840382677363742));
#84297=CARTESIAN_POINT('Ctrl Pts',(0.168723662724559,0.0993054610685011,
-0.841079366962286));
#84298=CARTESIAN_POINT('Ctrl Pts',(0.174232462703801,0.0884545586172281,
-0.841776056560829));
#84299=CARTESIAN_POINT('Ctrl Pts',(0.175940337576147,0.0850904895443564,
-0.841992048911915));
#84300=CARTESIAN_POINT('Ctrl Pts',(0.177549118335746,0.0816801484068674,
-0.842208041263));
#84301=CARTESIAN_POINT('Ctrl Pts',(0.179056510935435,0.078229955206612,
-0.842424033614086));
#84302=CARTESIAN_POINT('Ctrl Pts',(0.183918604355241,0.067101360267584,
-0.843120716740406));
#84303=CARTESIAN_POINT('Ctrl Pts',(0.18775631155332,0.055478697225224,-0.843817399866725));
#84304=CARTESIAN_POINT('Ctrl Pts',(0.190479756283891,0.0435731849424565,
-0.844514082993045));
#84305=CARTESIAN_POINT('Ctrl Pts',(0.193197518552431,0.0316925134874612,
-0.845209312491403));
#84306=CARTESIAN_POINT('Ctrl Pts',(0.194805367887041,0.0195309922381451,
-0.84590454198976));
#84307=CARTESIAN_POINT('Ctrl Pts',(0.195263016082719,0.00731536398820651,
-0.846599771488118));
#84308=CARTESIAN_POINT('Ctrl Pts',(0.195720601111664,-0.00489857820389136,
-0.847294905027666));
#84309=CARTESIAN_POINT('Ctrl Pts',(0.195028222143748,-0.01716574122849,
-0.847990038567214));
#84310=CARTESIAN_POINT('Ctrl Pts',(0.19319752702589,-0.0292553508110982,
-0.848685172106763));
#84311=CARTESIAN_POINT('Ctrl Pts',(0.191366926808907,-0.0413443336839361,
-0.849380269611484));
#84312=CARTESIAN_POINT('Ctrl Pts',(0.188398285339225,-0.0532549203161764,
-0.850075367116206));
#84313=CARTESIAN_POINT('Ctrl Pts',(0.184354590604969,-0.0647653064755681,
-0.850770464620928));
#84314=CARTESIAN_POINT('Ctrl Pts',(0.180301657159965,-0.0763019906458915,
-0.851467150228909));
#84315=CARTESIAN_POINT('Ctrl Pts',(0.175169118484121,-0.0874358457666871,
-0.852163835836891));
#84316=CARTESIAN_POINT('Ctrl Pts',(0.169068057282984,-0.0979650550275846,
-0.852860521444872));
#84317=CARTESIAN_POINT('Ctrl Pts',(0.167176374190521,-0.101229721038824,
-0.853076534420637));
#84318=CARTESIAN_POINT('Ctrl Pts',(0.165191901970452,-0.104436460480499,
-0.853292547396402));
#84319=CARTESIAN_POINT('Ctrl Pts',(0.163118777296953,-0.107579851706289,
-0.853508560372167));
#84320=CARTESIAN_POINT('Ctrl Pts',(0.156432510105898,-0.117717955743309,
-0.854205248078005));
#84321=CARTESIAN_POINT('Ctrl Pts',(0.148774015022097,-0.127265912653565,
-0.854901935783844));
#84322=CARTESIAN_POINT('Ctrl Pts',(0.140271507458899,-0.136033320165348,
-0.855598623489683));
#84323=CARTESIAN_POINT('Ctrl Pts',(0.13178674080447,-0.144782434041324,
-0.856293857521656));
#84324=CARTESIAN_POINT('Ctrl Pts',(0.122462007313727,-0.152753557937461,
-0.85698909155363));
#84325=CARTESIAN_POINT('Ctrl Pts',(0.112465545786131,-0.159789427093997,
-0.857684325585604));
#84326=CARTESIAN_POINT('Ctrl Pts',(0.102470465927083,-0.166824323782515,
-0.858379463525276));
#84327=CARTESIAN_POINT('Ctrl Pts',(0.0918045306694918,-0.17292368243484,
-0.859074601464948));
#84328=CARTESIAN_POINT('Ctrl Pts',(0.0806676418023429,-0.177971603257511,
-0.859769739404621));
#84329=CARTESIAN_POINT('Ctrl Pts',(0.0695313314239663,-0.183019261873604,
-0.860464841236409));
#84330=CARTESIAN_POINT('Ctrl Pts',(0.0579249240961688,-0.187015254500705,
-0.861159943068197));
#84331=CARTESIAN_POINT('Ctrl Pts',(0.0460687555565446,-0.18989162635954,
-0.861855044899985));
#84332=CARTESIAN_POINT('Ctrl Pts',(0.034185502306362,-0.192774569118494,
-0.862551734650489));
#84333=CARTESIAN_POINT('Ctrl Pts',(0.0220522138573652,-0.194532642413946,
-0.863248424400992));
#84334=CARTESIAN_POINT('Ctrl Pts',(0.00989865210069558,-0.195149113978489,
-0.863945114151496));
#84335=CARTESIAN_POINT('Ctrl Pts',(0.00613074842564256,-0.195340235356742,
-0.864161105144413));
#84336=CARTESIAN_POINT('Ctrl Pts',(0.00236090170122731,-0.195422010120875,
-0.864377096137329));
#84337=CARTESIAN_POINT('Ctrl Pts',(-0.00140409027209528,-0.195394955233004,
-0.864593087130246));
#84338=CARTESIAN_POINT('Ctrl Pts',(-0.0135483239942191,-0.195307687880524,
-0.865289780541132));
#84339=CARTESIAN_POINT('Ctrl Pts',(-0.0257270041931643,-0.194083600023529,
-0.865986473952018));
#84340=CARTESIAN_POINT('Ctrl Pts',(-0.0377106119642735,-0.191726549401172,
-0.866683167362904));
#84341=CARTESIAN_POINT('Ctrl Pts',(-0.0496692174156106,-0.189374416474262,
-0.867378407208905));
#84342=CARTESIAN_POINT('Ctrl Pts',(-0.0614326940351443,-0.185894107403963,
-0.868073647054907));
#84343=CARTESIAN_POINT('Ctrl Pts',(-0.0727775223520668,-0.181341093633777,
-0.868768886900908));
#84344=CARTESIAN_POINT('Ctrl Pts',(-0.0841207837437583,-0.176788708716841,
-0.869464030721759));
#84345=CARTESIAN_POINT('Ctrl Pts',(-0.0950446839703465,-0.17116419653728,
-0.870159174542609));
#84346=CARTESIAN_POINT('Ctrl Pts',(-0.105343155999477,-0.16457211028625,
-0.870854318363459));
#84347=CARTESIAN_POINT('Ctrl Pts',(-0.115641093753242,-0.157980366026662,
-0.87154942612088));
#84348=CARTESIAN_POINT('Ctrl Pts',(-0.125312945390698,-0.150421641829479,
-0.872244533878301));
#84349=CARTESIAN_POINT('Ctrl Pts',(-0.134181729704214,-0.142043737678171,
-0.872939641635722));
#84350=CARTESIAN_POINT('Ctrl Pts',(-0.143070773483751,-0.133646695406184,
-0.873636337267139));
#84351=CARTESIAN_POINT('Ctrl Pts',(-0.151152496979953,-0.124427385289625,
-0.874333032898556));
#84352=CARTESIAN_POINT('Ctrl Pts',(-0.158287747857834,-0.114569406379255,
-0.875029728529974));
#84353=CARTESIAN_POINT('Ctrl Pts',(-0.160499533685813,-0.111513629025431,
-0.875245690316091));
#84354=CARTESIAN_POINT('Ctrl Pts',(-0.162620689753645,-0.10839669430786,
-0.875461652102209));
#84355=CARTESIAN_POINT('Ctrl Pts',(-0.164647949236151,-0.105224582737732,
-0.875677613888326));
#84356=CARTESIAN_POINT('Ctrl Pts',(-0.171337062502713,-0.0947579336630299,
-0.876390197975886));
#84357=CARTESIAN_POINT('Ctrl Pts',(-0.177045708979376,-0.0836179136310407,
-0.877102782063446));
#84358=CARTESIAN_POINT('Ctrl Pts',(-0.181648137368076,-0.0720077370197724,
-0.877815366151006));
#84359=CARTESIAN_POINT('Ctrl Pts',(-0.186238975491459,-0.060426798240347,
-0.878526155742718));
#84360=CARTESIAN_POINT('Ctrl Pts',(-0.189728752788956,-0.0483787787415931,
-0.87923694533443));
#84361=CARTESIAN_POINT('Ctrl Pts',(-0.19203819111273,-0.0360900700214141,
-0.879947734926141));
#84362=CARTESIAN_POINT('Ctrl Pts',(-0.194274986862109,-0.024187898334174,
-0.880636166879953));
#84363=CARTESIAN_POINT('Ctrl Pts',(-0.195404560012147,-0.0120607127809722,
-0.881324598833765));
#84364=CARTESIAN_POINT('Ctrl Pts',(-0.195399986118627,7.3653515014446E-5,
-0.882013030787577));
#84365=CARTESIAN_POINT('Ctrl Pts',(-0.195109753188566,7.45643940919532E-5,
-0.882013088758234));
#84366=CARTESIAN_POINT('Ctrl Pts',(-0.195204102274039,0.0279355699642562,
-0.883596106054292));
#84367=CARTESIAN_POINT('Ctrl Pts',(-0.176621603793911,0.120705073777376,
-0.888873965603043));
#84368=CARTESIAN_POINT('Ctrl Pts',(-0.03438531833784,0.228170121929786,
-0.897846667404486));
#84369=CARTESIAN_POINT('Ctrl Pts',(0.172650552859722,0.153093766216358,
-0.908931194162567));
#84370=CARTESIAN_POINT('Ctrl Pts',(0.222416746898179,-0.0614474453631151,
-0.920015720920646));
#84371=CARTESIAN_POINT('Ctrl Pts',(0.0695869939549012,-0.219994184582197,
-0.931100247678726));
#84372=CARTESIAN_POINT('Ctrl Pts',(-0.138468335956508,-0.179768882909404,
-0.94176601763437));
#84373=CARTESIAN_POINT('Ctrl Pts',(-0.195199225693986,-0.0571389522596028,
-0.94873694533732));
#84374=CARTESIAN_POINT('Ctrl Pts',(-0.1956163961968,0.000134331411914747,
-0.952013030787577));
#84375=CARTESIAN_POINT('Origin',(0.,0.,-1.10400562256037));
#84376=CARTESIAN_POINT('',(-0.155549940342626,0.000136232908569803,-0.0190056209657492));
#84377=CARTESIAN_POINT('Ctrl Pts',(0.102472688294207,0.117287771082297,
-0.0445113451759945));
#84378=CARTESIAN_POINT('Ctrl Pts',(0.0989611449419164,0.120398369956428,
-0.0441741475577544));
#84379=CARTESIAN_POINT('Ctrl Pts',(0.055236448550028,0.15556450473979,-0.0401421076868207));
#84380=CARTESIAN_POINT('Ctrl Pts',(-0.065934354559954,0.171464947984463,
-0.0324152255631935));
#84381=CARTESIAN_POINT('Ctrl Pts',(-0.149738893304472,0.0731738720390481,
-0.0242505156428922));
#84382=CARTESIAN_POINT('Ctrl Pts',(-0.155685419418353,0.0109444862887444,
-0.0197806479752842));
#84383=CARTESIAN_POINT('Ctrl Pts',(-0.155585995199752,0.000136286723707784,
-0.0190056225603694));
#84384=CARTESIAN_POINT('',(0.0210111597547384,-0.154124409701257,-3.03070625262691E-7));
#84385=CARTESIAN_POINT('Ctrl Pts',(-0.155549940342626,0.000136232908569803,
-0.0190056209657492));
#84386=CARTESIAN_POINT('Ctrl Pts',(-0.155558853686153,-0.0100409707379475,
-0.0182756668891895));
#84387=CARTESIAN_POINT('Ctrl Pts',(-0.154564581067856,-0.0202492057705681,
-0.01754571281263));
#84388=CARTESIAN_POINT('Ctrl Pts',(-0.152575659837309,-0.0302732641981308,
-0.0168157587360704));
#84389=CARTESIAN_POINT('Ctrl Pts',(-0.150595804610828,-0.0402516304418793,
-0.0160891319740994));
#84390=CARTESIAN_POINT('Ctrl Pts',(-0.147630507612318,-0.0500465508032369,
-0.0153625052121281));
#84391=CARTESIAN_POINT('Ctrl Pts',(-0.143739789739225,-0.0594531357097622,
-0.014635878450157));
#84392=CARTESIAN_POINT('Ctrl Pts',(-0.13982234774238,-0.0689243315049017,
-0.0139042607163031));
#84393=CARTESIAN_POINT('Ctrl Pts',(-0.134967074703252,-0.0780009252912488,
-0.0131726429824491));
#84394=CARTESIAN_POINT('Ctrl Pts',(-0.129283997512143,-0.0864953784157288,
-0.0124410252485951));
#84395=CARTESIAN_POINT('Ctrl Pts',(-0.123600920321035,-0.0949898315402083,
-0.0117094075147413));
#84396=CARTESIAN_POINT('Ctrl Pts',(-0.117090687318054,-0.102901409291159,
-0.0109777897808876));
#84397=CARTESIAN_POINT('Ctrl Pts',(-0.109904308625208,-0.110076543575891,
-0.0102461720470337));
#84398=CARTESIAN_POINT('Ctrl Pts',(-0.102729446060097,-0.117240179751983,
-0.0095157267261066));
#84399=CARTESIAN_POINT('Ctrl Pts',(-0.0948223501874392,-0.123727993173485,
-0.00878528140517938));
#84400=CARTESIAN_POINT('Ctrl Pts',(-0.0863355949095739,-0.129390755278768,
-0.00805483608425228));
#84401=CARTESIAN_POINT('Ctrl Pts',(-0.0778602724806752,-0.135045888849732,
-0.00732537477556061));
#84402=CARTESIAN_POINT('Ctrl Pts',(-0.068807567315153,-0.139877575646078,
-0.00659591346686866));
#84403=CARTESIAN_POINT('Ctrl Pts',(-0.0593625781028027,-0.143777212453812,
-0.00586645215817705));
#84404=CARTESIAN_POINT('Ctrl Pts',(-0.0499260002920378,-0.147673376371267,
-0.00513764048410867));
#84405=CARTESIAN_POINT('Ctrl Pts',(-0.0400987007419705,-0.150638763861192,
-0.00440882881004057));
#84406=CARTESIAN_POINT('Ctrl Pts',(-0.0300864858397496,-0.152612600625946,
-0.0036800171359721));
#84407=CARTESIAN_POINT('Ctrl Pts',(-0.0200527190266847,-0.154590686196223,
-0.00294963664977016));
#84408=CARTESIAN_POINT('Ctrl Pts',(-0.00983418001629753,-0.155572803316964,
-0.00221925616356821));
#84409=CARTESIAN_POINT('Ctrl Pts',(0.000354303184596075,-0.15554959649338,
-0.00148887567736633));
#84410=CARTESIAN_POINT('Ctrl Pts',(0.00727594529835836,-0.155533830718998,
-0.000992684808452523));
#84411=CARTESIAN_POINT('Ctrl Pts',(0.0141835652280306,-0.155055188152375,
-0.000496493939539067));
#84412=CARTESIAN_POINT('Ctrl Pts',(0.0210111597547384,-0.154124409701257,
-3.03070625262691E-7));
#84413=CARTESIAN_POINT('',(-0.138946909435068,-0.0699253806456778,0.));
#84414=CARTESIAN_POINT('Origin',(0.,0.,0.));
#84415=CARTESIAN_POINT('',(-0.155549948455572,0.000126631232131687,-0.00519437743962925));
#84416=CARTESIAN_POINT('Ctrl Pts',(-0.155549936615206,0.000140424376441733,
-0.0050017268448989));
#84417=CARTESIAN_POINT('Ctrl Pts',(-0.155550517862743,-0.000503431197937891,
-0.00495542424155714));
#84418=CARTESIAN_POINT('Ctrl Pts',(-0.155547101522606,-0.0011472927388459,
-0.0049092353714434));
#84419=CARTESIAN_POINT('Ctrl Pts',(-0.155531454351363,-0.00250608036372759,
-0.00481199043401684));
#84420=CARTESIAN_POINT('Ctrl Pts',(-0.155518291643096,-0.00322098180988224,
-0.00476096163639329));
#84421=CARTESIAN_POINT('Ctrl Pts',(-0.155465720677275,-0.0052980293137128,
-0.00461307543001361));
#84422=CARTESIAN_POINT('Ctrl Pts',(-0.155413341233105,-0.0066598027843363,
-0.00451658109682896));
#84423=CARTESIAN_POINT('Ctrl Pts',(-0.155226329145725,-0.0102817887289338,
-0.00426101493953919));
#84424=CARTESIAN_POINT('Ctrl Pts',(-0.15506023115533,-0.0125400927092421,
-0.00410279931249361));
#84425=CARTESIAN_POINT('Ctrl Pts',(-0.154165829117664,-0.0219015287112345,
-0.00345034722190772));
#84426=CARTESIAN_POINT('Ctrl Pts',(-0.152998200286724,-0.028954161007669,
-0.00296738723038534));
#84427=CARTESIAN_POINT('Ctrl Pts',(-0.149139281806736,-0.0452219429515892,
-0.00184186572284642));
#84428=CARTESIAN_POINT('Ctrl Pts',(-0.146072590171909,-0.0543167899376314,
-0.00120369172680408));
#84429=CARTESIAN_POINT('Ctrl Pts',(-0.141566225103923,-0.0644761159143157,
-0.00042849118234209));
#84430=CARTESIAN_POINT('Ctrl Pts',(-0.140922145946666,-0.0658719518483347,
-0.000320527592429761));
#84431=CARTESIAN_POINT('Ctrl Pts',(-0.140029455127714,-0.067733539564464,
-0.000174304757339283));
#84432=CARTESIAN_POINT('Ctrl Pts',(-0.139798985468618,-0.0682079491771672,
-0.000136843834668115));
#84433=CARTESIAN_POINT('Ctrl Pts',(-0.139361561421611,-0.06909683287829,
-6.62681200140033E-5));
#84434=CARTESIAN_POINT('Ctrl Pts',(-0.139155158822226,-0.0695115736921777,
-3.31792881770164E-5));
#84435=CARTESIAN_POINT('Ctrl Pts',(-0.138946909435068,-0.0699253806456779,
1.65503461629912E-16));
#84436=CARTESIAN_POINT('Ctrl Pts',(0.10234224283772,0.117140376604078,-0.0306875317892119));
#84437=CARTESIAN_POINT('Ctrl Pts',(0.094583506915784,0.123918965326908,
-0.0299499611150766));
#84438=CARTESIAN_POINT('Ctrl Pts',(0.0861337948976529,0.12993622197685,
-0.0292123904409415));
#84439=CARTESIAN_POINT('Ctrl Pts',(0.0771670433343891,0.135059431077687,
-0.0284748197668061));
#84440=CARTESIAN_POINT('Ctrl Pts',(0.0682074047892692,0.140178576111506,
-0.0277378341823267));
#84441=CARTESIAN_POINT('Ctrl Pts',(0.0587323383981438,0.144404615767851,
-0.0270008485978476));
#84442=CARTESIAN_POINT('Ctrl Pts',(0.048942195600838,0.147649801861599,
-0.0262638630133682));
#84443=CARTESIAN_POINT('Ctrl Pts',(0.0391279920756871,0.150902963481447,
-0.0255250661775169));
#84444=CARTESIAN_POINT('Ctrl Pts',(0.0289980539335844,0.153170184543577,
-0.0247862693416651));
#84445=CARTESIAN_POINT('Ctrl Pts',(0.0187684845020169,0.154413556689487,
-0.0240474725058137));
#84446=CARTESIAN_POINT('Ctrl Pts',(0.0100987950178107,0.155467330310212,
-0.0234213328425959));
#84447=CARTESIAN_POINT('Ctrl Pts',(0.00135808684489701,0.155786583508046,
-0.0227951931793781));
#84448=CARTESIAN_POINT('Ctrl Pts',(-0.0073214427802927,0.155377601267412,
-0.0221690535161603));
#84449=CARTESIAN_POINT('Ctrl Pts',(-0.0174343336593535,0.154901078581321,
-0.0214395114369677));
#84450=CARTESIAN_POINT('Ctrl Pts',(-0.0275428404924019,0.15343092992204,
-0.0207099693577752));
#84451=CARTESIAN_POINT('Ctrl Pts',(-0.0374342961525748,0.150978395711311,
-0.0199804272785826));
#84452=CARTESIAN_POINT('Ctrl Pts',(-0.0474855104765481,0.148486250183311,
-0.0192391022352074));
#84453=CARTESIAN_POINT('Ctrl Pts',(-0.0573115842108452,0.144979686726725,
-0.0184977771918322));
#84454=CARTESIAN_POINT('Ctrl Pts',(-0.0666968112862147,0.140525221452418,
-0.017756452148457));
#84455=CARTESIAN_POINT('Ctrl Pts',(-0.075913181054113,0.136150900111379,
-0.0170284648911343));
#84456=CARTESIAN_POINT('Ctrl Pts',(-0.084703590970681,0.130863005220033,
-0.016300477633812));
#84457=CARTESIAN_POINT('Ctrl Pts',(-0.0928847001194851,0.124772733334304,
-0.0155724903764893));
#84458=CARTESIAN_POINT('Ctrl Pts',(-0.101290644007637,0.118515087481662,
-0.0148244964400879));
#84459=CARTESIAN_POINT('Ctrl Pts',(-0.109052378371382,0.111410830305483,
-0.0140765025036864));
#84460=CARTESIAN_POINT('Ctrl Pts',(-0.116007279635627,0.103624869464532,
-0.013328508567285));
#84461=CARTESIAN_POINT('Ctrl Pts',(-0.122962180899872,0.0958389086235821,
-0.0125805146308835));
#84462=CARTESIAN_POINT('Ctrl Pts',(-0.129109668280135,0.0873721506017285,
-0.011832520694482));
#84463=CARTESIAN_POINT('Ctrl Pts',(-0.13433441540455,0.0784223650364991,
-0.0110845267580806));
#84464=CARTESIAN_POINT('Ctrl Pts',(-0.139898640305477,0.0688910674417676,
-0.0102879319396981));
#84465=CARTESIAN_POINT('Ctrl Pts',(-0.144456639849757,0.058745004040905,
-0.00949133712131538));
#84466=CARTESIAN_POINT('Ctrl Pts',(-0.147892118257631,0.0482050190049829,
-0.00869474230293288));
#84467=CARTESIAN_POINT('Ctrl Pts',(-0.151308474758384,0.0377236996310117,
-0.00790258133926343));
#84468=CARTESIAN_POINT('Ctrl Pts',(-0.153614448655364,0.0268534505681371,
-0.00711042037559407));
#84469=CARTESIAN_POINT('Ctrl Pts',(-0.154742021800765,0.0158337989443936,
-0.00631825941192465));
#84470=CARTESIAN_POINT('Ctrl Pts',(-0.155275271644623,0.0106224053140157,
-0.00594363208782615));
#84471=CARTESIAN_POINT('Ctrl Pts',(-0.155545673493413,0.00537786453568078,
-0.00556900476372773));
#84472=CARTESIAN_POINT('Ctrl Pts',(-0.155549948455572,0.000126631232131687,
-0.00519437743962925));
#84473=CARTESIAN_POINT('Ctrl Pts',(-0.0684858909661362,0.139417771125461,
-0.997734010353788));
#84474=CARTESIAN_POINT('Ctrl Pts',(-0.114723552878964,0.116704544205191,
-0.994039168101094));
#84475=CARTESIAN_POINT('Ctrl Pts',(-0.182045051175031,0.0220707951371245,
-0.986649483595708));
#84476=CARTESIAN_POINT('Ctrl Pts',(-0.117521741175058,-0.140994311004445,
-0.975564956837627));
#84477=CARTESIAN_POINT('Ctrl Pts',(0.0542023734324004,-0.175183216767612,
-0.964480430079548));
#84478=CARTESIAN_POINT('Ctrl Pts',(0.17647635671274,-0.0500200511658903,
-0.953395903321467));
#84479=CARTESIAN_POINT('Ctrl Pts',(0.138038040413487,0.120822126492967,
-0.942311376563387));
#84480=CARTESIAN_POINT('Ctrl Pts',(-0.0261604923186076,0.181546629858235,
-0.931226849805308));
#84481=CARTESIAN_POINT('Ctrl Pts',(-0.166518288973121,0.0769318273169837,
-0.920142323047226));
#84482=CARTESIAN_POINT('Ctrl Pts',(-0.155200137290489,-0.097777006996296,
-0.909057796289148));
#84483=CARTESIAN_POINT('Ctrl Pts',(-0.00250686787299496,-0.183411833934768,
-0.897973269531066));
#84484=CARTESIAN_POINT('Ctrl Pts',(0.152468303420884,-0.101981132945721,
-0.886888742772987));
#84485=CARTESIAN_POINT('Ctrl Pts',(0.168560695380791,0.0723467668780286,
-0.875804216014907));
#84486=CARTESIAN_POINT('Ctrl Pts',(0.0311104340172021,0.180772608850168,
-0.864719689256827));
#84487=CARTESIAN_POINT('Ctrl Pts',(-0.134678138991185,0.124533056899584,
-0.853635162498746));
#84488=CARTESIAN_POINT('Ctrl Pts',(-0.17778829995743,-0.0451442083670213,
-0.842550635740667));
#84489=CARTESIAN_POINT('Ctrl Pts',(-0.0589507469967352,-0.173699357167665,
-0.831466108982587));
#84490=CARTESIAN_POINT('Ctrl Pts',(0.113585102895841,-0.144031577598204,
-0.820381582224506));
#84491=CARTESIAN_POINT('Ctrl Pts',(0.182656116776244,0.0168348494932255,
-0.809297055466426));
#84492=CARTESIAN_POINT('Ctrl Pts',(0.0853453694751092,0.162366358308449,
-0.798212528708347));
#84493=CARTESIAN_POINT('Ctrl Pts',(-0.0897066078766045,0.159998103029135,
-0.787128001950266));
#84494=CARTESIAN_POINT('Ctrl Pts',(-0.183044693750403,0.0118873098484331,
-0.776043475192187));
#84495=CARTESIAN_POINT('Ctrl Pts',(-0.109647071009597,-0.147051649214227,
-0.764958948434105));
#84496=CARTESIAN_POINT('Ctrl Pts',(0.0636282451524521,-0.172041025459065,
-0.753874421676027));
#84497=CARTESIAN_POINT('Ctrl Pts',(0.178944490378705,-0.0403179525962051,
-0.742789894917946));
#84498=CARTESIAN_POINT('Ctrl Pts',(0.131259910019175,0.128130807864812,
-0.731705368159865));
#84499=CARTESIAN_POINT('Ctrl Pts',(-0.0359895343390016,0.179865008726402,
-0.720620841401787));
#84500=CARTESIAN_POINT('Ctrl Pts',(-0.170456053776628,0.0677598823930454,
-0.709536314643705));
#84501=CARTESIAN_POINT('Ctrl Pts',(-0.149653878410367,-0.106067830204563,
-0.698451787885626));
#84502=CARTESIAN_POINT('Ctrl Pts',(0.00746825656729185,-0.183278184947211,
-0.687367261127545));
#84503=CARTESIAN_POINT('Ctrl Pts',(0.157787544579823,-0.0935401448930603,
-0.676282734369466));
#84504=CARTESIAN_POINT('Ctrl Pts',(0.164377903307406,0.0814037642567962,
-0.665198207611385));
#84505=CARTESIAN_POINT('Ctrl Pts',(0.0212361643438886,0.182196853034596,
-0.654113680853305));
#84506=CARTESIAN_POINT('Ctrl Pts',(-0.14124963103096,0.117026534020937,
-0.643029154095226));
#84507=CARTESIAN_POINT('Ctrl Pts',(-0.175070909294838,-0.0547434438998959,
-0.631944627337146));
#84508=CARTESIAN_POINT('Ctrl Pts',(-0.0494198134360999,-0.176647530329169,
-0.620860100579064));
#84509=CARTESIAN_POINT('Ctrl Pts',(0.121247870324878,-0.137643095987666,
-0.609775573820986));
#84510=CARTESIAN_POINT('Ctrl Pts',(0.1814706731176,0.0267406568662764,-0.598691047062905));
#84511=CARTESIAN_POINT('Ctrl Pts',(0.0763915465817655,0.166766302178392,
-0.587606520304825));
#84512=CARTESIAN_POINT('Ctrl Pts',(-0.0982727631543477,0.154884253406886,
-0.576521993546745));
#84513=CARTESIAN_POINT('Ctrl Pts',(-0.183420254162722,0.00191788797457964,
-0.565437466788665));
#84514=CARTESIAN_POINT('Ctrl Pts',(-0.101489939318737,-0.152795484712349,
-0.554352940030585));
#84515=CARTESIAN_POINT('Ctrl Pts',(0.0728877252188209,-0.168327203516921,
-0.543268413272505));
#84516=CARTESIAN_POINT('Ctrl Pts',(0.180871843096437,-0.0305294006868705,
-0.532183886514424));
#84517=CARTESIAN_POINT('Ctrl Pts',(0.124099506879204,0.135077682552448,
-0.521099359756346));
#84518=CARTESIAN_POINT('Ctrl Pts',(-0.0457152706506643,0.177642286521926,
-0.510014832998264));
#84519=CARTESIAN_POINT('Ctrl Pts',(-0.173887934286807,0.0583922446979787,
-0.498930306240185));
#84520=CARTESIAN_POINT('Ctrl Pts',(-0.143665797646062,-0.114047387160434,
-0.487845779482104));
#84521=CARTESIAN_POINT('Ctrl Pts',(0.0174217461783371,-0.182601069798343,
-0.476761252724024));
#84522=CARTESIAN_POINT('Ctrl Pts',(0.162639793262148,-0.0848231429448783,
-0.465676725965944));
#84523=CARTESIAN_POINT('Ctrl Pts',(0.159708989901038,0.0902203218581661,
-0.454592199207864));
#84524=CARTESIAN_POINT('Ctrl Pts',(0.0112990096116807,0.183081949719785,
-0.443507672449784));
#84525=CARTESIAN_POINT('Ctrl Pts',(-0.147403256787751,0.109173933792666,
-0.432423145691704));
#84526=CARTESIAN_POINT('Ctrl Pts',(-0.171835658433079,-0.0641807948086411,
-0.421338618933623));
#84527=CARTESIAN_POINT('Ctrl Pts',(-0.039742681192371,-0.179073133727677,
-0.410254092175544));
#84528=CARTESIAN_POINT('Ctrl Pts',(0.128551968555153,-0.130847465821811,
-0.399169565417463));
#84529=CARTESIAN_POINT('Ctrl Pts',(0.179748422455937,0.0365673700994489,
-0.388085038659384));
#84530=CARTESIAN_POINT('Ctrl Pts',(0.0672117479383925,0.17067292951877,
-0.377000511901303));
#84531=CARTESIAN_POINT('Ctrl Pts',(-0.106548216364339,0.149312241698129,
-0.365915985143223));
#84532=CARTESIAN_POINT('Ctrl Pts',(-0.183253238240171,-0.00805720831474408,
-0.354831458385143));
#84533=CARTESIAN_POINT('Ctrl Pts',(-0.0930325893378739,-0.158087334258128,
-0.343746931627063));
#84534=CARTESIAN_POINT('Ctrl Pts',(0.0819315954977009,-0.164115452015086,
-0.332662404868983));
#84535=CARTESIAN_POINT('Ctrl Pts',(0.182264157622932,-0.0206505393912029,
-0.321577878110903));
#84536=CARTESIAN_POINT('Ctrl Pts',(0.116572004105514,0.14162498293918,-0.310493351352823));
#84537=CARTESIAN_POINT('Ctrl Pts',(-0.0553057762937551,0.17489407947702,
-0.299408824594743));
#84538=CARTESIAN_POINT('Ctrl Pts',(-0.176805435700639,0.0488518765015995,
-0.288324297836663));
#84539=CARTESIAN_POINT('Ctrl Pts',(-0.137252738105612,-0.121689579786436,
-0.277239771078583));
#84540=CARTESIAN_POINT('Ctrl Pts',(0.0273237004269018,-0.181383801088499,
-0.266155244320502));
#84541=CARTESIAN_POINT('Ctrl Pts',(0.167010936000477,-0.075855225229966,
-0.255070717562423));
#84542=CARTESIAN_POINT('Ctrl Pts',(0.154567640328825,0.098769998407238,
-0.243986190804342));
#84543=CARTESIAN_POINT('Ctrl Pts',(0.00132843101394552,0.183425469847153,
-0.232901664046263));
#84544=CARTESIAN_POINT('Ctrl Pts',(-0.153120847597592,0.100998386504967,
-0.221817137288183));
#84545=CARTESIAN_POINT('Ctrl Pts',(-0.168092100005951,-0.0734282941735533,
-0.210732610530102));
#84546=CARTESIAN_POINT('Ctrl Pts',(-0.0299479845542862,-0.180969015641703,
-0.199648083772023));
#84547=CARTESIAN_POINT('Ctrl Pts',(0.135475793855047,-0.123664782507313,
-0.188563557013942));
#84548=CARTESIAN_POINT('Ctrl Pts',(0.177494461442691,0.0462859276935804,
-0.177479030255862));
#84549=CARTESIAN_POINT('Ctrl Pts',(0.0578331208192682,0.174074660385242,
-0.166394503497782));
#84550=CARTESIAN_POINT('Ctrl Pts',(-0.114508471537225,0.14329860116919,
-0.155309976739702));
#84551=CARTESIAN_POINT('Ctrl Pts',(-0.182544172064818,-0.0180085709609084,
-0.144225449981622));
#84552=CARTESIAN_POINT('Ctrl Pts',(-0.084299977295163,-0.162911353328334,
-0.133140923223542));
#84553=CARTESIAN_POINT('Ctrl Pts',(0.0907329858453492,-0.15941859359732,
-0.122056396465462));
#84554=CARTESIAN_POINT('Ctrl Pts',(0.183117539039973,-0.0107098982665486,
-0.110971869707382));
#84555=CARTESIAN_POINT('Ctrl Pts',(0.108699242850674,0.14775202136532,-0.0998873429493014));
#84556=CARTESIAN_POINT('Ctrl Pts',(-0.0647318703529614,0.1716310306231,
-0.0888028161912215));
#84557=CARTESIAN_POINT('Ctrl Pts',(-0.179201472288944,0.0391622132462028,
-0.0777182894331414));
#84558=CARTESIAN_POINT('Ctrl Pts',(-0.130430729224305,-0.128962688577941,
-0.0666337626750612));
#84559=CARTESIAN_POINT('Ctrl Pts',(0.0371392267897813,-0.179647334199356,
-0.0555492359169813));
#84560=CARTESIAN_POINT('Ctrl Pts',(0.170898721259193,-0.0666298511870843,
-0.0444647091589011));
#84561=CARTESIAN_POINT('Ctrl Pts',(0.14894861527182,0.106964324573014,-0.0333801824008211));
#84562=CARTESIAN_POINT('Ctrl Pts',(-0.00860614795259104,0.183348546767771,
-0.0222956556427411));
#84563=CARTESIAN_POINT('Ctrl Pts',(-0.158470039306694,0.0922754967336385,
-0.0112111288846609));
#84564=CARTESIAN_POINT('Ctrl Pts',(-0.161908972733501,-0.0238102660988092,
-0.00382144437927415));
#84565=CARTESIAN_POINT('Ctrl Pts',(-0.138751033761026,-0.0698268057214688,
-0.000126602126580784));
#84566=CARTESIAN_POINT('Ctrl Pts',(-0.0744116356088496,0.151480899730365,
-0.989974424426066));
#84567=CARTESIAN_POINT('Ctrl Pts',(-0.124650013194736,0.126802409880127,
-0.986279582173373));
#84568=CARTESIAN_POINT('Ctrl Pts',(-0.197796507007979,0.0239804716296012,
-0.978889897667986));
#84569=CARTESIAN_POINT('Ctrl Pts',(-0.127690314852737,-0.153193849789752,
-0.967805370909905));
#84570=CARTESIAN_POINT('Ctrl Pts',(0.0588922361100749,-0.190340952085206,
-0.956720844151826));
#84571=CARTESIAN_POINT('Ctrl Pts',(0.191745981019349,-0.0543480382307185,
-0.945636317393745));
#84572=CARTESIAN_POINT('Ctrl Pts',(0.149981787759574,0.131276266151323,
-0.934551790635665));
#84573=CARTESIAN_POINT('Ctrl Pts',(-0.0284240300344901,0.197254959765447,
-0.923467263877585));
#84574=CARTESIAN_POINT('Ctrl Pts',(-0.180926291042983,0.083588356963409,
-0.912382737119506));
#84575=CARTESIAN_POINT('Ctrl Pts',(-0.16862883580231,-0.106237166705329,
-0.901298210361425));
#84576=CARTESIAN_POINT('Ctrl Pts',(-0.0027237747228427,-0.199281550704414,
-0.890213683603345));
#84577=CARTESIAN_POINT('Ctrl Pts',(0.165660629890387,-0.1108050548322,-0.879129156845265));
#84578=CARTESIAN_POINT('Ctrl Pts',(0.183145416752364,0.0786065739740197,
-0.868044630087185));
#84579=CARTESIAN_POINT('Ctrl Pts',(0.0338022656501029,0.196413966556576,
-0.856960103329105));
#84580=CARTESIAN_POINT('Ctrl Pts',(-0.146331170723112,0.135308284969968,
-0.845875576571024));
#84581=CARTESIAN_POINT('Ctrl Pts',(-0.193171440209355,-0.0490503129252965,
-0.834791049812945));
#84582=CARTESIAN_POINT('Ctrl Pts',(-0.0640514628999968,-0.188728701469957,
-0.823706523054863));
#84583=CARTESIAN_POINT('Ctrl Pts',(0.123413058778169,-0.156493916005342,
-0.812621996296785));
#84584=CARTESIAN_POINT('Ctrl Pts',(0.198460445086451,0.0182914855650937,
-0.801537469538704));
#84585=CARTESIAN_POINT('Ctrl Pts',(0.0927298812163344,0.176415114400109,
-0.790452942780624));
#84586=CARTESIAN_POINT('Ctrl Pts',(-0.0974684759569022,0.173841945731542,
-0.779368416022544));
#84587=CARTESIAN_POINT('Ctrl Pts',(-0.198882643699906,0.0129158598410958,
-0.768283889264463));
#84588=CARTESIAN_POINT('Ctrl Pts',(-0.119134288514671,-0.159775299447008,
-0.757199362506384));
#84589=CARTESIAN_POINT('Ctrl Pts',(0.069133681783536,-0.186926882539398,
-0.746114835748302));
#84590=CARTESIAN_POINT('Ctrl Pts',(0.194427670056241,-0.0438064651676544,
-0.735030308990224));
#84591=CARTESIAN_POINT('Ctrl Pts',(0.142617179343217,0.139217331491218,
-0.723945782232142));
#84592=CARTESIAN_POINT('Ctrl Pts',(-0.039103530335761,0.195427836293314,
-0.712861255474064));
#84593=CARTESIAN_POINT('Ctrl Pts',(-0.185204771114401,0.073622809112947,
-0.701776728715982));
#84594=CARTESIAN_POINT('Ctrl Pts',(-0.162602686635556,-0.115245353746014,
-0.690692201957904));
#84595=CARTESIAN_POINT('Ctrl Pts',(0.008114447785945,-0.199136337732496,
-0.679607675199823));
#84596=CARTESIAN_POINT('Ctrl Pts',(0.171440118617931,-0.101633709927542,
-0.668523148441744));
#84597=CARTESIAN_POINT('Ctrl Pts',(0.178600708416069,0.0884472284380528,
-0.657438621683664));
#84598=CARTESIAN_POINT('Ctrl Pts',(0.0230736243713112,0.197961443529929,
-0.646354094925584));
#84599=CARTESIAN_POINT('Ctrl Pts',(-0.153471261392474,0.127152259878442,
-0.635269568167503));
#84600=CARTESIAN_POINT('Ctrl Pts',(-0.19021892720355,-0.0594801227228939,
-0.624185041409425));
#84601=CARTESIAN_POINT('Ctrl Pts',(-0.0536958649057056,-0.191931965440254,
-0.613100514651342));
#84602=CARTESIAN_POINT('Ctrl Pts',(0.131738847486486,-0.149552670750429,
-0.602015987893264));
#84603=CARTESIAN_POINT('Ctrl Pts',(0.197172430864581,0.0290543933444405,
-0.590931461135182));
#84604=CARTESIAN_POINT('Ctrl Pts',(0.0830013284144861,0.18119576360144,
-0.579846934377105));
#84605=CARTESIAN_POINT('Ctrl Pts',(-0.106775818186142,0.16828562005218,
-0.56876240761902));
#84606=CARTESIAN_POINT('Ctrl Pts',(-0.199290699492951,0.00208383331354575,
-0.557677880860944));
#84607=CARTESIAN_POINT('Ctrl Pts',(-0.11027136065565,-0.166016120557078,
-0.546593354102861));
#84608=CARTESIAN_POINT('Ctrl Pts',(0.0791943387583679,-0.182891721994993,
-0.535508827344784));
#84609=CARTESIAN_POINT('Ctrl Pts',(0.196521787050244,-0.0331709583860329,
-0.524424300586703));
#84610=CARTESIAN_POINT('Ctrl Pts',(0.134837222015547,0.14676528480809,-0.513339773828623));
#84611=CARTESIAN_POINT('Ctrl Pts',(-0.0496707863974368,0.193012792955104,
-0.502255247070543));
#84612=CARTESIAN_POINT('Ctrl Pts',(-0.188933595232391,0.0634446361659716,
-0.491170720312461));
#84613=CARTESIAN_POINT('Ctrl Pts',(-0.156096486927209,-0.123915342208513,
-0.480086193554382));
#84614=CARTESIAN_POINT('Ctrl Pts',(0.0189291635109664,-0.198400635166434,
-0.469001666796301));
#84615=CARTESIAN_POINT('Ctrl Pts',(0.176712208324863,-0.092162469013257,
-0.457917140038222));
#84616=CARTESIAN_POINT('Ctrl Pts',(0.173527817077681,0.0980266390626729,
-0.446832613280141));
#84617=CARTESIAN_POINT('Ctrl Pts',(0.0122766569012164,0.19892312324363,
-0.435748086522061));
#84618=CARTESIAN_POINT('Ctrl Pts',(-0.160157329880857,0.118620213079824,
-0.424663559763982));
#84619=CARTESIAN_POINT('Ctrl Pts',(-0.186703746122714,-0.0697340408223409,
-0.4135790330059));
#84620=CARTESIAN_POINT('Ctrl Pts',(-0.0431814183810181,-0.194567444276481,
-0.402494506247822));
#84621=CARTESIAN_POINT('Ctrl Pts',(0.13967493312829,-0.142169048394049,
-0.391409979489741));
#84622=CARTESIAN_POINT('Ctrl Pts',(0.195301162390815,0.0397313633600757,
-0.380325452731661));
#84623=CARTESIAN_POINT('Ctrl Pts',(0.0730272473011798,0.185440412039401,
-0.369240925973581));
#84624=CARTESIAN_POINT('Ctrl Pts',(-0.115767305338796,0.162231489792192,
-0.358156399215501));
#84625=CARTESIAN_POINT('Ctrl Pts',(-0.199109232510563,-0.00875435860851541,
-0.347071872457421));
#84626=CARTESIAN_POINT('Ctrl Pts',(-0.101082238106252,-0.171765847610963,
-0.335987345699341));
#84627=CARTESIAN_POINT('Ctrl Pts',(0.0890207302996347,-0.178315548514465,
-0.32490281894126));
#84628=CARTESIAN_POINT('Ctrl Pts',(0.198034571650647,-0.0224373281945668,
-0.313818292183181));
#84629=CARTESIAN_POINT('Ctrl Pts',(0.126658401742661,0.153879090640594,
-0.302733765425101));
#84630=CARTESIAN_POINT('Ctrl Pts',(-0.0600911109511644,0.190026797178187,
-0.29164923866702));
#84631=CARTESIAN_POINT('Ctrl Pts',(-0.192103533580739,0.0530787872036758,
-0.280564711908941));
#84632=CARTESIAN_POINT('Ctrl Pts',(-0.149128537135947,-0.132218775878082,
-0.26948018515086));
#84633=CARTESIAN_POINT('Ctrl Pts',(0.0296878847740664,-0.19707804222945,
-0.258395658392781));
#84634=CARTESIAN_POINT('Ctrl Pts',(0.181461564375435,-0.0824186018348015,
-0.2473111316347));
#84635=CARTESIAN_POINT('Ctrl Pts',(0.167941612014008,0.10731607674054,-0.23622660487662));
#84636=CARTESIAN_POINT('Ctrl Pts',(0.00144337356420142,0.1992963664647,
-0.22514207811854));
#84637=CARTESIAN_POINT('Ctrl Pts',(-0.166369635479871,0.109737276213662,
-0.21405755136046));
#84638=CARTESIAN_POINT('Ctrl Pts',(-0.182636276142689,-0.0797816804650109,
-0.20297302460238));
#84639=CARTESIAN_POINT('Ctrl Pts',(-0.0325392351977291,-0.196627367454142,
-0.1918884978443));
#84640=CARTESIAN_POINT('Ctrl Pts',(0.147197842708159,-0.134364883098799,
-0.18080397108622));
#84641=CARTESIAN_POINT('Ctrl Pts',(0.19285217730457,0.0502908195653797,
-0.16971944432814));
#84642=CARTESIAN_POINT('Ctrl Pts',(0.0628371340697605,0.189136477814472,
-0.158634917570059));
#84643=CARTESIAN_POINT('Ctrl Pts',(-0.124416321930711,0.155697518759482,
-0.147550390811979));
#84644=CARTESIAN_POINT('Ctrl Pts',(-0.198338814354084,-0.0195667633329289,
-0.136465864053899));
#84645=CARTESIAN_POINT('Ctrl Pts',(-0.0915940364333415,-0.177007265137383,
-0.125381337295819));
#84646=CARTESIAN_POINT('Ctrl Pts',(0.0985836613232566,-0.173212294221374,
-0.114296810537739));
#84647=CARTESIAN_POINT('Ctrl Pts',(0.198961791931268,-0.0116365726717701,
-0.103212283779659));
#84648=CARTESIAN_POINT('Ctrl Pts',(0.11810444948379,0.160536271328406,-0.0921277570215794));
#84649=CARTESIAN_POINT('Ctrl Pts',(-0.0703327982016847,0.18648141288273,
-0.0810432302634995));
#84650=CARTESIAN_POINT('Ctrl Pts',(-0.194706887337247,0.0425507254210006,
-0.0699587035054193));
#84651=CARTESIAN_POINT('Ctrl Pts',(-0.141716253644635,-0.140121190718603,
-0.0588741767473393));
#84652=CARTESIAN_POINT('Ctrl Pts',(0.0403526999749784,-0.195191327468512,
-0.0477896499892592));
#84653=CARTESIAN_POINT('Ctrl Pts',(0.185685740419814,-0.0723950019085964,
-0.0367051232311792));
#84654=CARTESIAN_POINT('Ctrl Pts',(0.161836400573806,0.116219417328008,
-0.025620596473099));
#84655=CARTESIAN_POINT('Ctrl Pts',(-0.00935079527198692,0.199212787612586,
-0.0145360697150191));
#84656=CARTESIAN_POINT('Ctrl Pts',(-0.172181666230212,0.10025963803208,
-0.00345154295693894));
#84657=CARTESIAN_POINT('Ctrl Pts',(-0.175918153518743,-0.0258704503905826,
0.00393814154844779));
#84658=CARTESIAN_POINT('Ctrl Pts',(-0.150756472886978,-0.0758685730706938,
0.00763298380114117));
#84659=CARTESIAN_POINT('Ctrl Pts',(-0.0803373802515631,0.163544028335269,
-0.982214838498344));
#84660=CARTESIAN_POINT('Ctrl Pts',(-0.134576473510508,0.136900275555064,
-0.97851999624565));
#84661=CARTESIAN_POINT('Ctrl Pts',(-0.213547962840926,0.0258901481220782,
-0.971130311740263));
#84662=CARTESIAN_POINT('Ctrl Pts',(-0.137858888530416,-0.16539338857506,
-0.960045784982185));
#84663=CARTESIAN_POINT('Ctrl Pts',(0.0635820987877494,-0.205498687402797,
-0.948961258224102));
#84664=CARTESIAN_POINT('Ctrl Pts',(0.207015605325956,-0.0586760252955468,
-0.937876731466025));
#84665=CARTESIAN_POINT('Ctrl Pts',(0.161925535105659,0.141730405809681,
-0.926792204707942));
#84666=CARTESIAN_POINT('Ctrl Pts',(-0.0306875677503726,0.212963289672657,
-0.915707677949864));
#84667=CARTESIAN_POINT('Ctrl Pts',(-0.195334293112845,0.0902448866098343,
-0.904623151191783));
#84668=CARTESIAN_POINT('Ctrl Pts',(-0.182057534314132,-0.114697326414361,
-0.893538624433703));
#84669=CARTESIAN_POINT('Ctrl Pts',(-0.00294068157269068,-0.215151267474059,
-0.882454097675622));
#84670=CARTESIAN_POINT('Ctrl Pts',(0.178852956359889,-0.11962897671868,
-0.871369570917544));
#84671=CARTESIAN_POINT('Ctrl Pts',(0.197730138123937,0.0848663810700111,
-0.860285044159461));
#84672=CARTESIAN_POINT('Ctrl Pts',(0.036494097283004,0.212055324262984,
-0.849200517401385));
#84673=CARTESIAN_POINT('Ctrl Pts',(-0.15798420245504,0.146083513040354,
-0.838115990643301));
#84674=CARTESIAN_POINT('Ctrl Pts',(-0.208554580461279,-0.052956417483572,
-0.827031463885224));
#84675=CARTESIAN_POINT('Ctrl Pts',(-0.0691521788032584,-0.203758045772247,
-0.815946937127142));
#84676=CARTESIAN_POINT('Ctrl Pts',(0.133241014660498,-0.16895625441248,
-0.804862410369063));
#84677=CARTESIAN_POINT('Ctrl Pts',(0.214264773396658,0.0197481216369616,
-0.793777883610981));
#84678=CARTESIAN_POINT('Ctrl Pts',(0.10011439295756,0.19046387049177,-0.782693356852903));
#84679=CARTESIAN_POINT('Ctrl Pts',(-0.1052303440372,0.187685788433949,-0.771608830094822));
#84680=CARTESIAN_POINT('Ctrl Pts',(-0.214720593649408,0.0139444098337588,
-0.760524303336743));
#84681=CARTESIAN_POINT('Ctrl Pts',(-0.128621506019745,-0.172498949679788,
-0.749439776578661));
#84682=CARTESIAN_POINT('Ctrl Pts',(0.0746391184146198,-0.201812739619732,
-0.738355249820582));
#84683=CARTESIAN_POINT('Ctrl Pts',(0.209910849733778,-0.0472949777391037,
-0.727270723062502));
#84684=CARTESIAN_POINT('Ctrl Pts',(0.153974448667259,0.150303855117625,
-0.716186196304421));
#84685=CARTESIAN_POINT('Ctrl Pts',(-0.0422175263325201,0.210990663860225,
-0.705101669546343));
#84686=CARTESIAN_POINT('Ctrl Pts',(-0.199953488452174,0.079485735832849,
-0.69401714278826));
#84687=CARTESIAN_POINT('Ctrl Pts',(-0.175551494860746,-0.124422877287465,
-0.682932616030183));
#84688=CARTESIAN_POINT('Ctrl Pts',(0.00876063900459808,-0.214994490517782,
-0.671848089272101));
#84689=CARTESIAN_POINT('Ctrl Pts',(0.185092692656038,-0.109727274962025,
-0.660763562514022));
#84690=CARTESIAN_POINT('Ctrl Pts',(0.192823513524732,0.0954906926193094,
-0.649679035755941));
#84691=CARTESIAN_POINT('Ctrl Pts',(0.0249110843987339,0.213726034025263,
-0.638594508997861));
#84692=CARTESIAN_POINT('Ctrl Pts',(-0.165692891753988,0.137277985735947,
-0.627509982239781));
#84693=CARTESIAN_POINT('Ctrl Pts',(-0.20536694511226,-0.0642168015458922,
-0.616425455481702));
#84694=CARTESIAN_POINT('Ctrl Pts',(-0.0579719163753115,-0.207216400551339,
-0.60534092872362));
#84695=CARTESIAN_POINT('Ctrl Pts',(0.142229824648094,-0.161462245513192,
-0.594256401965542));
#84696=CARTESIAN_POINT('Ctrl Pts',(0.212874188611563,0.0313681298226046,
-0.58317187520746));
#84697=CARTESIAN_POINT('Ctrl Pts',(0.0896111102472069,0.195625225024487,
-0.572087348449381));
#84698=CARTESIAN_POINT('Ctrl Pts',(-0.115278873217937,0.181686986697472,
-0.561002821691301));
#84699=CARTESIAN_POINT('Ctrl Pts',(-0.21516114482318,0.00224977865251208,
-0.549918294933221));
#84700=CARTESIAN_POINT('Ctrl Pts',(-0.119052781992563,-0.179236756401807,
-0.53883376817514));
#84701=CARTESIAN_POINT('Ctrl Pts',(0.0855009522979151,-0.197456240473065,
-0.527749241417061));
#84702=CARTESIAN_POINT('Ctrl Pts',(0.212171731004051,-0.0358125160851952,
-0.51666471465898));
#84703=CARTESIAN_POINT('Ctrl Pts',(0.14557493715189,0.15845288706373,-0.505580187900901));
#84704=CARTESIAN_POINT('Ctrl Pts',(-0.05362630214421,0.208383299388281,
-0.49449566114282));
#84705=CARTESIAN_POINT('Ctrl Pts',(-0.203979256177974,0.0684970276339647,
-0.483411134384741));
#84706=CARTESIAN_POINT('Ctrl Pts',(-0.168527176208356,-0.133783297256591,
-0.47232660762666));
#84707=CARTESIAN_POINT('Ctrl Pts',(0.0204365808435957,-0.214200200534527,
-0.46124208086858));
#84708=CARTESIAN_POINT('Ctrl Pts',(0.190784623387578,-0.0995017950816356,
-0.4501575541105));
#84709=CARTESIAN_POINT('Ctrl Pts',(0.187346644254324,0.10583295626718,-0.43907302735242));
#84710=CARTESIAN_POINT('Ctrl Pts',(0.0132543041907522,0.214764296767476,
-0.427988500594339));
#84711=CARTESIAN_POINT('Ctrl Pts',(-0.172911402973964,0.128066492366983,
-0.416903973836261));
#84712=CARTESIAN_POINT('Ctrl Pts',(-0.201571833812347,-0.0752872868360405,
-0.405819447078179));
#84713=CARTESIAN_POINT('Ctrl Pts',(-0.0466201555696652,-0.210061754825286,
-0.3947349203201));
#84714=CARTESIAN_POINT('Ctrl Pts',(0.150797897701427,-0.153490630966287,
-0.383650393562019));
#84715=CARTESIAN_POINT('Ctrl Pts',(0.210853902325691,0.0428953566207025,
-0.372565866803939));
#84716=CARTESIAN_POINT('Ctrl Pts',(0.0788427466639674,0.200207894560031,
-0.361481340045859));
#84717=CARTESIAN_POINT('Ctrl Pts',(-0.124986394313251,0.175150737886255,
-0.350396813287779));
#84718=CARTESIAN_POINT('Ctrl Pts',(-0.214965226780956,-0.00945150890228677,
-0.3393122865297));
#84719=CARTESIAN_POINT('Ctrl Pts',(-0.109131886874631,-0.185444360963798,
-0.328227759771619));
#84720=CARTESIAN_POINT('Ctrl Pts',(0.0961098651015682,-0.192515645013844,
-0.317143233013539));
#84721=CARTESIAN_POINT('Ctrl Pts',(0.213804985678363,-0.0242241169979305,
-0.306058706255459));
#84722=CARTESIAN_POINT('Ctrl Pts',(0.13674479937981,0.166133198342007,-0.294974179497379));
#84723=CARTESIAN_POINT('Ctrl Pts',(-0.0648764456085735,0.205159514879355,
-0.283889652739298));
#84724=CARTESIAN_POINT('Ctrl Pts',(-0.20740163146084,0.0573056979057522,
-0.272805125981219));
#84725=CARTESIAN_POINT('Ctrl Pts',(-0.161004336166281,-0.142747971969729,
-0.261720599223138));
#84726=CARTESIAN_POINT('Ctrl Pts',(0.0320520691212311,-0.2127722833704,
-0.250636072465059));
#84727=CARTESIAN_POINT('Ctrl Pts',(0.195912192750394,-0.0889819784396372,
-0.239551545706979));
#84728=CARTESIAN_POINT('Ctrl Pts',(0.181315583699191,0.11586215507384,-0.228467018948898));
#84729=CARTESIAN_POINT('Ctrl Pts',(0.0015583161144573,0.215167263082248,
-0.217382492190819));
#84730=CARTESIAN_POINT('Ctrl Pts',(-0.179618423362151,0.118476165922355,
-0.206297965432738));
#84731=CARTESIAN_POINT('Ctrl Pts',(-0.197180452279427,-0.0861350667564684,
-0.195213438674658));
#84732=CARTESIAN_POINT('Ctrl Pts',(-0.0351304858411718,-0.212285719266582,
-0.184128911916578));
#84733=CARTESIAN_POINT('Ctrl Pts',(0.158919891561272,-0.145064983690286,
-0.173044385158498));
#84734=CARTESIAN_POINT('Ctrl Pts',(0.20820989316645,0.054295711437179,-0.161959858400418));
#84735=CARTESIAN_POINT('Ctrl Pts',(0.0678411473202531,0.204198295243703,
-0.150875331642338));
#84736=CARTESIAN_POINT('Ctrl Pts',(-0.134324172324197,0.168096436349775,
-0.139790804884258));
#84737=CARTESIAN_POINT('Ctrl Pts',(-0.214133456643352,-0.0211249557049494,
-0.128706278126178));
#84738=CARTESIAN_POINT('Ctrl Pts',(-0.0988880955715197,-0.191103176946429,
-0.117621751368098));
#84739=CARTESIAN_POINT('Ctrl Pts',(0.106434336801163,-0.187005994845427,
-0.106537224610018));
#84740=CARTESIAN_POINT('Ctrl Pts',(0.214806044822565,-0.0125632470769915,
-0.0954526978519376));
#84741=CARTESIAN_POINT('Ctrl Pts',(0.127509656116906,0.173320521291492,
-0.0843681710938575));
#84742=CARTESIAN_POINT('Ctrl Pts',(-0.075933726050408,0.20133179514236,
-0.0732836443357776));
#84743=CARTESIAN_POINT('Ctrl Pts',(-0.21021230238555,0.045939237595798,
-0.0621991175776973));
#84744=CARTESIAN_POINT('Ctrl Pts',(-0.153001778064964,-0.151279692859263,
-0.0511145908196174));
#84745=CARTESIAN_POINT('Ctrl Pts',(0.0435661731601757,-0.210735320737669,
-0.0400300640615372));
#84746=CARTESIAN_POINT('Ctrl Pts',(0.200472759580433,-0.0781601526301082,
-0.0289455373034573));
#84747=CARTESIAN_POINT('Ctrl Pts',(0.174724185875792,0.125474510083003,
-0.0178610105453771));
#84748=CARTESIAN_POINT('Ctrl Pts',(-0.0100954425913831,0.215077028457403,
-0.00677648378729714));
#84749=CARTESIAN_POINT('Ctrl Pts',(-0.185893293153729,0.10824377933052,
0.00430804297078301));
#84750=CARTESIAN_POINT('Ctrl Pts',(-0.189927334303986,-0.0279306346823561,
0.0116977274761698));
#84751=CARTESIAN_POINT('Ctrl Pts',(-0.16276191201293,-0.081910340419919,
0.0153925697288631));
#84752=CARTESIAN_POINT('Ctrl Pts',(-0.0862631248942766,0.175607156940174,
-0.974455252570622));
#84753=CARTESIAN_POINT('Ctrl Pts',(-0.14450293382628,0.146998141230001,
-0.970760410317929));
#84754=CARTESIAN_POINT('Ctrl Pts',(-0.229299418673872,0.0277998246145549,
-0.963370725812542));
#84755=CARTESIAN_POINT('Ctrl Pts',(-0.148027462208095,-0.177592927360367,
-0.952286199054462));
#84756=CARTESIAN_POINT('Ctrl Pts',(0.0682719614654239,-0.22065642272039,
-0.941201672296381));
#84757=CARTESIAN_POINT('Ctrl Pts',(0.222285229632565,-0.0630040123603747,
-0.930117145538302));
#84758=CARTESIAN_POINT('Ctrl Pts',(0.173869282451744,0.152184545468037,
-0.919032618780222));
#84759=CARTESIAN_POINT('Ctrl Pts',(-0.0329511054662551,0.228671619579868,
-0.907948092022141));
#84760=CARTESIAN_POINT('Ctrl Pts',(-0.209742295182707,0.0969014162562596,
-0.896863565264062));
#84761=CARTESIAN_POINT('Ctrl Pts',(-0.195486232825953,-0.123157486123393,
-0.885779038505981));
#84762=CARTESIAN_POINT('Ctrl Pts',(-0.00315758842253853,-0.231020984243704,
-0.874694511747901));
#84763=CARTESIAN_POINT('Ctrl Pts',(0.192045282829392,-0.128452898605159,
-0.863609984989822));
#84764=CARTESIAN_POINT('Ctrl Pts',(0.212314859495509,0.0911261881660022,
-0.852525458231741));
#84765=CARTESIAN_POINT('Ctrl Pts',(0.0391859289159049,0.227696681969392,
-0.841440931473661));
#84766=CARTESIAN_POINT('Ctrl Pts',(-0.169637234186967,0.156858741110739,
-0.830356404715581));
#84767=CARTESIAN_POINT('Ctrl Pts',(-0.223937720713203,-0.0568625220418472,
-0.819271877957501));
#84768=CARTESIAN_POINT('Ctrl Pts',(-0.0742528947065199,-0.218787390074539,
-0.808187351199421));
#84769=CARTESIAN_POINT('Ctrl Pts',(0.143068970542826,-0.181418592819617,
-0.79710282444134));
#84770=CARTESIAN_POINT('Ctrl Pts',(0.230069101706865,0.0212047577088296,
-0.786018297683261));
#84771=CARTESIAN_POINT('Ctrl Pts',(0.107498904698785,0.204512626583431,
-0.77493377092518));
#84772=CARTESIAN_POINT('Ctrl Pts',(-0.112992212117498,0.201529631136357,
-0.763849244167102));
#84773=CARTESIAN_POINT('Ctrl Pts',(-0.230558543598911,0.0149729598264217,
-0.752764717409019));
#84774=CARTESIAN_POINT('Ctrl Pts',(-0.13810872352482,-0.18522259991257,
-0.741680190650942));
#84775=CARTESIAN_POINT('Ctrl Pts',(0.0801445550457034,-0.216698596700065,
-0.73059566389286));
#84776=CARTESIAN_POINT('Ctrl Pts',(0.225394029411315,-0.050783490310553,
-0.719511137134781));
#84777=CARTESIAN_POINT('Ctrl Pts',(0.165331717991301,0.161390378744031,
-0.708426610376699));
#84778=CARTESIAN_POINT('Ctrl Pts',(-0.0453315223292791,0.226553491427137,
-0.697342083618621));
#84779=CARTESIAN_POINT('Ctrl Pts',(-0.214702205789946,0.0853486625527506,
-0.686257556860539));
#84780=CARTESIAN_POINT('Ctrl Pts',(-0.188500303085936,-0.133600400828916,
-0.675173030102461));
#84781=CARTESIAN_POINT('Ctrl Pts',(0.00940683022325126,-0.230852643303067,
-0.664088503344379));
#84782=CARTESIAN_POINT('Ctrl Pts',(0.198745266694145,-0.117820839996506,
-0.6530039765863));
#84783=CARTESIAN_POINT('Ctrl Pts',(0.207046318633396,0.102534156800566,
-0.641919449828219));
#84784=CARTESIAN_POINT('Ctrl Pts',(0.0267485444261562,0.229490624520597,
-0.630834923070141));
#84785=CARTESIAN_POINT('Ctrl Pts',(-0.177914522115502,0.147403711593452,
-0.619750396312058));
#84786=CARTESIAN_POINT('Ctrl Pts',(-0.220514963020972,-0.0689534803688902,
-0.608665869553981));
#84787=CARTESIAN_POINT('Ctrl Pts',(-0.0622479678449172,-0.222500835662425,
-0.597581342795898));
#84788=CARTESIAN_POINT('Ctrl Pts',(0.152720801809701,-0.173371820275954,
-0.58649681603782));
#84789=CARTESIAN_POINT('Ctrl Pts',(0.228575946358543,0.0336818663007685,
-0.575412289279738));
#84790=CARTESIAN_POINT('Ctrl Pts',(0.0962208920799274,0.210054686447534,
-0.56432776252166));
#84791=CARTESIAN_POINT('Ctrl Pts',(-0.123781928249732,0.195088353342765,
-0.553243235763578));
#84792=CARTESIAN_POINT('Ctrl Pts',(-0.23103159015341,0.00241572399147842,
-0.5421587090055));
#84793=CARTESIAN_POINT('Ctrl Pts',(-0.127834203329475,-0.192457392246536,
-0.531074182247418));
#84794=CARTESIAN_POINT('Ctrl Pts',(0.0918075658374621,-0.212020758951138,
-0.519989655489339));
#84795=CARTESIAN_POINT('Ctrl Pts',(0.227821674957858,-0.0384540737843577,
-0.508905128731259));
#84796=CARTESIAN_POINT('Ctrl Pts',(0.156312652288233,0.170140489319371,
-0.497820601973179));
#84797=CARTESIAN_POINT('Ctrl Pts',(-0.0575818178909828,0.223753805821459,
-0.486736075215099));
#84798=CARTESIAN_POINT('Ctrl Pts',(-0.219024917123558,0.0735494191019577,
-0.475651548457019));
#84799=CARTESIAN_POINT('Ctrl Pts',(-0.180957865489502,-0.14365125230467,
-0.464567021698939));
#84800=CARTESIAN_POINT('Ctrl Pts',(0.0219439981762253,-0.229999765902618,
-0.453482494940859));
#84801=CARTESIAN_POINT('Ctrl Pts',(0.204857038450294,-0.106841121150014,
-0.442397968182778));
#84802=CARTESIAN_POINT('Ctrl Pts',(0.201165471430968,0.113639273471686,
-0.431313441424699));
#84803=CARTESIAN_POINT('Ctrl Pts',(0.014231951480288,0.230605470291321,
-0.420228914666617));
#84804=CARTESIAN_POINT('Ctrl Pts',(-0.185665476067071,0.137512771654142,
-0.409144387908539));
#84805=CARTESIAN_POINT('Ctrl Pts',(-0.21643992150198,-0.0808405328497407,
-0.398059861150457));
#84806=CARTESIAN_POINT('Ctrl Pts',(-0.0500588927583125,-0.225556065374089,
-0.386975334392379));
#84807=CARTESIAN_POINT('Ctrl Pts',(0.161920862274563,-0.164812213538526,
-0.375890807634297));
#84808=CARTESIAN_POINT('Ctrl Pts',(0.226406642260568,0.0460593498813293,
-0.364806280876218));
#84809=CARTESIAN_POINT('Ctrl Pts',(0.0846582460267547,0.214975377080661,
-0.353721754118138));
#84810=CARTESIAN_POINT('Ctrl Pts',(-0.134205483287707,0.188069985980317,
-0.342637227360058));
#84811=CARTESIAN_POINT('Ctrl Pts',(-0.230821221051348,-0.0101486591960582,
-0.331552700601978));
#84812=CARTESIAN_POINT('Ctrl Pts',(-0.117181535643009,-0.199122874316633,
-0.320468173843897));
#84813=CARTESIAN_POINT('Ctrl Pts',(0.103198999903502,-0.206715741513223,
-0.309383647085818));
#84814=CARTESIAN_POINT('Ctrl Pts',(0.229575399706078,-0.0260109058012938,
-0.298299120327737));
#84815=CARTESIAN_POINT('Ctrl Pts',(0.146831197016957,0.178387306043421,
-0.287214593569658));
#84816=CARTESIAN_POINT('Ctrl Pts',(-0.0696617802659827,0.220292232580522,
-0.276130066811577));
#84817=CARTESIAN_POINT('Ctrl Pts',(-0.22269972934094,0.0615326086078283,
-0.265045540053497));
#84818=CARTESIAN_POINT('Ctrl Pts',(-0.172880135196616,-0.153277168061375,
-0.253961013295417));
#84819=CARTESIAN_POINT('Ctrl Pts',(0.0344162534683956,-0.228466524511351,
-0.242876486537337));
#84820=CARTESIAN_POINT('Ctrl Pts',(0.210362821125352,-0.0955453550444726,
-0.231791959779257));
#84821=CARTESIAN_POINT('Ctrl Pts',(0.194689555384374,0.124408233407141,
-0.220707433021177));
#84822=CARTESIAN_POINT('Ctrl Pts',(0.0016732586647134,0.231038159699794,
-0.209622906263097));
#84823=CARTESIAN_POINT('Ctrl Pts',(-0.192867211244431,0.127215055631049,
-0.198538379505017));
#84824=CARTESIAN_POINT('Ctrl Pts',(-0.211724628416165,-0.0924884530479261,
-0.187453852746937));
#84825=CARTESIAN_POINT('Ctrl Pts',(-0.0377217364846146,-0.22794407107902,
-0.176369325988857));
#84826=CARTESIAN_POINT('Ctrl Pts',(0.170641940414384,-0.155765084281773,
-0.165284799230776));
#84827=CARTESIAN_POINT('Ctrl Pts',(0.223567609028329,0.0583006033089783,
-0.154200272472697));
#84828=CARTESIAN_POINT('Ctrl Pts',(0.0728451605707456,0.219260112672934,
-0.143115745714616));
#84829=CARTESIAN_POINT('Ctrl Pts',(-0.144232022717683,0.180495353940067,
-0.132031218956536));
#84830=CARTESIAN_POINT('Ctrl Pts',(-0.229928098932619,-0.0226831480769699,
-0.120946692198456));
#84831=CARTESIAN_POINT('Ctrl Pts',(-0.106182154709698,-0.205199088755477,
-0.109862165440376));
#84832=CARTESIAN_POINT('Ctrl Pts',(0.114285012279071,-0.200799695469481,
-0.0987776386822957));
#84833=CARTESIAN_POINT('Ctrl Pts',(0.230650297713861,-0.0134899214822133,
-0.0876931119242156));
#84834=CARTESIAN_POINT('Ctrl Pts',(0.136914862750022,0.186104771254577,
-0.0766085851661355));
#84835=CARTESIAN_POINT('Ctrl Pts',(-0.0815346538991313,0.216182177401989,
-0.0655240584080556));
#84836=CARTESIAN_POINT('Ctrl Pts',(-0.225717717433852,0.0493277497705959,
-0.0544395316499754));
#84837=CARTESIAN_POINT('Ctrl Pts',(-0.164287302485293,-0.162438194999925,
-0.0433550048918953));
#84838=CARTESIAN_POINT('Ctrl Pts',(0.0467796463453727,-0.226279314006825,
-0.0322704781338153));
#84839=CARTESIAN_POINT('Ctrl Pts',(0.215259778741053,-0.0839253033516204,
-0.0211859513757352));
#84840=CARTESIAN_POINT('Ctrl Pts',(0.187611971177778,0.134729602837997,
-0.0101014246176551));
#84841=CARTESIAN_POINT('Ctrl Pts',(-0.0108400899107792,0.230941269302219,
0.000983102140424831));
#84842=CARTESIAN_POINT('Ctrl Pts',(-0.199604920077247,0.116227920628962,
0.012067628898505));
#84843=CARTESIAN_POINT('Ctrl Pts',(-0.203936515089227,-0.0299908189741295,
0.0194573134038917));
#84844=CARTESIAN_POINT('Ctrl Pts',(-0.174767351138882,-0.087952107769144,
0.0231521556565851));
#84845=CARTESIAN_POINT('Ctrl Pts',(0.00540516581313481,0.195637521218248,
-4.85722573273506E-16));
#84846=CARTESIAN_POINT('Ctrl Pts',(0.000530987028742651,0.195316024296212,
-6.89315582075481E-16));
#84847=CARTESIAN_POINT('Ctrl Pts',(-0.00432231600472944,0.194799753536188,
-6.5733328270164E-16));
#84848=CARTESIAN_POINT('Ctrl Pts',(-0.00914525981218943,0.194083130228181,
-7.73686670285656E-16));
#84849=CARTESIAN_POINT('Ctrl Pts',(-0.0182975460219355,0.192723226011732,
-6.37220818447363E-16));
#84850=CARTESIAN_POINT('Ctrl Pts',(-0.0273404118900563,0.190642703413875,
-4.3456410221573E-16));
#84851=CARTESIAN_POINT('Ctrl Pts',(-0.0362103123303198,0.187887905371836,
-5.72458747072346E-16));
#84852=CARTESIAN_POINT('Ctrl Pts',(-0.0426952759989041,0.185873816787954,
-6.73276311825183E-16));
#84853=CARTESIAN_POINT('Ctrl Pts',(-0.0490889890704407,0.183497301278578,
-5.53257083171345E-16));
#84854=CARTESIAN_POINT('Ctrl Pts',(-0.0553333559413038,0.180788923207186,
-5.62050406216485E-16));
#84855=CARTESIAN_POINT('Ctrl Pts',(-0.0654069179123671,0.176419702931141,
-5.76236005246569E-16));
#84856=CARTESIAN_POINT('Ctrl Pts',(-0.0751114695691119,0.171183241386391,
-3.41160100153046E-16));
#84857=CARTESIAN_POINT('Ctrl Pts',(-0.0843298237574837,0.165151495399874,
-4.68375338513738E-16));
#84858=CARTESIAN_POINT('Ctrl Pts',(-0.0881916390397545,0.162624635577229,
-5.21669206551349E-16));
#84859=CARTESIAN_POINT('Ctrl Pts',(-0.0919679137130864,0.159957413059854,
-6.04042371500311E-16));
#84860=CARTESIAN_POINT('Ctrl Pts',(-0.0956347997707068,0.157166413867924,
-4.8919202022546E-16));
#84861=CARTESIAN_POINT('Ctrl Pts',(-0.104794954097449,0.150194290130738,
-2.02287293537293E-16));
#84862=CARTESIAN_POINT('Ctrl Pts',(-0.113294139529456,0.142440339385748,
-3.10624878440371E-16));
#84863=CARTESIAN_POINT('Ctrl Pts',(-0.120997002971,0.133986645954499,-1.07552855510562E-16));
#84864=CARTESIAN_POINT('Ctrl Pts',(-0.125172453318786,0.12940419717484,
2.52531933996346E-18));
#84865=CARTESIAN_POINT('Ctrl Pts',(-0.129113156531883,0.124615891131193,
-1.51055882874737E-16));
#84866=CARTESIAN_POINT('Ctrl Pts',(-0.132792406759928,0.119633076898729,
9.8879238130678E-17));
#84867=CARTESIAN_POINT('Ctrl Pts',(-0.135556286113385,0.115889950847057,
2.86632306781755E-16));
#84868=CARTESIAN_POINT('Ctrl Pts',(-0.138174807679848,0.112032992900381,
-3.37097310003989E-16));
#84869=CARTESIAN_POINT('Ctrl Pts',(-0.140624206910481,0.108085595299114,
-4.63171168085807E-16));
#84870=CARTESIAN_POINT('Ctrl Pts',(-0.140929371379385,0.107593798993523,
-4.78878391907511E-16));
#84871=CARTESIAN_POINT('Ctrl Pts',(-0.141231895824984,0.107100637144526,
-4.76751570490669E-16));
#84872=CARTESIAN_POINT('Ctrl Pts',(-0.141531732093613,0.106606173963904,
-4.82253126321552E-16));
#84873=CARTESIAN_POINT('Ctrl Pts',(-0.14512786301753,0.100675756197219,
-5.17611903429286E-16));
#84874=CARTESIAN_POINT('Ctrl Pts',(-0.148344736494633,0.094547001960059,
-1.53978557988108E-16));
#84875=CARTESIAN_POINT('Ctrl Pts',(-0.151148162339273,0.0882379718247826,
-1.64798730217797E-16));
#84876=CARTESIAN_POINT('Ctrl Pts',(-0.154328174579003,0.0810814447172957,
1.1508442599124E-16));
#84877=CARTESIAN_POINT('Ctrl Pts',(-0.1569763429285,0.0736927501953974,
9.29594947834426E-17));
#84878=CARTESIAN_POINT('Ctrl Pts',(-0.159093979189513,0.0661295205528138,
-5.3776427755281E-17));
#84879=CARTESIAN_POINT('Ctrl Pts',(-0.160234456452329,0.0620562566029943,
2.41628073730984E-16));
#84880=CARTESIAN_POINT('Ctrl Pts',(-0.161220877544346,0.057932365739095,
2.60879163199896E-17));
#84881=CARTESIAN_POINT('Ctrl Pts',(-0.162052257864859,0.0537670724081219,
8.84708972748172E-17));
#84882=CARTESIAN_POINT('Ctrl Pts',(-0.162804807434059,0.0499967285300273,
1.44938778802232E-16));
#84883=CARTESIAN_POINT('Ctrl Pts',(-0.163429545394715,0.0461947404422942,
-9.50192087901827E-17));
#84884=CARTESIAN_POINT('Ctrl Pts',(-0.163924812172196,0.0423819372460028,
-2.67147415300428E-16));
#84885=CARTESIAN_POINT('Ctrl Pts',(-0.165187320646542,0.0326625363792493,
-7.05927743950919E-16));
#84886=CARTESIAN_POINT('Ctrl Pts',(-0.165615374754996,0.0228510577214756,
2.09168582709701E-16));
#84887=CARTESIAN_POINT('Ctrl Pts',(-0.165212654472542,0.0130612428985379,
1.92554305833426E-16));
#84888=CARTESIAN_POINT('Ctrl Pts',(-0.164960053646113,0.00692071454025313,
1.82133226358855E-16));
#84889=CARTESIAN_POINT('Ctrl Pts',(-0.164380026075269,0.000788975702457714,
-7.40388912887612E-17));
#84890=CARTESIAN_POINT('Ctrl Pts',(-0.163468309056199,-0.00530325479555159,
-1.56125112837913E-17));
#84891=CARTESIAN_POINT('Ctrl Pts',(-0.16264648558514,-0.0107948030606855,
3.70531398039655E-17));
#84892=CARTESIAN_POINT('Ctrl Pts',(-0.161552824018776,-0.0162603049141666,
-7.32136910689234E-17));
#84893=CARTESIAN_POINT('Ctrl Pts',(-0.160193793940068,-0.021636056037818,
-1.15792792021452E-16));
#84894=CARTESIAN_POINT('Ctrl Pts',(-0.157557295101067,-0.0320649360297449,
-1.98395636495481E-16));
#84895=CARTESIAN_POINT('Ctrl Pts',(-0.153922696083113,-0.042186526932804,
6.12453783703427E-16));
#84896=CARTESIAN_POINT('Ctrl Pts',(-0.149273689660746,-0.0518329037170428,
1.85398571495021E-16));
#84897=CARTESIAN_POINT('Ctrl Pts',(-0.146262157372015,-0.0580816314054429,
-9.1239153600102E-17));
#84898=CARTESIAN_POINT('Ctrl Pts',(-0.14282411654673,-0.064130517147505,
8.59534368207069E-17));
#84899=CARTESIAN_POINT('Ctrl Pts',(-0.138946909435068,-0.0699253806456778,
-1.51788304147971E-18));
#84900=CARTESIAN_POINT('Ctrl Pts',(-0.0905532414578939,-0.126782311156848,
-0.9746));
#84901=CARTESIAN_POINT('Ctrl Pts',(-0.0940297960121039,-0.124924866292241,
-0.9746));
#84902=CARTESIAN_POINT('Ctrl Pts',(-0.0974241536190665,-0.122930444609242,
-0.9746));
#84903=CARTESIAN_POINT('Ctrl Pts',(-0.100727224830823,-0.120800921794934,
-0.9746));
#84904=CARTESIAN_POINT('Ctrl Pts',(-0.10828471896806,-0.115928530268235,
-0.9746));
#84905=CARTESIAN_POINT('Ctrl Pts',(-0.115365087206815,-0.110350660277646,
-0.9746));
#84906=CARTESIAN_POINT('Ctrl Pts',(-0.12193959644215,-0.104174135776912,
-0.9746));
#84907=CARTESIAN_POINT('Ctrl Pts',(-0.125553172842108,-0.10077930547541,
-0.9746));
#84908=CARTESIAN_POINT('Ctrl Pts',(-0.129009586137417,-0.0972064788121822,
-0.9746));
#84909=CARTESIAN_POINT('Ctrl Pts',(-0.132294618133166,-0.0934837784148553,
-0.9746));
#84910=CARTESIAN_POINT('Ctrl Pts',(-0.137791783897699,-0.0872542192500508,
-0.9746));
#84911=CARTESIAN_POINT('Ctrl Pts',(-0.142817433677964,-0.0805988103873133,
-0.9746));
#84912=CARTESIAN_POINT('Ctrl Pts',(-0.147349142107892,-0.0735898319648689,
-0.9746));
#84913=CARTESIAN_POINT('Ctrl Pts',(-0.15016186090448,-0.0692395332511452,
-0.9746));
#84914=CARTESIAN_POINT('Ctrl Pts',(-0.152782767435203,-0.0647533954404122,
-0.9746));
#84915=CARTESIAN_POINT('Ctrl Pts',(-0.155194586759511,-0.0601701145151422,
-0.9746));
#84916=CARTESIAN_POINT('Ctrl Pts',(-0.160644212994169,-0.0498139623276951,
-0.9746));
#84917=CARTESIAN_POINT('Ctrl Pts',(-0.165043005663089,-0.0389449931280598,
-0.9746));
#84918=CARTESIAN_POINT('Ctrl Pts',(-0.168323366438074,-0.027755975176349,
-0.9746));
#84919=CARTESIAN_POINT('Ctrl Pts',(-0.169980006434906,-0.0221053239414555,
-0.9746));
#84920=CARTESIAN_POINT('Ctrl Pts',(-0.171350852496603,-0.0163723993947195,
-0.9746));
#84921=CARTESIAN_POINT('Ctrl Pts',(-0.172423067159833,-0.0105792113265366,
-0.9746));
#84922=CARTESIAN_POINT('Ctrl Pts',(-0.173278550653338,-0.00595702424305383,
-0.9746));
#84923=CARTESIAN_POINT('Ctrl Pts',(-0.173942658225041,-0.00129956377914802,
-0.9746));
#84924=CARTESIAN_POINT('Ctrl Pts',(-0.174407751945051,0.00335988535112334,
-0.9746));
#84925=CARTESIAN_POINT('Ctrl Pts',(-0.174995692542755,0.00925005154507497,
-0.9746));
#84926=CARTESIAN_POINT('Ctrl Pts',(-0.175267577699845,0.0151526234854924,
-0.9746));
#84927=CARTESIAN_POINT('Ctrl Pts',(-0.175214225529177,0.0210443329477897,
-0.9746));
#84928=CARTESIAN_POINT('Ctrl Pts',(-0.175144700049102,0.0287220698364688,
-0.9746));
#84929=CARTESIAN_POINT('Ctrl Pts',(-0.174523326685391,0.0363814112077174,
-0.9746));
#84930=CARTESIAN_POINT('Ctrl Pts',(-0.173385196589427,0.0439834824917145,
-0.9746));
#84931=CARTESIAN_POINT('Ctrl Pts',(-0.172591342738426,0.0492859813763208,
-0.9746));
#84932=CARTESIAN_POINT('Ctrl Pts',(-0.171545526366501,0.0545620014471183,
-0.9746));
#84933=CARTESIAN_POINT('Ctrl Pts',(-0.170257892847336,0.0597943370226613,
-0.9746));
#84934=CARTESIAN_POINT('Ctrl Pts',(-0.16917772877666,0.0641836145696469,
-0.9746));
#84935=CARTESIAN_POINT('Ctrl Pts',(-0.167929193511731,0.0685340110951642,
-0.9746));
#84936=CARTESIAN_POINT('Ctrl Pts',(-0.166522756084503,0.0728284761344198,
-0.9746));
#84937=CARTESIAN_POINT('Ctrl Pts',(-0.163087091801193,0.0833190531523973,
-0.9746));
#84938=CARTESIAN_POINT('Ctrl Pts',(-0.158706981261738,0.0934946544278663,
-0.9746));
#84939=CARTESIAN_POINT('Ctrl Pts',(-0.153475389427475,0.103246175515399,
-0.9746));
#84940=CARTESIAN_POINT('Ctrl Pts',(-0.150477503861082,0.108834139034881,
-0.9746));
#84941=CARTESIAN_POINT('Ctrl Pts',(-0.147199377055609,0.114282853508606,
-0.9746));
#84942=CARTESIAN_POINT('Ctrl Pts',(-0.143653574449483,0.119570985860742,
-0.9746));
#84943=CARTESIAN_POINT('Ctrl Pts',(-0.140594184743723,0.124133692665932,
-0.9746));
#84944=CARTESIAN_POINT('Ctrl Pts',(-0.137333362290461,0.128578228872186,
-0.9746));
#84945=CARTESIAN_POINT('Ctrl Pts',(-0.133900829694537,0.132864190726999,
-0.9746));
#84946=CARTESIAN_POINT('Ctrl Pts',(-0.125893219189598,0.142862730351392,
-0.9746));
#84947=CARTESIAN_POINT('Ctrl Pts',(-0.11693274942408,0.152034765661666,
-0.9746));
#84948=CARTESIAN_POINT('Ctrl Pts',(-0.107134319818378,0.160216555670847,
-0.9746));
#84949=CARTESIAN_POINT('Ctrl Pts',(-0.100515704826846,0.165743167606786,
-0.974600000000001));
#84950=CARTESIAN_POINT('Ctrl Pts',(-0.0935136574613262,0.170817815415233,
-0.9746));
#84951=CARTESIAN_POINT('Ctrl Pts',(-0.0861525859670518,0.175382131162754,
-0.9746));
#84952=CARTESIAN_POINT('Origin',(-2.59090492670967E-17,0.,-0.9746));
#84953=CARTESIAN_POINT('',(-0.1954,-2.39295984553393E-17,-0.9746));
#84954=CARTESIAN_POINT('Origin',(0.,0.,-0.9746));
#84955=CARTESIAN_POINT('',(0.089187861459517,0.173858233536057,-0.9746));
#84956=CARTESIAN_POINT('Origin',(0.,0.,-0.9746));
#84957=CARTESIAN_POINT('Ctrl Pts',(0.0891878614595168,0.173858233536056,
-0.9746));
#84958=CARTESIAN_POINT('Ctrl Pts',(0.0923684083710216,0.171824919272554,
-0.9746));
#84959=CARTESIAN_POINT('Ctrl Pts',(0.0954821720660944,0.169694318827644,
-0.9746));
#84960=CARTESIAN_POINT('Ctrl Pts',(0.0985240274780785,0.167466145207355,
-0.9746));
#84961=CARTESIAN_POINT('Ctrl Pts',(0.105746831175391,0.162175406995579,
-0.9746));
#84962=CARTESIAN_POINT('Ctrl Pts',(0.112564936659085,0.156334970325733,
-0.9746));
#84963=CARTESIAN_POINT('Ctrl Pts',(0.118945973249969,0.150010093026968,
-0.9746));
#84964=CARTESIAN_POINT('Ctrl Pts',(0.123811088224797,0.145187795768224,
-0.9746));
#84965=CARTESIAN_POINT('Ctrl Pts',(0.128424432090268,0.140079378982527,
-0.9746));
#84966=CARTESIAN_POINT('Ctrl Pts',(0.132746242480251,0.1347416062205,-0.9746));
#84967=CARTESIAN_POINT('Ctrl Pts',(0.137683220397198,0.128644053603919,
-0.974600000000001));
#84968=CARTESIAN_POINT('Ctrl Pts',(0.142247212696115,0.12224100971048,-0.9746));
#84969=CARTESIAN_POINT('Ctrl Pts',(0.146414335551708,0.115576031346523,
-0.9746));
#84970=CARTESIAN_POINT('Ctrl Pts',(0.148827550732419,0.11171628745982,-0.9746));
#84971=CARTESIAN_POINT('Ctrl Pts',(0.151107538509771,0.107768645316273,
-0.9746));
#84972=CARTESIAN_POINT('Ctrl Pts',(0.153248499385483,0.103741352735909,
-0.9746));
#84973=CARTESIAN_POINT('Ctrl Pts',(0.155301440138075,0.0998796319755569,
-0.9746));
#84974=CARTESIAN_POINT('Ctrl Pts',(0.157222955525038,0.0959510427103076,
-0.9746));
#84975=CARTESIAN_POINT('Ctrl Pts',(0.159005757143888,0.0919709142949633,
-0.9746));
#84976=CARTESIAN_POINT('Ctrl Pts',(0.163158600449716,0.0826996361722365,
-0.9746));
#84977=CARTESIAN_POINT('Ctrl Pts',(0.166567079218136,0.0731365417482814,
-0.9746));
#84978=CARTESIAN_POINT('Ctrl Pts',(0.169173701012897,0.0633765445475195,
-0.9746));
#84979=CARTESIAN_POINT('Ctrl Pts',(0.170831815402072,0.0571680520729268,
-0.9746));
#84980=CARTESIAN_POINT('Ctrl Pts',(0.1721649817233,0.0508798122827543,-0.9746));
#84981=CARTESIAN_POINT('Ctrl Pts',(0.17315298703667,0.0445368070399667,
-0.9746));
#84982=CARTESIAN_POINT('Ctrl Pts',(0.174093136343655,0.0385010378973178,
-0.9746));
#84983=CARTESIAN_POINT('Ctrl Pts',(0.174720282450967,0.0324079620925687,
-0.9746));
#84984=CARTESIAN_POINT('Ctrl Pts',(0.175013450792712,0.0263260434350132,
-0.9746));
#84985=CARTESIAN_POINT('Ctrl Pts',(0.175314120252881,0.0200885104576577,
-0.9746));
#84986=CARTESIAN_POINT('Ctrl Pts',(0.175265697707793,0.0138545067086832,
-0.9746));
#84987=CARTESIAN_POINT('Ctrl Pts',(0.174851965608991,0.00764741813027898,
-0.9746));
#84988=CARTESIAN_POINT('Ctrl Pts',(0.17433114008016,-0.000166358467454291,
-0.9746));
#84989=CARTESIAN_POINT('Ctrl Pts',(0.173231574277968,-0.00793775250040705,
-0.9746));
#84990=CARTESIAN_POINT('Ctrl Pts',(0.171581280878545,-0.0156163834798823,
-0.9746));
#84991=CARTESIAN_POINT('Ctrl Pts',(0.170692439127582,-0.0197520649333607,
-0.9746));
#84992=CARTESIAN_POINT('Ctrl Pts',(0.169643681680851,-0.0238607579522018,
-0.9746));
#84993=CARTESIAN_POINT('Ctrl Pts',(0.168438435903388,-0.027933840546177,
-0.9746));
#84994=CARTESIAN_POINT('Ctrl Pts',(0.167347408280003,-0.0316209272014028,
-0.9746));
#84995=CARTESIAN_POINT('Ctrl Pts',(0.166128520428818,-0.0352764519303832,
-0.9746));
#84996=CARTESIAN_POINT('Ctrl Pts',(0.164790010901572,-0.0388812084305513,
-0.9746));
#84997=CARTESIAN_POINT('Ctrl Pts',(0.16137835252225,-0.04806918764839,-0.9746));
#84998=CARTESIAN_POINT('Ctrl Pts',(0.157185477598737,-0.0569498321473851,
-0.9746));
#84999=CARTESIAN_POINT('Ctrl Pts',(0.152267636060245,-0.0654242188104072,
-0.9746));
#85000=CARTESIAN_POINT('Ctrl Pts',(0.149183032157992,-0.0707395844978447,
-0.9746));
#85001=CARTESIAN_POINT('Ctrl Pts',(0.145812828254551,-0.0758946172057797,
-0.9746));
#85002=CARTESIAN_POINT('Ctrl Pts',(0.142167564876524,-0.0808601523014113,
-0.9746));
#85003=CARTESIAN_POINT('Ctrl Pts',(0.138881773074575,-0.0853360194247216,
-0.9746));
#85004=CARTESIAN_POINT('Ctrl Pts',(0.135367611992976,-0.0896621905227919,
-0.9746));
#85005=CARTESIAN_POINT('Ctrl Pts',(0.131660485192568,-0.0937853191898041,
-0.9746));
#85006=CARTESIAN_POINT('Ctrl Pts',(0.124468401335915,-0.101784475604323,
-0.9746));
#85007=CARTESIAN_POINT('Ctrl Pts',(0.116536365050231,-0.10904667878116,
-0.9746));
#85008=CARTESIAN_POINT('Ctrl Pts',(0.107928190692747,-0.115415747498982,
-0.9746));
#85009=CARTESIAN_POINT('Ctrl Pts',(0.102351941465377,-0.119541536898908,
-0.9746));
#85010=CARTESIAN_POINT('Ctrl Pts',(0.0964914220373157,-0.123291767245807,
-0.9746));
#85011=CARTESIAN_POINT('Ctrl Pts',(0.0903606778650203,-0.126612599672284,
-0.9746));
#85012=CARTESIAN_POINT('Ctrl Pts',(0.113597585008592,-0.159278481118232,
-0.997748074722608));
#85013=CARTESIAN_POINT('Ctrl Pts',(0.16644003092961,-0.121593162196469,
-0.994052057794214));
#85014=CARTESIAN_POINT('Ctrl Pts',(0.230765385058606,0.00981445541203181,
-0.986661198613126));
#85015=CARTESIAN_POINT('Ctrl Pts',(0.117189675071622,0.199275529823258,
-0.975575497179346));
#85016=CARTESIAN_POINT('Ctrl Pts',(-0.103218031716069,0.206613681168277,
-0.964490970421265));
#85017=CARTESIAN_POINT('Ctrl Pts',(-0.229553900654321,0.0260392872026454,
-0.953406443663186));
#85018=CARTESIAN_POINT('Ctrl Pts',(-0.146815211474769,-0.1784061830235,
-0.942321916905106));
#85019=CARTESIAN_POINT('Ctrl Pts',(0.0696715872818821,-0.220261620189527,
-0.931237390147025));
#85020=CARTESIAN_POINT('Ctrl Pts',(0.222687127489829,-0.0615221438598078,
-0.920152863388945));
#85021=CARTESIAN_POINT('Ctrl Pts',(0.172860435250692,0.153279874428372,
-0.909068336630866));
#85022=CARTESIAN_POINT('Ctrl Pts',(-0.034427118799567,0.228447496603342,
-0.897983809872785));
#85023=CARTESIAN_POINT('Ctrl Pts',(-0.210353898174444,0.0955279693800359,
-0.886899283114706));
#85024=CARTESIAN_POINT('Ctrl Pts',(-0.194669526643631,-0.124411313377869,
-0.875814756356625));
#85025=CARTESIAN_POINT('Ctrl Pts',(-0.0016600774612449,-0.231022463164353,
-0.864730229598545));
#85026=CARTESIAN_POINT('Ctrl Pts',(0.192861385988943,-0.127195753155124,
-0.853645702840465));
#85027=CARTESIAN_POINT('Ctrl Pts',(0.211705181679844,0.0924942334409426,
-0.842561176082385));
#85028=CARTESIAN_POINT('Ctrl Pts',(0.0377063431658909,0.227930832056205,
-0.831476649324304));
#85029=CARTESIAN_POINT('Ctrl Pts',(-0.170639242107946,0.155744994213846,
-0.820392122566225));
#85030=CARTESIAN_POINT('Ctrl Pts',(-0.223549277689542,-0.0583092770165013,
-0.809307595808144));
#85031=CARTESIAN_POINT('Ctrl Pts',(-0.0728279089482567,-0.219249498669582,
-0.798223069050065));
#85032=CARTESIAN_POINT('Ctrl Pts',(0.144232516508625,-0.18047501610888,
-0.787138542291984));
#85033=CARTESIAN_POINT('Ctrl Pts',(0.229911311338269,0.0226944598360864,
-0.776054015533904));
#85034=CARTESIAN_POINT('Ctrl Pts',(0.106163520338706,0.205191510592405,
-0.764969488775825));
#85035=CARTESIAN_POINT('Ctrl Pts',(-0.114288792391887,0.200779285496967,
-0.753884962017745));
#85036=CARTESIAN_POINT('Ctrl Pts',(-0.230635259730438,0.0134768834665719,
-0.742800435259663));
#85037=CARTESIAN_POINT('Ctrl Pts',(-0.136895696235943,-0.186101632754491,
-0.731715908501585));
#85038=CARTESIAN_POINT('Ctrl Pts',(0.0815423780626619,-0.216159871416477,
-0.720631381743503));
#85039=CARTESIAN_POINT('Ctrl Pts',(0.225703368478632,-0.0493177337732571,
-0.709546854985425));
#85040=CARTESIAN_POINT('Ctrl Pts',(0.164270795880326,0.162448007136189,
-0.698462328227344));
#85041=CARTESIAN_POINT('Ctrl Pts',(-0.0467963100731284,0.226239595948386,
-0.687377801469264));
#85042=CARTESIAN_POINT('Ctrl Pts',(-0.215236581581508,0.0839491712670712,
-0.676293274711184));
#85043=CARTESIAN_POINT('Ctrl Pts',(-0.187617503186297,-0.134810689135161,
-0.665208747953103));
#85044=CARTESIAN_POINT('Ctrl Pts',(0.0109026619765615,-0.230771275010779,
-0.654124221195024));
#85045=CARTESIAN_POINT('Ctrl Pts',(0.199491574731264,-0.116521933638534,
-0.643039694436944));
#85046=CARTESIAN_POINT('Ctrl Pts',(0.206363289762344,0.103867425336797,
-0.631955167678864));
#85047=CARTESIAN_POINT('Ctrl Pts',(0.0252583507465755,0.229643778764786,
-0.620870640920783));
#85048=CARTESIAN_POINT('Ctrl Pts',(-0.178854460771993,0.1462372431006,-0.609786114162703));
#85049=CARTESIAN_POINT('Ctrl Pts',(-0.220048455014294,-0.0703770335659106,
-0.598701587404623));
#85050=CARTESIAN_POINT('Ctrl Pts',(-0.0607999560716834,-0.222884756655582,
-0.587617060646543));
#85051=CARTESIAN_POINT('Ctrl Pts',(0.153831321085638,-0.17236639481282,
-0.576532533888463));
#85052=CARTESIAN_POINT('Ctrl Pts',(0.228337399334668,0.0351607945417151,
-0.565448007130383));
#85053=CARTESIAN_POINT('Ctrl Pts',(0.0948505716256339,0.210659959342106,
-0.554363480372303));
#85054=CARTESIAN_POINT('Ctrl Pts',(-0.125035795018697,0.194268626833483,
-0.543278953614223));
#85055=CARTESIAN_POINT('Ctrl Pts',(-0.23102685397145,0.000917688279968637,
-0.532194426856142));
#85056=CARTESIAN_POINT('Ctrl Pts',(-0.126575178392383,-0.193269174010399,
-0.521109900098063));
#85057=CARTESIAN_POINT('Ctrl Pts',(0.0931740316803935,-0.211406833447139,
-0.510025373339982));
#85058=CARTESIAN_POINT('Ctrl Pts',(0.228050865762629,-0.0369736667459479,
-0.498940846581903));
#85059=CARTESIAN_POINT('Ctrl Pts',(0.155195797780493,0.171138872729142,
-0.487856319823823));
#85060=CARTESIAN_POINT('Ctrl Pts',(-0.0590273731357318,0.223360736541632,
-0.476771793065742));
#85061=CARTESIAN_POINT('Ctrl Pts',(-0.219482414497422,0.0721229445745739,
-0.465687266307662));
#85062=CARTESIAN_POINT('Ctrl Pts',(-0.18001056989549,-0.14481175412799,
-0.454602739549582));
#85063=CARTESIAN_POINT('Ctrl Pts',(0.0234331936510666,-0.229837192036099,
-0.443518212791502));
#85064=CARTESIAN_POINT('Ctrl Pts',(0.205531623241974,-0.105503560391314,
-0.432433686033422));
#85065=CARTESIAN_POINT('Ctrl Pts',(0.200410965162878,0.11493343486647,-0.421349159275342));
#85066=CARTESIAN_POINT('Ctrl Pts',(0.0127356351310226,0.230677378616861,
-0.410264632517262));
#85067=CARTESIAN_POINT('Ctrl Pts',(-0.18654060551751,0.136296925500451,
-0.399180105759182));
#85068=CARTESIAN_POINT('Ctrl Pts',(-0.215896707223304,-0.0822366172567873,
-0.388095579001102));
#85069=CARTESIAN_POINT('Ctrl Pts',(-0.0485921495146213,-0.225860692492862,
-0.377011052243022));
#85070=CARTESIAN_POINT('Ctrl Pts',(0.162975075692969,-0.163747898033848,
-0.365926525484941));
#85071=CARTESIAN_POINT('Ctrl Pts',(0.226088041147545,0.0475231212957209,
-0.354841998726862));
#85072=CARTESIAN_POINT('Ctrl Pts',(0.0832570446511227,0.215505252660433,
-0.343757471968781));
#85073=CARTESIAN_POINT('Ctrl Pts',(-0.135412928329534,0.187183301200128,
-0.332672945210701));
#85074=CARTESIAN_POINT('Ctrl Pts',(-0.230735046119166,-0.0116442217304382,
-0.321588418452622));
#85075=CARTESIAN_POINT('Ctrl Pts',(-0.115880237623372,-0.199865004289646,
-0.310503891694541));
#85076=CARTESIAN_POINT('Ctrl Pts',(0.104530066545176,-0.206028431508216,
-0.299419364936461));
#85077=CARTESIAN_POINT('Ctrl Pts',(0.229723764209575,-0.0245202276603256,
-0.288334838178381));
#85078=CARTESIAN_POINT('Ctrl Pts',(0.145661713927447,0.179323491284942,
-0.277250311420301));
#85079=CARTESIAN_POINT('Ctrl Pts',(-0.0710838269339852,0.219821152099225,
-0.266165784662221));
#85080=CARTESIAN_POINT('Ctrl Pts',(-0.2230789949398,0.0600833707072694,
-0.255081257904141));
#85081=CARTESIAN_POINT('Ctrl Pts',(-0.171871146156301,-0.154384450868564,
-0.243996731146061));
#85082=CARTESIAN_POINT('Ctrl Pts',(0.0358944075470365,-0.228223225322811,
-0.232912204387981));
#85083=CARTESIAN_POINT('Ctrl Pts',(0.210963687025698,-0.0941730977777479,
-0.2218276776299));
#85084=CARTESIAN_POINT('Ctrl Pts',(0.193865803917006,0.125659461758854,
-0.21074315087182));
#85085=CARTESIAN_POINT('Ctrl Pts',(0.000175245362767064,0.23102860489061,
-0.199658624113741));
#85086=CARTESIAN_POINT('Ctrl Pts',(-0.193674941721658,0.125953436994848,
-0.18857409735566));
#85087=CARTESIAN_POINT('Ctrl Pts',(-0.211106316733187,-0.0938529552288718,
-0.17748957059758));
#85088=CARTESIAN_POINT('Ctrl Pts',(-0.0362405967794985,-0.228168472103057,
-0.1664050438395));
#85089=CARTESIAN_POINT('Ctrl Pts',(0.171636722311097,-0.154645086324223,
-0.15532051708142));
#85090=CARTESIAN_POINT('Ctrl Pts',(0.223169909972479,0.0597450007042502,
-0.14423599032334));
#85091=CARTESIAN_POINT('Ctrl Pts',(0.0714171971037106,0.219712808687961,
-0.13315146356526));
#85092=CARTESIAN_POINT('Ctrl Pts',(-0.145389424622739,0.179544742913656,
-0.12206693680718));
#85093=CARTESIAN_POINT('Ctrl Pts',(-0.229760834740975,-0.0241725925417204,
-0.1109824100491));
#85094=CARTESIAN_POINT('Ctrl Pts',(-0.10484225286162,-0.205867887802041,
-0.0998978832910191));
#85095=CARTESIAN_POINT('Ctrl Pts',(0.115576399225017,-0.20004385999579,
-0.0888133565329394));
#85096=CARTESIAN_POINT('Ctrl Pts',(0.230718050422665,-0.0119879999976286,
-0.0777288297748591));
#85097=CARTESIAN_POINT('Ctrl Pts',(0.135694965983318,0.186965739133346,
-0.0666443030167789));
#85098=CARTESIAN_POINT('Ctrl Pts',(-0.0829266138056062,0.215654003403905,
-0.055559776258699));
#85099=CARTESIAN_POINT('Ctrl Pts',(-0.22602215760672,0.0478228193903156,
-0.0444752495006188));
#85100=CARTESIAN_POINT('Ctrl Pts',(-0.163210881612501,-0.163417818613872,
-0.0333907227425388));
#85101=CARTESIAN_POINT('Ctrl Pts',(0.0482249176056553,-0.226094038071907,
-0.0223061959844587));
#85102=CARTESIAN_POINT('Ctrl Pts',(0.215825725144946,-0.0822379657419614,
-0.0112216692263785));
#85103=CARTESIAN_POINT('Ctrl Pts',(0.196338036420179,0.0627312190287936,
-0.00383198472099195));
#85104=CARTESIAN_POINT('Ctrl Pts',(0.158139484186755,0.115177904597422,
-0.000137142468298633));
#85105=CARTESIAN_POINT('Ctrl Pts',(0.105785576840747,-0.148325037034332,
-0.989980505168611));
#85106=CARTESIAN_POINT('Ctrl Pts',(0.154994093227852,-0.113231305065781,
-0.986284488240217));
#85107=CARTESIAN_POINT('Ctrl Pts',(0.214895848106765,0.00913952375890018,
-0.978893629059131));
#85108=CARTESIAN_POINT('Ctrl Pts',(0.109130641961213,0.185571523118247,
-0.967807927625349));
#85109=CARTESIAN_POINT('Ctrl Pts',(-0.0961198164963202,0.192405036109906,
-0.956723400867269));
#85110=CARTESIAN_POINT('Ctrl Pts',(-0.213767676442455,0.0242485878290922,
-0.945638874109188));
#85111=CARTESIAN_POINT('Ctrl Pts',(-0.136718855719335,-0.16613734333938,
-0.93455434735111));
#85112=CARTESIAN_POINT('Ctrl Pts',(0.064880332178426,-0.205114418109014,
-0.923469820593028));
#85113=CARTESIAN_POINT('Ctrl Pts',(0.207373125359477,-0.0572913189677125,
-0.91238529383495));
#85114=CARTESIAN_POINT('Ctrl Pts',(0.16097297186867,0.142738949364604,-0.901300767076867));
#85115=CARTESIAN_POINT('Ctrl Pts',(-0.0320595954650073,0.212737358845976,
-0.89021624031879));
#85116=CARTESIAN_POINT('Ctrl Pts',(-0.195888041611099,0.0889585931296678,
-0.879131713560708));
#85117=CARTESIAN_POINT('Ctrl Pts',(-0.181282270813716,-0.115855654415518,
-0.868047186802629));
#85118=CARTESIAN_POINT('Ctrl Pts',(-0.00154591536276689,-0.215135247172401,
-0.856962660044548));
#85119=CARTESIAN_POINT('Ctrl Pts',(0.179598474435907,-0.118448610665361,
-0.845878133286468));
#85120=CARTESIAN_POINT('Ctrl Pts',(0.19714639851264,0.086133484600512,-0.834793606528389));
#85121=CARTESIAN_POINT('Ctrl Pts',(0.0351133103935012,0.212256224875146,
-0.823709079770307));
#85122=CARTESIAN_POINT('Ctrl Pts',(-0.158904528266968,0.145034544983717,
-0.812624553012229));
#85123=CARTESIAN_POINT('Ctrl Pts',(-0.208175986231854,-0.0542993982124802,
-0.801540026254147));
#85124=CARTESIAN_POINT('Ctrl Pts',(-0.0678195963198858,-0.204171899315044,
-0.790455499496069));
#85125=CARTESIAN_POINT('Ctrl Pts',(0.134313770463549,-0.168063904553753,
-0.779370972737988));
#85126=CARTESIAN_POINT('Ctrl Pts',(0.214100508301226,0.0211337813622365,
-0.768286445979907));
#85127=CARTESIAN_POINT('Ctrl Pts',(0.098862746401033,0.191080666980729,
-0.757201919221828));
#85128=CARTESIAN_POINT('Ctrl Pts',(-0.106429250487093,0.186971866808289,
-0.746117392463747));
#85129=CARTESIAN_POINT('Ctrl Pts',(-0.21477467138544,0.0125500897877264,
-0.735032865705668));
#85130=CARTESIAN_POINT('Ctrl Pts',(-0.127481497007524,-0.173303583614474,
-0.723948338947588));
#85131=CARTESIAN_POINT('Ctrl Pts',(0.0759347788922858,-0.201294743069443,
-0.712863812189507));
#85132=CARTESIAN_POINT('Ctrl Pts',(0.21018194205102,-0.045926195660653,
-0.701779285431428));
#85133=CARTESIAN_POINT('Ctrl Pts',(0.152974034606232,0.151276597475482,
-0.690694758673347));
#85134=CARTESIAN_POINT('Ctrl Pts',(-0.0435781680986445,0.210681293619115,
-0.679610231915267));
#85135=CARTESIAN_POINT('Ctrl Pts',(-0.200434947081913,0.0781760589991238,
-0.668525705157188));
#85136=CARTESIAN_POINT('Ctrl Pts',(-0.174715208941123,-0.125539874050871,
-0.657441178399106));
#85137=CARTESIAN_POINT('Ctrl Pts',(0.0101528952944126,-0.214901333011996,
-0.646356651641028));
#85138=CARTESIAN_POINT('Ctrl Pts',(0.18577271080384,-0.108508820531872,
-0.635272124882946));
#85139=CARTESIAN_POINT('Ctrl Pts',(0.192171863905492,0.0967245518765679,
-0.624187598124867));
#85140=CARTESIAN_POINT('Ctrl Pts',(0.0235213557010934,0.213851373712605,
-0.613103071366787));
#85141=CARTESIAN_POINT('Ctrl Pts',(-0.166554793412863,0.136180633732903,
-0.602018544608706));
#85142=CARTESIAN_POINT('Ctrl Pts',(-0.204915912119448,-0.065537265528554,
-0.590934017850627));
#85143=CARTESIAN_POINT('Ctrl Pts',(-0.056618795412319,-0.207557163737565,
-0.579849491092546));
#85144=CARTESIAN_POINT('Ctrl Pts',(0.143252473509781,-0.160512906166578,
-0.568764964334467));
#85145=CARTESIAN_POINT('Ctrl Pts',(0.212634832871727,0.0327428169577119,
-0.557680437576386));
#85146=CARTESIAN_POINT('Ctrl Pts',(0.0883277794359205,0.196173055215632,
-0.546595910818307));
#85147=CARTESIAN_POINT('Ctrl Pts',(-0.116437190991286,0.180908940538528,
-0.535511384060226));
#85148=CARTESIAN_POINT('Ctrl Pts',(-0.215139336027473,0.000854579646644794,
-0.524426857302147));
#85149=CARTESIAN_POINT('Ctrl Pts',(-0.117870712295035,-0.179978219226038,
-0.513342330544065));
#85150=CARTESIAN_POINT('Ctrl Pts',(0.0867665337000174,-0.196868567431163,
-0.502257803785986));
#85151=CARTESIAN_POINT('Ctrl Pts',(0.21236800396687,-0.0344310195004734,
-0.491173277027906));
#85152=CARTESIAN_POINT('Ctrl Pts',(0.144523116316493,0.159369799720287,
-0.480088750269826));
#85153=CARTESIAN_POINT('Ctrl Pts',(-0.0549681114795289,0.208000410896443,
-0.469004223511746));
#85154=CARTESIAN_POINT('Ctrl Pts',(-0.204388797721832,0.0671631117395441,
-0.457919696753665));
#85155=CARTESIAN_POINT('Ctrl Pts',(-0.167631397906793,-0.134853174410277,
-0.446835169995586));
#85156=CARTESIAN_POINT('Ctrl Pts',(0.0218217130884572,-0.214031486119685,
-0.435750643237505));
#85157=CARTESIAN_POINT('Ctrl Pts',(0.191397390376061,-0.0982481713313137,
-0.424666116479425));
#85158=CARTESIAN_POINT('Ctrl Pts',(0.186628875546626,0.107029561453428,
-0.413581589721345));
#85159=CARTESIAN_POINT('Ctrl Pts',(0.0118598164623526,0.214813893792287,
-0.402497062963266));
#85160=CARTESIAN_POINT('Ctrl Pts',(-0.173712368598325,0.126923903220257,
-0.391412536205185));
#85161=CARTESIAN_POINT('Ctrl Pts',(-0.201049676451375,-0.0765812758544393,
-0.380328009447106));
#85162=CARTESIAN_POINT('Ctrl Pts',(-0.0452505092071028,-0.210328447028174,
-0.369243482689025));
#85163=CARTESIAN_POINT('Ctrl Pts',(0.151767419981167,-0.152487095994691,
-0.358158955930945));
#85164=CARTESIAN_POINT('Ctrl Pts',(0.210540161111511,0.0442549971388958,
-0.347074429172865));
#85165=CARTESIAN_POINT('Ctrl Pts',(0.0775315293349641,0.200685141881938,
-0.335989902414785));
#85166=CARTESIAN_POINT('Ctrl Pts',(-0.126100697774086,0.174310866651902,
-0.324905375656704));
#85167=CARTESIAN_POINT('Ctrl Pts',(-0.214867595550083,-0.0108434586221435,
-0.313820848898625));
#85168=CARTESIAN_POINT('Ctrl Pts',(-0.10791125339948,-0.186120459932837,
-0.302736322140544));
#85169=CARTESIAN_POINT('Ctrl Pts',(0.0973416238192642,-0.191860033565348,
-0.291651795382465));
#85170=CARTESIAN_POINT('Ctrl Pts',(0.213925858627184,-0.0228339927043137,
-0.280567268624384));
#85171=CARTESIAN_POINT('Ctrl Pts',(0.135644683205733,0.166991569101047,
-0.269482741866305));
#85172=CARTESIAN_POINT('Ctrl Pts',(-0.0661954533249173,0.204704240630249,
-0.258398215108224));
#85173=CARTESIAN_POINT('Ctrl Pts',(-0.207738044422124,0.0559514890067786,
-0.247313688350144));
#85174=CARTESIAN_POINT('Ctrl Pts',(-0.160051715333997,-0.143767565033517,
-0.236229161592064));
#85175=CARTESIAN_POINT('Ctrl Pts',(0.0334259800279473,-0.212528510508417,
-0.225144634833984));
#85176=CARTESIAN_POINT('Ctrl Pts',(0.196455895807788,-0.0876968948815729,
-0.214060108075904));
#85177=CARTESIAN_POINT('Ctrl Pts',(0.180533819407379,0.117017968706402,
-0.202975581317824));
#85178=CARTESIAN_POINT('Ctrl Pts',(0.000163193889970841,0.215140966537429,
-0.191891054559744));
#85179=CARTESIAN_POINT('Ctrl Pts',(-0.180356082640966,0.117291727518387,
-0.180806527801664));
#85180=CARTESIAN_POINT('Ctrl Pts',(-0.196588716993028,-0.0873987682602953,
-0.169722001043584));
#85181=CARTESIAN_POINT('Ctrl Pts',(-0.033748362124794,-0.21247752262047,
-0.158637474285504));
#85182=CARTESIAN_POINT('Ctrl Pts',(0.159833412614901,-0.144010276813171,
-0.147552947527423));
#85183=CARTESIAN_POINT('Ctrl Pts',(0.207822707306238,0.0556363884176943,
-0.136468420769343));
#85184=CARTESIAN_POINT('Ctrl Pts',(0.0665058979149409,0.204603347902146,
-0.125383894011263));
#85185=CARTESIAN_POINT('Ctrl Pts',(-0.135391119002199,0.167197605445644,
-0.114299367253183));
#85186=CARTESIAN_POINT('Ctrl Pts',(-0.21396037985004,-0.0225102641536699,
-0.103214840495103));
#85187=CARTESIAN_POINT('Ctrl Pts',(-0.0976323413513673,-0.191710530311696,
-0.0921303137370228));
#85188=CARTESIAN_POINT('Ctrl Pts',(0.107628309706322,-0.186287015885978,
-0.0810457869789431));
#85189=CARTESIAN_POINT('Ctrl Pts',(0.214851768633005,-0.0111635955537256,
-0.0699612602208629));
#85190=CARTESIAN_POINT('Ctrl Pts',(0.126363339941118,0.174108266141238,
-0.0588767334627826));
#85191=CARTESIAN_POINT('Ctrl Pts',(-0.0772238219343526,0.200823663164785,
-0.0477922067047027));
#85192=CARTESIAN_POINT('Ctrl Pts',(-0.210478808325096,0.0445340852534203,
-0.0367076799466226));
#85193=CARTESIAN_POINT('Ctrl Pts',(-0.151987009730526,-0.152179715852388,
-0.0256231531885425));
#85194=CARTESIAN_POINT('Ctrl Pts',(0.0449085315205072,-0.210545745632544,
-0.0145386264304624));
#85195=CARTESIAN_POINT('Ctrl Pts',(0.200983575749465,-0.0765825316054464,
-0.00345409967238224));
#85196=CARTESIAN_POINT('Ctrl Pts',(0.182836038608719,0.0584172470777646,
0.00393558483300434));
#85197=CARTESIAN_POINT('Ctrl Pts',(0.147264367941702,0.107257219211354,
0.00763042708569767));
#85198=CARTESIAN_POINT('Ctrl Pts',(0.0979735686729031,-0.137371592950432,
-0.982212935614615));
#85199=CARTESIAN_POINT('Ctrl Pts',(0.143548155526095,-0.104869447935093,
-0.978516918686221));
#85200=CARTESIAN_POINT('Ctrl Pts',(0.199026311154924,0.00846459210576822,
-0.971126059505134));
#85201=CARTESIAN_POINT('Ctrl Pts',(0.101071608850804,0.171867516413235,
-0.960040358071353));
#85202=CARTESIAN_POINT('Ctrl Pts',(-0.0890216012765712,0.178196391051536,
-0.948955831313273));
#85203=CARTESIAN_POINT('Ctrl Pts',(-0.197981452230588,0.0224578884555389,
-0.937871304555193));
#85204=CARTESIAN_POINT('Ctrl Pts',(-0.126622499963902,-0.153868503655261,
-0.926786777797113));
#85205=CARTESIAN_POINT('Ctrl Pts',(0.0600890770749705,-0.189967216028501,
-0.915702251039033));
#85206=CARTESIAN_POINT('Ctrl Pts',(0.192059123229125,-0.0530604940756169,
-0.904617724280951));
#85207=CARTESIAN_POINT('Ctrl Pts',(0.149085508486649,0.132198024300836,
-0.893533197522875));
#85208=CARTESIAN_POINT('Ctrl Pts',(-0.0296920721304479,0.197027221088611,
-0.882448670764791));
#85209=CARTESIAN_POINT('Ctrl Pts',(-0.181422185047754,0.0823892168792999,
-0.871364144006712));
#85210=CARTESIAN_POINT('Ctrl Pts',(-0.1678950149838,-0.107299995453168,
-0.860279617248632));
#85211=CARTESIAN_POINT('Ctrl Pts',(-0.00143175326428869,-0.19924803118045,
-0.849195090490551));
#85212=CARTESIAN_POINT('Ctrl Pts',(0.16633556288287,-0.109701468175598,
-0.838110563732473));
#85213=CARTESIAN_POINT('Ctrl Pts',(0.182587615345437,0.0797727357600818,
-0.827026036974391));
#85214=CARTESIAN_POINT('Ctrl Pts',(0.0325202776211112,0.196581617694085,
-0.815941510216311));
#85215=CARTESIAN_POINT('Ctrl Pts',(-0.147169814425989,0.13432409575359,
-0.804856983458232));
#85216=CARTESIAN_POINT('Ctrl Pts',(-0.192802694774166,-0.0502895194084593,
-0.793772456700151));
#85217=CARTESIAN_POINT('Ctrl Pts',(-0.062811283691515,-0.189094299960506,
-0.782687929942072));
#85218=CARTESIAN_POINT('Ctrl Pts',(0.124395024418474,-0.155652792998626,
-0.771603403183991));
#85219=CARTESIAN_POINT('Ctrl Pts',(0.198289705264184,0.0195731028883869,
-0.760518876425912));
#85220=CARTESIAN_POINT('Ctrl Pts',(0.0915619724633603,0.176969823369053,
-0.749434349667831));
#85221=CARTESIAN_POINT('Ctrl Pts',(-0.0985697085822984,0.17316444811961,
-0.738349822909751));
#85222=CARTESIAN_POINT('Ctrl Pts',(-0.198914083040442,0.011623296108881,
-0.727265296151671));
#85223=CARTESIAN_POINT('Ctrl Pts',(-0.118067297779106,-0.160505534474456,
-0.716180769393592));
#85224=CARTESIAN_POINT('Ctrl Pts',(0.0703271797219096,-0.186429614722409,
-0.705096242635511));
#85225=CARTESIAN_POINT('Ctrl Pts',(0.194660515623409,-0.0425346575480492,
-0.694011715877431));
#85226=CARTESIAN_POINT('Ctrl Pts',(0.141677273332138,0.140105187814775,
-0.682927189119351));
#85227=CARTESIAN_POINT('Ctrl Pts',(-0.0403600261241604,0.195122991289844,
-0.67184266236127));
#85228=CARTESIAN_POINT('Ctrl Pts',(-0.185633312582319,0.0724029467311765,
-0.660758135603191));
#85229=CARTESIAN_POINT('Ctrl Pts',(-0.161812914695948,-0.116269058966581,
-0.64967360884511));
#85230=CARTESIAN_POINT('Ctrl Pts',(0.00940312861226361,-0.199031391013213,
-0.638589082087031));
#85231=CARTESIAN_POINT('Ctrl Pts',(0.172053846876416,-0.100495707425211,
-0.62750455532895));
#85232=CARTESIAN_POINT('Ctrl Pts',(0.17798043804864,0.089581678416339,-0.616420028570871));
#85233=CARTESIAN_POINT('Ctrl Pts',(0.0217843606556112,0.198058968660423,
-0.60533550181279));
#85234=CARTESIAN_POINT('Ctrl Pts',(-0.154255126053732,0.126124024365207,
-0.59425097505471));
#85235=CARTESIAN_POINT('Ctrl Pts',(-0.189783369224603,-0.0606974974911975,
-0.58316644829663));
#85236=CARTESIAN_POINT('Ctrl Pts',(-0.0524376347529544,-0.192229570819549,
-0.57208192153855));
#85237=CARTESIAN_POINT('Ctrl Pts',(0.132673625933925,-0.148659417520336,
-0.56099739478047));
#85238=CARTESIAN_POINT('Ctrl Pts',(0.196932266408787,0.0303248393737088,
-0.54991286802239));
#85239=CARTESIAN_POINT('Ctrl Pts',(0.0818049872462071,0.181686151089158,
-0.53882834126431));
#85240=CARTESIAN_POINT('Ctrl Pts',(-0.107838586963876,0.167549254243574,
-0.52774381450623));
#85241=CARTESIAN_POINT('Ctrl Pts',(-0.199251818083495,0.000791471013320985,
-0.51665928774815));
#85242=CARTESIAN_POINT('Ctrl Pts',(-0.109166246197688,-0.166687264441677,
-0.50557476099007));
#85243=CARTESIAN_POINT('Ctrl Pts',(0.0803590357196412,-0.182330301415187,
-0.494490234231989));
#85244=CARTESIAN_POINT('Ctrl Pts',(0.196685142171111,-0.0318883722549989,
-0.48340570747391));
#85245=CARTESIAN_POINT('Ctrl Pts',(0.133850434852491,0.147600726711432,
-0.472321180715829));
#85246=CARTESIAN_POINT('Ctrl Pts',(-0.0509088498233257,0.192640085251252,
-0.461236653957749));
#85247=CARTESIAN_POINT('Ctrl Pts',(-0.189295180946243,0.0622032789045141,
-0.450152127199669));
#85248=CARTESIAN_POINT('Ctrl Pts',(-0.155252225918095,-0.124894594692565,
-0.439067600441589));
#85249=CARTESIAN_POINT('Ctrl Pts',(0.020210232525848,-0.198225780203272,
-0.427983073683509));
#85250=CARTESIAN_POINT('Ctrl Pts',(0.17726315751015,-0.0909927822713134,
-0.416898546925429));
#85251=CARTESIAN_POINT('Ctrl Pts',(0.172846785930375,0.0991256880403857,
-0.405814020167349));
#85252=CARTESIAN_POINT('Ctrl Pts',(0.0109839977936825,0.198950408967714,
-0.394729493409269));
#85253=CARTESIAN_POINT('Ctrl Pts',(-0.16088413167914,0.117550880940063,
-0.383644966651188));
#85254=CARTESIAN_POINT('Ctrl Pts',(-0.186202645679447,-0.0709259344520911,
-0.372560439893108));
#85255=CARTESIAN_POINT('Ctrl Pts',(-0.0419088688995842,-0.194796201563484,
-0.361475913135029));
#85256=CARTESIAN_POINT('Ctrl Pts',(0.140559764269364,-0.141226293955535,
-0.350391386376948));
#85257=CARTESIAN_POINT('Ctrl Pts',(0.194992281075478,0.0409868729820711,
-0.339306859618868));
#85258=CARTESIAN_POINT('Ctrl Pts',(0.0718060140188057,0.185865031103444,
-0.328222332860789));
#85259=CARTESIAN_POINT('Ctrl Pts',(-0.116788467218639,0.161438432103676,
-0.317137806102708));
#85260=CARTESIAN_POINT('Ctrl Pts',(-0.199000144981,-0.0100426955138486,
-0.306053279344628));
#85261=CARTESIAN_POINT('Ctrl Pts',(-0.0999422691755887,-0.172375915576028,
-0.294968752586547));
#85262=CARTESIAN_POINT('Ctrl Pts',(0.0901531810933522,-0.177691635622479,
-0.283884225828468));
#85263=CARTESIAN_POINT('Ctrl Pts',(0.198127953044795,-0.0211477577483022,
-0.272799699070387));
#85264=CARTESIAN_POINT('Ctrl Pts',(0.125627652484019,0.154659646917152,
-0.261715172312308));
#85265=CARTESIAN_POINT('Ctrl Pts',(-0.0613070797158493,0.189587329161274,
-0.250630645554227));
#85266=CARTESIAN_POINT('Ctrl Pts',(-0.192397093904447,0.0518196073062874,
-0.239546118796148));
#85267=CARTESIAN_POINT('Ctrl Pts',(-0.148232284511692,-0.133150679198468,
-0.228461592038067));
#85268=CARTESIAN_POINT('Ctrl Pts',(0.030957552508858,-0.196833795694023,
-0.217377065279988));
#85269=CARTESIAN_POINT('Ctrl Pts',(0.181948104589878,-0.0812206919853976,
-0.206292538521907));
#85270=CARTESIAN_POINT('Ctrl Pts',(0.167201834897751,0.10837647565395,-0.195208011763827));
#85271=CARTESIAN_POINT('Ctrl Pts',(0.00015114241717486,0.199253328184248,
-0.184123485005747));
#85272=CARTESIAN_POINT('Ctrl Pts',(-0.167037223560273,0.108630018041926,
-0.173038958247667));
#85273=CARTESIAN_POINT('Ctrl Pts',(-0.18207111725287,-0.0809445812917186,
-0.161954431489587));
#85274=CARTESIAN_POINT('Ctrl Pts',(-0.0312561274700897,-0.196786573137883,
-0.150869904731507));
#85275=CARTESIAN_POINT('Ctrl Pts',(0.148030102918704,-0.133375467302118,
-0.139785377973427));
#85276=CARTESIAN_POINT('Ctrl Pts',(0.192475504639999,0.0515277761311382,
-0.128700851215347));
#85277=CARTESIAN_POINT('Ctrl Pts',(0.0615945987261712,0.189493887116332,
-0.117616324457267));
#85278=CARTESIAN_POINT('Ctrl Pts',(-0.125392813381662,0.154850467977633,
-0.106531797699187));
#85279=CARTESIAN_POINT('Ctrl Pts',(-0.198159924959106,-0.0208479357656191,
-0.0954472709411068));
#85280=CARTESIAN_POINT('Ctrl Pts',(-0.0904224298411148,-0.177553172821352,
-0.0843627441830265));
#85281=CARTESIAN_POINT('Ctrl Pts',(0.0996802201876276,-0.172530171776165,
-0.0732782174249468));
#85282=CARTESIAN_POINT('Ctrl Pts',(0.198985486843346,-0.0103391911098226,
-0.0621936906668666));
#85283=CARTESIAN_POINT('Ctrl Pts',(0.117031713898918,0.161250793149128,
-0.0511091639087864));
#85284=CARTESIAN_POINT('Ctrl Pts',(-0.0715210300630994,0.185993322925665,
-0.0400246371507064));
#85285=CARTESIAN_POINT('Ctrl Pts',(-0.194935459043471,0.0412453511165247,
-0.0289401103926264));
#85286=CARTESIAN_POINT('Ctrl Pts',(-0.140763137848552,-0.140941613090905,
-0.0178555836345462));
#85287=CARTESIAN_POINT('Ctrl Pts',(0.0415921454353594,-0.194997453193184,
-0.00677105687646613));
#85288=CARTESIAN_POINT('Ctrl Pts',(0.186141426353985,-0.0709270974689309,
0.00431346988161405));
#85289=CARTESIAN_POINT('Ctrl Pts',(0.16933404079726,0.0541032751267355,
0.0117031543870006));
#85290=CARTESIAN_POINT('Ctrl Pts',(0.136389251696648,0.0993365338252848,
0.0153979966396939));
#85291=CARTESIAN_POINT('Ctrl Pts',(0.0901615605050589,-0.126418148866534,
-0.974445366060619));
#85292=CARTESIAN_POINT('Ctrl Pts',(0.132102217824338,-0.0965075908044056,
-0.970749349132225));
#85293=CARTESIAN_POINT('Ctrl Pts',(0.183156774203084,0.00778966045263656,
-0.963358489951137));
#85294=CARTESIAN_POINT('Ctrl Pts',(0.0930125757403958,0.158163509708224,
-0.952272788517358));
#85295=CARTESIAN_POINT('Ctrl Pts',(-0.0819233860568225,0.163987745993166,
-0.941188261759276));
#85296=CARTESIAN_POINT('Ctrl Pts',(-0.182195228018721,0.0206671890819858,
-0.930103735001198));
#85297=CARTESIAN_POINT('Ctrl Pts',(-0.116526144208468,-0.141599663971141,
-0.919019208243116));
#85298=CARTESIAN_POINT('Ctrl Pts',(0.0552978219715147,-0.174820013947988,
-0.907934681485038));
#85299=CARTESIAN_POINT('Ctrl Pts',(0.176745121098773,-0.0488296691835216,
-0.896850154726956));
#85300=CARTESIAN_POINT('Ctrl Pts',(0.137198045104627,0.121657099237068,
-0.885765627968878));
#85301=CARTESIAN_POINT('Ctrl Pts',(-0.027324548795888,0.181317083331244,
-0.874681101210796));
#85302=CARTESIAN_POINT('Ctrl Pts',(-0.166956328484408,0.0758198406289321,
-0.863596574452717));
#85303=CARTESIAN_POINT('Ctrl Pts',(-0.154507759153884,-0.0987443364908174,
-0.852512047694636));
#85304=CARTESIAN_POINT('Ctrl Pts',(-0.00131759116581058,-0.183360815188498,
-0.841427520936557));
#85305=CARTESIAN_POINT('Ctrl Pts',(0.153072651329834,-0.100954325685835,
-0.830342994178476));
#85306=CARTESIAN_POINT('Ctrl Pts',(0.168028832178233,0.0734119869196514,
-0.819258467420397));
#85307=CARTESIAN_POINT('Ctrl Pts',(0.0299272448487212,0.180907010513025,
-0.808173940662315));
#85308=CARTESIAN_POINT('Ctrl Pts',(-0.13543510058501,0.123613646523463,
-0.797089413904237));
#85309=CARTESIAN_POINT('Ctrl Pts',(-0.177429403316478,-0.0462796406044383,
-0.786004887146155));
#85310=CARTESIAN_POINT('Ctrl Pts',(-0.0578029710631441,-0.174016700605967,
-0.774920360388076));
#85311=CARTESIAN_POINT('Ctrl Pts',(0.114476278373398,-0.1432416814435,-0.763835833629995));
#85312=CARTESIAN_POINT('Ctrl Pts',(0.182478902227141,0.0180124244145374,
-0.752751306871914));
#85313=CARTESIAN_POINT('Ctrl Pts',(0.0842611985256882,0.162858979757378,
-0.741666780113836));
#85314=CARTESIAN_POINT('Ctrl Pts',(-0.0907101666775044,0.15935702943093,
-0.730582253355755));
#85315=CARTESIAN_POINT('Ctrl Pts',(-0.183053494695443,0.0106965024300354,
-0.719497726597676));
#85316=CARTESIAN_POINT('Ctrl Pts',(-0.108653098550686,-0.147707485334438,
-0.708413199839595));
#85317=CARTESIAN_POINT('Ctrl Pts',(0.0647195805515337,-0.171564486375374,
-0.697328673081514));
#85318=CARTESIAN_POINT('Ctrl Pts',(0.179139089195798,-0.0391431194354451,
-0.686244146323435));
#85319=CARTESIAN_POINT('Ctrl Pts',(0.130380512058046,0.128933778154068,
-0.675159619565355));
#85320=CARTESIAN_POINT('Ctrl Pts',(-0.0371418841496764,0.179564688960573,
-0.664075092807276));
#85321=CARTESIAN_POINT('Ctrl Pts',(-0.170831678082726,0.0666298344632292,
-0.652990566049193));
#85322=CARTESIAN_POINT('Ctrl Pts',(-0.148910620450773,-0.106998243882291,
-0.641906039291115));
#85323=CARTESIAN_POINT('Ctrl Pts',(0.00865336193011468,-0.18316144901443,
-0.630821512533036));
#85324=CARTESIAN_POINT('Ctrl Pts',(0.158334982948992,-0.0924825943185493,
-0.619736985774954));
#85325=CARTESIAN_POINT('Ctrl Pts',(0.163789012191789,0.08243880495611,-0.608652459016875));
#85326=CARTESIAN_POINT('Ctrl Pts',(0.0200473656101289,0.182266563608242,
-0.597567932258793));
#85327=CARTESIAN_POINT('Ctrl Pts',(-0.141955458694602,0.11606741499751,
-0.586483405500715));
#85328=CARTESIAN_POINT('Ctrl Pts',(-0.174650826329757,-0.0558577294538408,
-0.575398878742634));
#85329=CARTESIAN_POINT('Ctrl Pts',(-0.0482564740935901,-0.176901977901532,
-0.564314351984555));
#85330=CARTESIAN_POINT('Ctrl Pts',(0.122094778358068,-0.136805928874095,
-0.553229825226472));
#85331=CARTESIAN_POINT('Ctrl Pts',(0.181229699945847,0.0279068617897054,
-0.542145298468395));
#85332=CARTESIAN_POINT('Ctrl Pts',(0.0752821950564939,0.167199246962685,
-0.531060771710313));
#85333=CARTESIAN_POINT('Ctrl Pts',(-0.0992399829364661,0.154189567948618,
-0.519976244952235));
#85334=CARTESIAN_POINT('Ctrl Pts',(-0.183364300139518,0.000728362379997262,
-0.508891718194153));
#85335=CARTESIAN_POINT('Ctrl Pts',(-0.10046178010034,-0.153396309657315,
-0.497807191436073));
#85336=CARTESIAN_POINT('Ctrl Pts',(0.0739515377392648,-0.167792035399211,
-0.486722664677994));
#85337=CARTESIAN_POINT('Ctrl Pts',(0.181002280375352,-0.0293457250095247,
-0.475638137919914));
#85338=CARTESIAN_POINT('Ctrl Pts',(0.12317775338849,0.135831653702577,-0.464553611161834));
#85339=CARTESIAN_POINT('Ctrl Pts',(-0.0468495881671225,0.177279759606062,
-0.453469084403753));
#85340=CARTESIAN_POINT('Ctrl Pts',(-0.174201564170652,0.0572434460694844,
-0.442384557645674));
#85341=CARTESIAN_POINT('Ctrl Pts',(-0.142873053929396,-0.114936014974851,
-0.431300030887593));
#85342=CARTESIAN_POINT('Ctrl Pts',(0.0185987519632387,-0.182420074286859,
-0.420215504129514));
#85343=CARTESIAN_POINT('Ctrl Pts',(0.163128924644238,-0.0837373932113132,
-0.409130977371433));
#85344=CARTESIAN_POINT('Ctrl Pts',(0.159064696314123,0.0912218146273431,
-0.398046450613352));
#85345=CARTESIAN_POINT('Ctrl Pts',(0.0101081791250124,0.183086924143141,
-0.386961923855273));
#85346=CARTESIAN_POINT('Ctrl Pts',(-0.148055894759956,0.108177858659869,
-0.375877397097193));
#85347=CARTESIAN_POINT('Ctrl Pts',(-0.171355614907519,-0.0652705930497431,
-0.364792870339113));
#85348=CARTESIAN_POINT('Ctrl Pts',(-0.0385672285920655,-0.179263956098795,
-0.353708343581032));
#85349=CARTESIAN_POINT('Ctrl Pts',(0.129352108557561,-0.129965491916379,
-0.342623816822953));
#85350=CARTESIAN_POINT('Ctrl Pts',(0.179444401039445,0.0377187488252464,
-0.331539290064872));
#85351=CARTESIAN_POINT('Ctrl Pts',(0.066080498702647,0.17104492032495,-0.320454763306793));
#85352=CARTESIAN_POINT('Ctrl Pts',(-0.107476236663192,0.148565997555451,
-0.309370236548711));
#85353=CARTESIAN_POINT('Ctrl Pts',(-0.183132694411917,-0.009241932405554,
-0.298285709790633));
#85354=CARTESIAN_POINT('Ctrl Pts',(-0.0919732849516963,-0.158631371219217,
-0.287201183032551));
#85355=CARTESIAN_POINT('Ctrl Pts',(0.0829647383674402,-0.163523237679612,
-0.276116656274472));
#85356=CARTESIAN_POINT('Ctrl Pts',(0.182330047462404,-0.0194615227922904,
-0.265032129516391));
#85357=CARTESIAN_POINT('Ctrl Pts',(0.115610621762305,0.142327724733257,
-0.253947602758312));
#85358=CARTESIAN_POINT('Ctrl Pts',(-0.0564187061067814,0.174470417692299,
-0.242863076000231));
#85359=CARTESIAN_POINT('Ctrl Pts',(-0.177056143386771,0.0476877256057966,
-0.231778549242151));
#85360=CARTESIAN_POINT('Ctrl Pts',(-0.136412853689387,-0.12253379336342,
-0.220694022484071));
#85361=CARTESIAN_POINT('Ctrl Pts',(0.0284891249897688,-0.181139080879629,
-0.209609495725991));
#85362=CARTESIAN_POINT('Ctrl Pts',(0.167440313371968,-0.0747444890892225,
-0.198524968967911));
#85363=CARTESIAN_POINT('Ctrl Pts',(0.153869850388125,0.0997349826014979,
-0.187440442209831));
#85364=CARTESIAN_POINT('Ctrl Pts',(0.000139090944378808,0.183365689831066,
-0.176355915451751));
#85365=CARTESIAN_POINT('Ctrl Pts',(-0.153718364479581,0.0999683085654659,
-0.165271388693671));
#85366=CARTESIAN_POINT('Ctrl Pts',(-0.167553517512711,-0.0744903943231421,
-0.15418686193559));
#85367=CARTESIAN_POINT('Ctrl Pts',(-0.0287638928153855,-0.181095623655295,
-0.143102335177511));
#85368=CARTESIAN_POINT('Ctrl Pts',(0.136226793222509,-0.122740657791065,
-0.13201780841943));
#85369=CARTESIAN_POINT('Ctrl Pts',(0.177128301973759,0.0474191638445822,
-0.12093328166135));
#85370=CARTESIAN_POINT('Ctrl Pts',(0.0566832995374016,0.174384426330519,
-0.10984875490327));
#85371=CARTESIAN_POINT('Ctrl Pts',(-0.115394507761123,0.142503330509622,
-0.0987642281451906));
#85372=CARTESIAN_POINT('Ctrl Pts',(-0.18235947006817,-0.0191856073775684,
-0.0876797013871106));
#85373=CARTESIAN_POINT('Ctrl Pts',(-0.0832125183308621,-0.163395815331006,
-0.0765951746290301));
#85374=CARTESIAN_POINT('Ctrl Pts',(0.0917321306689327,-0.158773327666352,
-0.0655106478709507));
#85375=CARTESIAN_POINT('Ctrl Pts',(0.183119205053686,-0.00951478666591987,
-0.05442612111287));
#85376=CARTESIAN_POINT('Ctrl Pts',(0.107700087856717,0.148393320157019,
-0.0433415943547902));
#85377=CARTESIAN_POINT('Ctrl Pts',(-0.065818238191846,0.171162982686544,
-0.03225706759671));
#85378=CARTESIAN_POINT('Ctrl Pts',(-0.179392109761845,0.0379566169796293,
-0.0211725408386302));
#85379=CARTESIAN_POINT('Ctrl Pts',(-0.129539265966577,-0.129703510329422,
-0.0100880140805498));
#85380=CARTESIAN_POINT('Ctrl Pts',(0.0382757593502112,-0.179449160753822,
0.000996512677530166));
#85381=CARTESIAN_POINT('Ctrl Pts',(0.171299276958504,-0.0652716633324161,
0.0120810394356104));
#85382=CARTESIAN_POINT('Ctrl Pts',(0.1558320429858,0.0497893031757065,0.019470723940997));
#85383=CARTESIAN_POINT('Ctrl Pts',(0.125514135451595,0.0914158484392161,
0.0231655661936903));
#85384=CARTESIAN_POINT('Ctrl Pts',(0.0210491062034705,-0.154371551634071,
-1.92554305833426E-15));
#85385=CARTESIAN_POINT('Ctrl Pts',(0.0249906761485533,-0.154347944482943,
-2.08179767172651E-15));
#85386=CARTESIAN_POINT('Ctrl Pts',(0.0289233405816073,-0.154164839339631,
-1.82232685243181E-15));
#85387=CARTESIAN_POINT('Ctrl Pts',(0.0328381830330719,-0.153819660683202,
-1.9671764217577E-15));
#85388=CARTESIAN_POINT('Ctrl Pts',(0.0417954224626671,-0.15302988487231,
-2.40177476828239E-15));
#85389=CARTESIAN_POINT('Ctrl Pts',(0.0506592073437473,-0.151393578924998,
-2.68040904842411E-15));
#85390=CARTESIAN_POINT('Ctrl Pts',(0.0593543406709811,-0.148991873564261,
-2.49106291150269E-15));
#85391=CARTESIAN_POINT('Ctrl Pts',(0.0641334869885079,-0.147671813146716,
-2.21133230102988E-15));
#85392=CARTESIAN_POINT('Ctrl Pts',(0.0688565095039308,-0.14612102978709,
-2.56627996653982E-15));
#85393=CARTESIAN_POINT('Ctrl Pts',(0.0734977242378156,-0.144357781793704,
-2.47024622979097E-15));
#85394=CARTESIAN_POINT('Ctrl Pts',(0.0812645483498012,-0.14140708077777,
-2.30953891825472E-15));
#85395=CARTESIAN_POINT('Ctrl Pts',(0.0888125783363352,-0.137859846860542,
-1.52387926237079E-15));
#85396=CARTESIAN_POINT('Ctrl Pts',(0.0960882881071144,-0.133769590071901,
-2.19615992058664E-15));
#85397=CARTESIAN_POINT('Ctrl Pts',(0.100603799299556,-0.131231061063605,
-2.61339630470243E-15));
#85398=CARTESIAN_POINT('Ctrl Pts',(0.105012894248953,-0.128482986224302,
-2.24724647575841E-15));
#85399=CARTESIAN_POINT('Ctrl Pts',(0.109282262285862,-0.125551551600707,
-2.11289319373975E-15));
#85400=CARTESIAN_POINT('Ctrl Pts',(0.118929558089528,-0.118927522775262,
-1.80930122354136E-15));
#85401=CARTESIAN_POINT('Ctrl Pts',(0.127886007007196,-0.111360115256469,
-1.91826500988144E-15));
#85402=CARTESIAN_POINT('Ctrl Pts',(0.136001978678605,-0.102988394911393,
-1.38604405730547E-15));
#85403=CARTESIAN_POINT('Ctrl Pts',(0.14010066837913,-0.0987605482230019,
-1.11726434428458E-15));
#85404=CARTESIAN_POINT('Ctrl Pts',(0.14398482089894,-0.0943267422381278,
-9.21274069104527E-16));
#85405=CARTESIAN_POINT('Ctrl Pts',(0.147632822555182,-0.0897004696527729,
-5.95010152260045E-16));
#85406=CARTESIAN_POINT('Ctrl Pts',(0.150543464665863,-0.0860092915582159,
-3.34692974514596E-16));
#85407=CARTESIAN_POINT('Ctrl Pts',(0.153301209336262,-0.082197730922776,
-8.41928195914956E-17));
#85408=CARTESIAN_POINT('Ctrl Pts',(0.155883789306881,-0.0782916799561493,
-1.09287578986539E-16));
#85409=CARTESIAN_POINT('Ctrl Pts',(0.159148499358082,-0.0733539339826171,
-1.41010551425541E-16));
#85410=CARTESIAN_POINT('Ctrl Pts',(0.162139340594116,-0.0682579463034665,
3.42436685437861E-16));
#85411=CARTESIAN_POINT('Ctrl Pts',(0.164837347197669,-0.063020026556347,
5.91540705308091E-16));
#85412=CARTESIAN_POINT('Ctrl Pts',(0.168353236127199,-0.0561942671129082,
8.97277816030434E-16));
#85413=CARTESIAN_POINT('Ctrl Pts',(0.171372272563736,-0.0491276521825463,
1.12084903965696E-15));
#85414=CARTESIAN_POINT('Ctrl Pts',(0.173907391890521,-0.0418709293396242,
1.60461921527855E-15));
#85415=CARTESIAN_POINT('Ctrl Pts',(0.175675656440153,-0.0368093112871495,
1.40713357097467E-15));
#85416=CARTESIAN_POINT('Ctrl Pts',(0.177208643735401,-0.0316537207737417,
1.59324788500904E-15));
#85417=CARTESIAN_POINT('Ctrl Pts',(0.178507313524868,-0.0264241089443225,
1.66533453693773E-15));
#85418=CARTESIAN_POINT('Ctrl Pts',(0.179596733069877,-0.0220371266752443,
1.72580611191571E-15));
#85419=CARTESIAN_POINT('Ctrl Pts',(0.180519059980037,-0.0176060950243616,
1.88764134780047E-15));
#85420=CARTESIAN_POINT('Ctrl Pts',(0.181275612730176,-0.0131509784388465,
1.85268467234323E-15));
#85421=CARTESIAN_POINT('Ctrl Pts',(0.183123733832993,-0.00226793693819612,
1.76729185659452E-15));
#85422=CARTESIAN_POINT('Ctrl Pts',(0.183989435438147,0.00877647129111679,
1.46112760885068E-15));
#85423=CARTESIAN_POINT('Ctrl Pts',(0.183904136655522,0.0198423917610982,
1.51875040321769E-15));
#85424=CARTESIAN_POINT('Ctrl Pts',(0.18385525744904,0.0261835539079751,
1.5517702937391E-15));
#85425=CARTESIAN_POINT('Ctrl Pts',(0.183493534385419,0.0325320838244838,
7.45918507883439E-16));
#85426=CARTESIAN_POINT('Ctrl Pts',(0.182820145325716,0.0388632508128488,
7.19042880792387E-16));
#85427=CARTESIAN_POINT('Ctrl Pts',(0.182239131666724,0.0443259093526593,
6.95854047815544E-16));
#85428=CARTESIAN_POINT('Ctrl Pts',(0.181424826261944,0.0497778655432242,
9.96295625820296E-16));
#85429=CARTESIAN_POINT('Ctrl Pts',(0.180384702012361,0.055169520382088,
9.51062145704284E-16));
#85430=CARTESIAN_POINT('Ctrl Pts',(0.177958241768075,0.0677474754895241,
8.45538943782813E-16));
#85431=CARTESIAN_POINT('Ctrl Pts',(0.174303572517529,0.080038108209797,
4.0076412894154E-16));
#85432=CARTESIAN_POINT('Ctrl Pts',(0.169446063228336,0.0918430005340087,
-2.68231617472914E-16));
#85433=CARTESIAN_POINT('Ctrl Pts',(0.166164925312101,0.0998169389242502,
-7.20123148436007E-16));
#85434=CARTESIAN_POINT('Ctrl Pts',(0.162333929398081,0.107569631004673,
-1.26651752900455E-16));
#85435=CARTESIAN_POINT('Ctrl Pts',(0.157947475570094,0.115038058750287,
1.30104260698261E-18));
#85436=CARTESIAN_POINT('Ctrl Pts',(0.089187861459517,0.173858233536057,
-0.9746));
#85437=CARTESIAN_POINT('Ctrl Pts',(0.0882329452274535,0.174454830838509,
-0.9746));
#85438=CARTESIAN_POINT('Ctrl Pts',(0.08727802899539,0.175051428140961,-0.9746));
#85439=CARTESIAN_POINT('Ctrl Pts',(0.0863231127633264,0.175648025443413,
-0.9746));
#85440=CARTESIAN_POINT('Origin',(0.,0.,0.232200846792815));
#85441=CARTESIAN_POINT('',(0.125,-0.0422728431058792,0.201303634366138));
#85442=CARTESIAN_POINT('',(0.125,0.0422728431058792,0.201303634366138));
#85443=CARTESIAN_POINT('Ctrl Pts',(0.125,-0.0422728431058792,0.201303634366138));
#85444=CARTESIAN_POINT('Ctrl Pts',(0.125,2.15105711021124E-16,0.193484871477951));
#85445=CARTESIAN_POINT('Ctrl Pts',(0.125,0.0422728431058792,0.201303634366138));
#85446=CARTESIAN_POINT('Origin',(0.,0.,0.201303634366138));
#85447=CARTESIAN_POINT('Origin',(0.,0.,0.232200846792815));
#85448=CARTESIAN_POINT('',(0.0258906439801145,-0.129389597025995,0.201303634366138));
#85449=CARTESIAN_POINT('',(0.0991093560198853,-0.0871167539201152,0.201303634366137));
#85450=CARTESIAN_POINT('Ctrl Pts',(0.0258906439801145,-0.129389597025995,
0.201303634366138));
#85451=CARTESIAN_POINT('Ctrl Pts',(0.0625000000000001,-0.108253175473055,
0.19348487147795));
#85452=CARTESIAN_POINT('Ctrl Pts',(0.0991093560198853,-0.0871167539201152,
0.201303634366138));
#85453=CARTESIAN_POINT('Origin',(0.,0.,0.201303634366138));
#85454=CARTESIAN_POINT('Origin',(0.,0.,0.232200846792815));
#85455=CARTESIAN_POINT('',(0.0991093560198853,0.0871167539201153,0.201303634366138));
#85456=CARTESIAN_POINT('',(0.0258906439801146,0.129389597025995,0.201303634366138));
#85457=CARTESIAN_POINT('Ctrl Pts',(0.0991093560198853,0.0871167539201153,
0.201303634366138));
#85458=CARTESIAN_POINT('Ctrl Pts',(0.0624999999999998,0.108253175473055,
0.193484871477951));
#85459=CARTESIAN_POINT('Ctrl Pts',(0.0258906439801146,0.129389597025995,
0.201303634366138));
#85460=CARTESIAN_POINT('Origin',(0.,0.,0.201303634366138));
#85461=CARTESIAN_POINT('Origin',(0.,0.,0.232200846792815));
#85462=CARTESIAN_POINT('',(-0.0258906439801146,0.129389597025995,0.201303634366138));
#85463=CARTESIAN_POINT('',(-0.0991093560198852,0.0871167539201153,0.201303634366138));
#85464=CARTESIAN_POINT('Ctrl Pts',(-0.0258906439801146,0.129389597025995,
0.201303634366138));
#85465=CARTESIAN_POINT('Ctrl Pts',(-0.0625000000000002,0.108253175473055,
0.19348487147795));
#85466=CARTESIAN_POINT('Ctrl Pts',(-0.0991093560198852,0.0871167539201153,
0.201303634366137));
#85467=CARTESIAN_POINT('Origin',(0.,0.,0.201303634366138));
#85468=CARTESIAN_POINT('Origin',(0.,0.,0.232200846792815));
#85469=CARTESIAN_POINT('',(-0.125,0.0422728431058793,0.201303634366137));
#85470=CARTESIAN_POINT('',(-0.125,-0.0422728431058794,0.201303634366138));
#85471=CARTESIAN_POINT('Ctrl Pts',(-0.125,0.0422728431058793,0.201303634366137));
#85472=CARTESIAN_POINT('Ctrl Pts',(-0.125,-2.98372437868011E-16,0.19348487147795));
#85473=CARTESIAN_POINT('Ctrl Pts',(-0.125,-0.0422728431058794,0.201303634366137));
#85474=CARTESIAN_POINT('',(-0.131954512102672,-1.61597670879588E-17,0.201303634366138));
#85475=CARTESIAN_POINT('Origin',(0.,0.,0.201303634366138));
#85476=CARTESIAN_POINT('Origin',(0.,0.,0.201303634366138));
#85477=CARTESIAN_POINT('Origin',(0.,0.,0.232200846792815));
#85478=CARTESIAN_POINT('',(-0.0991093560198854,-0.0871167539201152,0.201303634366138));
#85479=CARTESIAN_POINT('',(-0.0258906439801146,-0.129389597025995,0.201303634366138));
#85480=CARTESIAN_POINT('Ctrl Pts',(-0.0991093560198854,-0.0871167539201152,
0.201303634366138));
#85481=CARTESIAN_POINT('Ctrl Pts',(-0.0624999999999998,-0.108253175473055,
0.19348487147795));
#85482=CARTESIAN_POINT('Ctrl Pts',(-0.0258906439801146,-0.129389597025995,
0.201303634366138));
#85483=CARTESIAN_POINT('Origin',(0.,0.,0.201303634366138));
#85484=CARTESIAN_POINT('Origin',(5.55111512312578E-17,0.,-0.255));
#85485=CARTESIAN_POINT('',(-0.38,-4.65365783675994E-17,0.03));
#85486=CARTESIAN_POINT('Origin',(5.55111512312578E-17,0.,-0.255));
#85487=CARTESIAN_POINT('Origin',(0.,0.,0.03));
#85488=CARTESIAN_POINT('',(-0.125,0.0721687836487032,0.197539132746182));
#85489=CARTESIAN_POINT('Origin',(-0.125,-2.40370335797946E-17,-0.255));
#85490=CARTESIAN_POINT('Origin',(-0.0625,0.108253175473055,-0.255));
#85491=CARTESIAN_POINT('',(8.83812698937422E-18,0.144337567297406,0.197539132746182));
#85492=CARTESIAN_POINT('Origin',(-0.0625,0.108253175473055,-0.255));
#85493=CARTESIAN_POINT('Origin',(0.0625000000000001,0.108253175473055,-0.255));
#85494=CARTESIAN_POINT('',(0.125,0.0721687836487032,0.197539132746182));
#85495=CARTESIAN_POINT('Origin',(0.0625000000000001,0.108253175473055,-0.255));
#85496=CARTESIAN_POINT('Origin',(0.125,-4.80740671595891E-17,-0.255));
#85497=CARTESIAN_POINT('',(0.125,-0.0721687836487033,0.197539132746182));
#85498=CARTESIAN_POINT('Origin',(0.125,-4.80740671595891E-17,-0.255));
#85499=CARTESIAN_POINT('Origin',(0.0625,-0.108253175473055,-0.255));
#85500=CARTESIAN_POINT('',(-2.65143809681227E-17,-0.144337567297406,0.197539132746182));
#85501=CARTESIAN_POINT('Origin',(0.0625,-0.108253175473055,-0.255));
#85502=CARTESIAN_POINT('Origin',(-0.0625,-0.108253175473055,-0.255));
#85503=CARTESIAN_POINT('',(-0.125,-0.0721687836487032,0.197539132746182));
#85504=CARTESIAN_POINT('Origin',(-0.0625,-0.108253175473055,-0.255));
#85505=CARTESIAN_POINT('Origin',(-0.125,-2.40370335797946E-17,-0.255));
#85506=CARTESIAN_POINT('Origin',(0.,0.,0.033697287084562));
#85507=CARTESIAN_POINT('',(0.,0.,-0.00360542583087612));
#85508=CARTESIAN_POINT('',(-0.120858028271594,1.48008397474068E-17,0.07));
#85509=CARTESIAN_POINT('',(-0.06125,-7.50096164477754E-18,0.033697287084562));
#85510=CARTESIAN_POINT('Origin',(0.,0.,0.07));
#85511=CARTESIAN_POINT('Origin',(-2.77555756156289E-17,-0.144337567297406,
0.22));
#85512=CARTESIAN_POINT('',(-2.77555756156289E-17,-0.144337567297406,0.07));
#85513=CARTESIAN_POINT('',(-2.65143809681227E-17,-0.144337567297406,0.22));
#85514=CARTESIAN_POINT('',(-0.125,-0.0721687836487032,0.07));
#85515=CARTESIAN_POINT('',(-0.125,-0.0721687836487032,0.07));
#85516=CARTESIAN_POINT('',(-0.125,-0.0721687836487032,0.22));
#85517=CARTESIAN_POINT('Origin',(-0.125,-0.0721687836487032,0.22));
#85518=CARTESIAN_POINT('',(-0.125,0.0721687836487032,0.07));
#85519=CARTESIAN_POINT('',(-0.125,0.0721687836487032,0.07));
#85520=CARTESIAN_POINT('',(-0.125,0.0721687836487032,0.22));
#85521=CARTESIAN_POINT('Origin',(-0.125,0.0721687836487032,0.22));
#85522=CARTESIAN_POINT('',(1.38777878078145E-17,0.144337567297406,0.07));
#85523=CARTESIAN_POINT('',(8.83812698937423E-18,0.144337567297406,0.07));
#85524=CARTESIAN_POINT('',(8.83812698937423E-18,0.144337567297406,0.22));
#85525=CARTESIAN_POINT('Origin',(0.,0.144337567297406,0.22));
#85526=CARTESIAN_POINT('',(0.125,0.0721687836487032,0.07));
#85527=CARTESIAN_POINT('',(0.125,0.0721687836487032,0.07));
#85528=CARTESIAN_POINT('',(0.125,0.0721687836487032,0.22));
#85529=CARTESIAN_POINT('Origin',(0.125,-0.0721687836487033,0.22));
#85530=CARTESIAN_POINT('',(0.125,-0.0721687836487033,0.07));
#85531=CARTESIAN_POINT('',(0.125,-0.0721687836487033,0.22));
#85532=CARTESIAN_POINT('',(-2.65143809681227E-17,-0.144337567297406,0.07));
#85533=CARTESIAN_POINT('Origin',(0.125,0.0721687836487032,0.22));
#85534=CARTESIAN_POINT('',(0.125,-0.0721687836487033,0.07));
#85535=CARTESIAN_POINT('Origin',(0.,0.,0.07));
#85536=CARTESIAN_POINT('Origin',(0.17,0.,-1.));
#85537=CARTESIAN_POINT('',(-0.17,-2.0818995585505E-17,-1.));
#85538=CARTESIAN_POINT('Origin',(0.,0.,-1.));
#85539=CARTESIAN_POINT('Origin',(0.,0.,-0.985));
#85540=CARTESIAN_POINT('',(-0.185,-2.2655965784226E-17,-0.985));
#85541=CARTESIAN_POINT('Origin',(0.38,0.,0.));
#85542=CARTESIAN_POINT('',(-0.38,-4.65365783675994E-17,0.));
#85543=CARTESIAN_POINT('Origin',(0.,0.,0.));
#85544=CARTESIAN_POINT('Origin',(0.,0.,0.015));
#85545=CARTESIAN_POINT('',(-0.38,-4.65365783675994E-17,0.015));
#85766=UNCERTAINTY_MEASURE_WITH_UNIT(LENGTH_MEASURE(0.001),#85790,
'DISTANCE_ACCURACY_VALUE',
'Maximum model space distance between geometric entities at asserted c
onnectivities');
#85769=UNCERTAINTY_MEASURE_WITH_UNIT(LENGTH_MEASURE(0.001),#85790,
'DISTANCE_ACCURACY_VALUE',
'Maximum model space distance between geometric entities at asserted c
onnectivities');
#85786=(
GEOMETRIC_REPRESENTATION_CONTEXT(3)
GLOBAL_UNCERTAINTY_ASSIGNED_CONTEXT((#85766))
GLOBAL_UNIT_ASSIGNED_CONTEXT((#85790,#85792,#85793))
REPRESENTATION_CONTEXT('','3D')
);
#85789=(
GEOMETRIC_REPRESENTATION_CONTEXT(3)
GLOBAL_UNCERTAINTY_ASSIGNED_CONTEXT((#85769))
GLOBAL_UNIT_ASSIGNED_CONTEXT((#85790,#85792,#85793))
REPRESENTATION_CONTEXT('','3D')
);
#85790=(
LENGTH_UNIT()
NAMED_UNIT(*)
SI_UNIT(.CENTI.,.METRE.)
);
#85792=(
NAMED_UNIT(*)
PLANE_ANGLE_UNIT()
SI_UNIT($,.RADIAN.)
);
#85793=(
NAMED_UNIT(*)
SI_UNIT($,.STERADIAN.)
SOLID_ANGLE_UNIT()
);
#85810=SHAPE_DEFINITION_REPRESENTATION(#85829,#85878);
#85829=PRODUCT_DEFINITION_SHAPE('',$,#85898);
#85878=SHAPE_REPRESENTATION('',(#10788),#85786);
#85881=PRODUCT_DEFINITION_CONTEXT('part definition',#85940,'design');
#85898=PRODUCT_DEFINITION('ISO 7380 M4x10 Button Head',
'ISO 7380 M4x10 Button Head',#85917,#85881);
#85917=PRODUCT_DEFINITION_FORMATION('',$,#85958);
#85940=APPLICATION_CONTEXT(
'Core Data for Automotive Mechanical Design Process');
#85941=PRODUCT_CONTEXT('part definition',#85940,'mechanical');
#85958=PRODUCT('ISO 7380 M4x10 Button Head',
'ISO 7380 M4x10 Button Head',$,(#85941));
#85977=PRESENTATION_STYLE_ASSIGNMENT((#85995));
#85995=SURFACE_STYLE_USAGE(.BOTH.,#86013);
#86013=SURFACE_SIDE_STYLE('',(#86031));
#86031=SURFACE_STYLE_FILL_AREA(#86049);
#86049=FILL_AREA_STYLE('Opaque(200,204,209)',(#86067));
#86067=FILL_AREA_STYLE_COLOUR('Opaque(200,204,209)',#86085);
#86085=COLOUR_RGB('Opaque(200,204,209)', 0.72549020, 0.75294118, 0.79215686);
ENDSEC;
END-ISO-10303-21;
